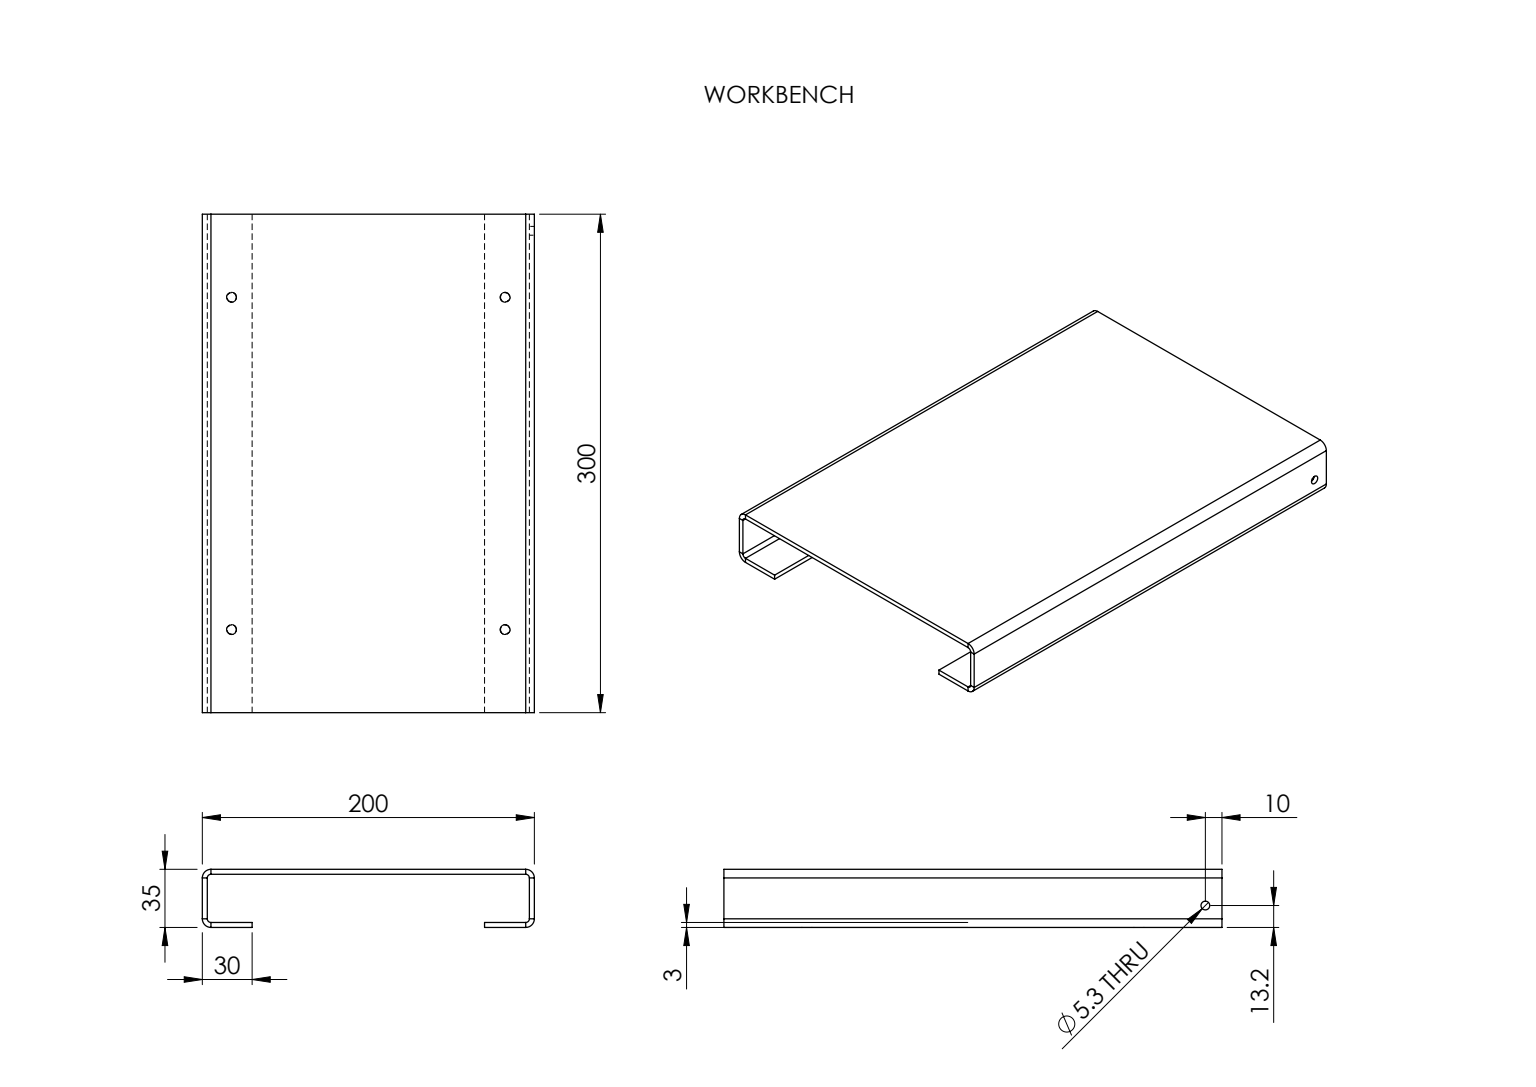
ISO-10303-21;
HEADER;
FILE_DESCRIPTION (('STEP AP214'),
    '1' );
FILE_NAME ('workbench.step',
    '2026-10-25T17:17:34',
    ( '' ),
    ( '' ),
    'SwSTEP 2.0',
    'SolidWorks 2026',
    '' );
FILE_SCHEMA (( 'AUTOMOTIVE_DESIGN' ));
ENDSEC;

DATA;
#2=CARTESIAN_POINT ( 'NONE',  ( 85.15643035625001289, -33.70312499938548711, 98.40857419181659793 ) ) ;
#3=CARTESIAN_POINT ( 'NONE',  ( 82.39999999999999147, -32.36250000000000426, -96.99999999999997158 ) ) ;
#5=CARTESIAN_POINT ( 'NONE',  ( 80.90000000000000568, -33.24374999877097281, -97.40192378864668399 ) ) ;
#8=ORIENTED_EDGE ( 'NONE', *, *, #12900, .F. ) ;
#13=ORIENTED_EDGE ( 'NONE', *, *, #6864, .F. ) ;
#14=VERTEX_POINT ( 'NONE', #6375 ) ;
#17=CARTESIAN_POINT ( 'NONE',  ( -85.40000000000000568, -32.23124999877096997, 98.26794919243111792 ) ) ;
#19=CARTESIAN_POINT ( 'NONE',  ( -79.77811200999887831, -35.00000000000000000, 100.8506536761481414 ) ) ;
#20=CARTESIAN_POINT ( 'NONE',  ( 82.40000000000000568, -30.00000000000000355, -103.0000000000000000 ) ) ;
#21=CARTESIAN_POINT ( 'NONE',  ( -81.02178482187500208, -34.45312499938548711, 97.61286128772489690 ) ) ;
#29=EDGE_LOOP ( 'NONE', ( #8971, #4412, #15076, #17801 ) ) ;
#30=CARTESIAN_POINT ( 'NONE',  ( -85.15643035624999868, -34.22812499938547859, -101.5914258081833879 ) ) ;
#33=CARTESIAN_POINT ( 'NONE',  ( 80.07894310789828296, -34.99999999999997868, -101.4973817956044400 ) ) ;
#38=ORIENTED_EDGE ( 'NONE', *, *, #10348, .F. ) ;
#39=CARTESIAN_POINT ( 'NONE',  ( -84.28136653320154892, -32.00000000000001421, 97.98546077809197641 ) ) ;
#41=CARTESIAN_POINT ( 'NONE',  ( -85.40000000000000568, -32.60624999877097707, 101.7320508075688679 ) ) ;
#42=CARTESIAN_POINT ( 'NONE',  ( 82.39999999999999147, -32.36250000000000426, 103.4641016151377499 ) ) ;
#43=CARTESIAN_POINT ( 'NONE',  ( -80.80636817121818183, -32.00000000000000000, -97.53037344451308854 ) ) ;
#46=CARTESIAN_POINT ( 'NONE',  ( 82.39999999999999147, -33.62812499938549138, 96.81714838363319586 ) ) ;
#48=CARTESIAN_POINT ( 'NONE',  ( 85.15643035625001289, -30.59062499938548285, -99.99999999999998579 ) ) ;
#50=( BOUNDED_CURVE ( )  B_SPLINE_CURVE ( 2, ( #14072, #3327, #4905, #3619, #6463, #18477, #9481, #10851, #12417 ),
 .UNSPECIFIED., .F., .F. ) 
 B_SPLINE_CURVE_WITH_KNOTS ( ( 3, 2, 2, 2, 3 ),
 ( 0.6041666666666666297, 0.6111111111111111605, 0.6250000000000000000, 0.6388888888888888395, 0.6458333333333332593 ),
 .UNSPECIFIED. ) 
 CURVE ( )  GEOMETRIC_REPRESENTATION_ITEM ( )  RATIONAL_B_SPLINE_CURVE ( ( 0.9330127018922192983, 0.9330127018922187432, 1.000000000000000000, 0.8660254037844387076, 1.000000000000000000, 0.8660254037844387076, 1.000000000000000000, 0.9330127018922198534, 0.9330127018922192983 ) ) 
 REPRESENTATION_ITEM ( '' )  );
#53=CARTESIAN_POINT ( 'NONE',  ( 83.77821517812500929, -34.26562499938548711, -97.61286128772489690 ) ) ;
#55=CYLINDRICAL_SURFACE ( 'NONE', #7872, 3.000000000000002665 ) ;
#57=( BOUNDED_CURVE ( )  B_SPLINE_CURVE ( 2, ( #14794, #2683, #1229, #10402, #2880, #14892, #1421, #4162, #17640 ),
 .UNSPECIFIED., .F., .F. ) 
 B_SPLINE_CURVE_WITH_KNOTS ( ( 3, 2, 2, 2, 3 ),
 ( 0.6458333333333333703, 0.6527777777777777901, 0.6666666666666666297, 0.6805555555555555802, 0.6875000000000000000 ),
 .UNSPECIFIED. ) 
 CURVE ( )  GEOMETRIC_REPRESENTATION_ITEM ( )  RATIONAL_B_SPLINE_CURVE ( ( 0.9330127018922192983, 0.9330127018922198534, 1.000000000000000000, 0.8660254037844387076, 1.000000000000000000, 0.8660254037844387076, 1.000000000000000000, 0.9330127018922194093, 0.9330127018922194093 ) ) 
 REPRESENTATION_ITEM ( '' )  );
#58=CARTESIAN_POINT ( 'NONE',  ( -85.40000000000000568, -30.03750000000000497, 98.26794919243111792 ) ) ;
#60=CARTESIAN_POINT ( 'NONE',  ( -80.90000000000000568, -32.85000000000000142, 97.40192378864668399 ) ) ;
#64=EDGE_CURVE ( 'NONE', #2579, #12229, #9687, .T. ) ;
#65=LINE ( 'NONE', #3169, #11720 ) ;
#68=CARTESIAN_POINT ( 'NONE',  ( -79.39999999999999147, -32.47500000000000142, 99.99999999999998579 ) ) ;
#69=CARTESIAN_POINT ( 'NONE',  ( 83.77821517812500929, -32.57812499938548711, 102.3871387122750889 ) ) ;
#72=CARTESIAN_POINT ( 'NONE',  ( 85.15643035625001289, -30.25312499938548783, -99.99999999999998579 ) ) ;
#74=CARTESIAN_POINT ( 'NONE',  ( -83.77821517812500929, -32.87812499938548427, 102.3871387122750889 ) ) ;
#75=CARTESIAN_POINT ( 'NONE',  ( -85.15643035624999868, -30.29062499938548925, -101.5914258081833879 ) ) ;
#76=ORIENTED_EDGE ( 'NONE', *, *, #18961, .F. ) ;
#77=CARTESIAN_POINT ( 'NONE',  ( 85.40000000000000568, -35.34374999877096712, 99.99999999999998579 ) ) ;
#79=CARTESIAN_POINT ( 'NONE',  ( -82.40000000000000568, -30.00000000000000355, -96.99999999999998579 ) ) ;
#80=VECTOR ( 'NONE', #9829, 1000.000000000000000 ) ;
#81=CARTESIAN_POINT ( 'NONE',  ( -99.99999999999998579, -5.200000000000000178, 150.0000000000000000 ) ) ;
#83=CARTESIAN_POINT ( 'NONE',  ( -83.77821517812500929, -31.07812499938548711, 102.3871387122750889 ) ) ;
#84=( BOUNDED_CURVE ( )  B_SPLINE_CURVE ( 2, ( #13183, #17688, #10354, #13091, #8980, #17790, #14840, #19061, #2929 ),
 .UNSPECIFIED., .F., .F. ) 
 B_SPLINE_CURVE_WITH_KNOTS ( ( 3, 2, 2, 2, 3 ),
 ( 0.7708333333333332593, 0.7777777777777777901, 0.7916666666666666297, 0.8055555555555555802, 0.8125000000000000000 ),
 .UNSPECIFIED. ) 
 CURVE ( )  GEOMETRIC_REPRESENTATION_ITEM ( )  RATIONAL_B_SPLINE_CURVE ( ( 0.9330127018922192983, 0.9330127018922187432, 1.000000000000000000, 0.8660254037844387076, 1.000000000000000000, 0.8660254037844387076, 1.000000000000000000, 0.9330127018922194093, 0.9330127018922194093 ) ) 
 REPRESENTATION_ITEM ( '' )  );
#85=CARTESIAN_POINT ( 'NONE',  ( 82.61711639273572416, -31.99999999999999289, 102.8399189874672857 ) ) ;
#87=CARTESIAN_POINT ( 'NONE',  ( -83.90000000000000568, -30.82500000000000284, -97.40192378864668399 ) ) ;
#90=CARTESIAN_POINT ( 'NONE',  ( -85.15643035625001289, -32.95312499938548711, -99.99999999999998579 ) ) ;
#91=CARTESIAN_POINT ( 'NONE',  ( -82.14831453747900980, -32.00000000000000711, -102.8584433575392438 ) ) ;
#97=CARTESIAN_POINT ( 'NONE',  ( 83.77821517812500929, -33.66562499938548569, 97.61286128772489690 ) ) ;
#98=CARTESIAN_POINT ( 'NONE',  ( 80.90000000000000568, -32.40000000000000568, -97.40192378864668399 ) ) ;
#99=AXIS2_PLACEMENT_3D ( 'NONE', #13083, #5582, #10259 ) ;
#102=CARTESIAN_POINT ( 'NONE',  ( 83.90000000000000568, -35.26874999877097139, -102.5980762113533018 ) ) ;
#110=ORIENTED_EDGE ( 'NONE', *, *, #1169, .T. ) ;
#113=CARTESIAN_POINT ( 'NONE',  ( -81.90908125319960220, -32.00000000000000711, 97.16185054498753004 ) ) ;
#116=CARTESIAN_POINT ( 'NONE',  ( -79.39999999999999147, -34.76250000000000284, 101.7320508075688537 ) ) ;
#118=CARTESIAN_POINT ( 'NONE',  ( 69.99999999999998579, -31.99999999999998579, 150.0000000000000000 ) ) ;
#120=CARTESIAN_POINT ( 'NONE',  ( -85.15643035624999868, -33.44062499938548427, 98.40857419181659793 ) ) ;
#124=( BOUNDED_SURFACE ( )  B_SPLINE_SURFACE ( 1, 2, ( 
 ( #72, #18045, #10508, #17940, #4551, #3080, #4656, #1713, #12454, #13815, #2197, #651, #7770, #5135, #16858, #3463, #457, #16755, #7864, #15189, #8158, #2001, #1806, #6406, #9522, #9323, #14107, #17050, #9225, #11080, #551, #3563, #9626, #9421, #3371, #6508, #18420, #5041, #15389, #15287, #4754, #4848, #1902, #10982, #8060, #13913, #2100, #4947, #3269, #18518, #15588, #14015, #6599, #13723, #10793, #6699, #18329, #3661, #12361, #10890, #7958, #744, #364, #6313, #18135, #12266, #16951, #15487, #12547, #18231, #10698, #16664, #18617, #11277, #3951, #5339, #19004, #9815, #8536, #840, #5526, #6893, #1218, #6984, #14302, #2574, #12935, #5624, #16064, #14392, #1117, #18907, #15777, #18717, #3852, #17245, #2386, #12643, #12749, #8348, #11474, #4052, #15878, #938, #17441, #15685, #4148, #5235, #6803, #12843, #2482, #11183, #8440, #8253, #14486, #9719, #10011, #18812, #2669, #7077, #2289, #11570, #11375, #17341, #5436, #9916, #1031, #14203, #8629, #15969, #13033, #17533, #10108, #14587, #17147 ),
 ( #3754, #18022, #5908, #5808, #8918, #14880, #1509, #17822, #17733, #13124, #13221, #4340, #48, #16450, #2963, #10487, #13318, #11665, #7554, #4636, #3060, #9022, #16165, #19193, #15075, #7362, #148, #11759, #19295, #10301, #13511, #17628, #2776, #6099, #10201, #10391, #7459, #13419, #1318, #4243, #8729, #19094, #16260, #4433, #2870, #12047, #8827, #14981, #14683, #6000, #1409, #7174, #11950, #14784, #1605, #17920, #10586, #16551, #4529, #3150, #9113, #11854, #16352, #5715, #7266, #7751, #9602, #1786, #6293, #530, #12435, #4925, #16736, #15366, #4730, #12527, #7646, #15169, #15268, #10870, #13706, #6483, #3544, #1982, #15468, #346, #18116, #1883, #2078, #8035, #1694, #6581, #13601, #18403, #11059, #13992, #12244, #18211, #10964, #7940, #10772, #12341, #631, #3346, #5023, #4831, #18500, #9306, #10675, #440, #16841, #16644, #3447, #13891, #9500, #7842, #3640, #3246, #16934, #5119, #13797, #6385, #18305, #17030, #9402, #242, #6201, #12148, #9204, #17221, #8136, #18982, #17420, #4123, #2271 ) ),
 .UNSPECIFIED., .F., .F., .F. ) 
 B_SPLINE_SURFACE_WITH_KNOTS ( ( 2, 2 ),
 ( 3, 2, 2, 2, 2, 2, 2, 2, 2, 2, 2, 2, 2, 2, 2, 2, 2, 2, 2, 2, 2, 2, 2, 2, 2, 2, 2, 2, 2, 2, 2, 2, 2, 2, 2, 2, 2, 2, 2, 2, 2, 2, 2, 2, 2, 2, 2, 2, 2, 2, 2, 2, 2, 2, 2, 2, 2, 2, 2, 2, 2, 2, 2, 2, 2, 2, 2, 3 ),
 ( 0.000000000000000000, 1.000000000000000000 ),
 ( 0.000000000000000000, 0.01388888888888888812, 0.02777777777777777624, 0.04166666666666666435, 0.05555555555555555247, 0.06944444444444444753, 0.08333333333333332871, 0.09722222222222222376, 0.1111111111111111049, 0.1250000000000000000, 0.1388888888888888951, 0.1527777777777777901, 0.1666666666666666574, 0.1805555555555555525, 0.1944444444444444475, 0.2083333333333333426, 0.2222222222222222099, 0.2361111111111111049, 0.2500000000000000000, 0.2638888888888888951, 0.2777777777777777901, 0.2916666666666666852, 0.3055555555555555802, 0.3194444444444444198, 0.3333333333333333148, 0.3472222222222222099, 0.3611111111111111049, 0.3750000000000000000, 0.3888888888888888951, 0.4027777777777777901, 0.4166666666666666852, 0.4305555555555555802, 0.4444444444444444198, 0.4583333333333333148, 0.4722222222222222099, 0.4861111111111111049, 0.5000000000000000000, 0.5138888888888888395, 0.5277777777777777901, 0.5416666666666666297, 0.5555555555555555802, 0.5694444444444444198, 0.5833333333333333703, 0.5972222222222222099, 0.6111111111111111605, 0.6250000000000000000, 0.6388888888888888395, 0.6527777777777777901, 0.6666666666666666297, 0.6805555555555555802, 0.6944444444444444198, 0.7083333333333333703, 0.7222222222222222099, 0.7361111111111111605, 0.7500000000000000000, 0.7638888888888888395, 0.7777777777777777901, 0.7916666666666666297, 0.8055555555555555802, 0.8194444444444444198, 0.8333333333333333703, 0.8472222222222222099, 0.8611111111111111605, 0.8750000000000000000, 0.8888888888888888395, 0.9027777777777777901, 0.9166666666666666297, 0.9258785565094813652 ),
 .UNSPECIFIED. ) 
 GEOMETRIC_REPRESENTATION_ITEM ( )  RATIONAL_B_SPLINE_SURFACE ( (
 ( 1.000000000000000000, 0.8660254037844387076, 1.000000000000000000, 0.8660254037844387076, 1.000000000000000000, 0.8660254037844387076, 1.000000000000000000, 0.8660254037844387076, 1.000000000000000000, 0.8660254037844387076, 1.000000000000000000, 0.8660254037844387076, 1.000000000000000000, 0.8660254037844387076, 1.000000000000000000, 0.8660254037844387076, 1.000000000000000000, 0.8660254037844387076, 1.000000000000000000, 0.8660254037844387076, 1.000000000000000000, 0.8660254037844387076, 1.000000000000000000, 0.8660254037844387076, 1.000000000000000000, 0.8660254037844387076, 1.000000000000000000, 0.8660254037844387076, 1.000000000000000000, 0.8660254037844387076, 1.000000000000000000, 0.8660254037844387076, 1.000000000000000000, 0.8660254037844387076, 1.000000000000000000, 0.8660254037844387076, 1.000000000000000000, 0.8660254037844387076, 1.000000000000000000, 0.8660254037844387076, 1.000000000000000000, 0.8660254037844387076, 1.000000000000000000, 0.8660254037844387076, 1.000000000000000000, 0.8660254037844387076, 1.000000000000000000, 0.8660254037844387076, 1.000000000000000000, 0.8660254037844387076, 1.000000000000000000, 0.8660254037844387076, 1.000000000000000000, 0.8660254037844387076, 1.000000000000000000, 0.8660254037844387076, 1.000000000000000000, 0.8660254037844387076, 1.000000000000000000, 0.8660254037844387076, 1.000000000000000000, 0.8660254037844387076, 1.000000000000000000, 0.8660254037844387076, 1.000000000000000000, 0.8660254037844387076, 1.000000000000000000, 0.8660254037844387076, 1.000000000000000000, 0.8660254037844387076, 1.000000000000000000, 0.8660254037844387076, 1.000000000000000000, 0.8660254037844387076, 1.000000000000000000, 0.8660254037844387076, 1.000000000000000000, 0.8660254037844387076, 1.000000000000000000, 0.8660254037844387076, 1.000000000000000000, 0.8660254037844387076, 1.000000000000000000, 0.8660254037844387076, 1.000000000000000000, 0.8660254037844387076, 1.000000000000000000, 0.8660254037844387076, 1.000000000000000000, 0.8660254037844387076, 1.000000000000000000, 0.8660254037844387076, 1.000000000000000000, 0.8660254037844387076, 1.000000000000000000, 0.8660254037844387076, 1.000000000000000000, 0.8660254037844387076, 1.000000000000000000, 0.8660254037844387076, 1.000000000000000000, 0.8660254037844387076, 1.000000000000000000, 0.8660254037844387076, 1.000000000000000000, 0.8660254037844387076, 1.000000000000000000, 0.8660254037844387076, 1.000000000000000000, 0.8660254037844387076, 1.000000000000000000, 0.8660254037844387076, 1.000000000000000000, 0.8660254037844387076, 1.000000000000000000, 0.8660254037844387076, 1.000000000000000000, 0.8660254037844387076, 1.000000000000000000, 0.8660254037844387076, 1.000000000000000000, 0.8660254037844387076, 1.000000000000000000, 0.8660254037844387076, 1.000000000000000000, 0.8660254037844387076, 1.000000000000000000, 0.8660254037844387076, 1.000000000000000000, 0.8660254037844387076, 1.000000000000000000, 0.8660254037844387076, 1.000000000000000000, 0.9111405360107203144, 0.9401542295229963209),
 ( 1.000000000000000000, 0.8660254037844387076, 1.000000000000000000, 0.8660254037844387076, 1.000000000000000000, 0.8660254037844387076, 1.000000000000000000, 0.8660254037844387076, 1.000000000000000000, 0.8660254037844387076, 1.000000000000000000, 0.8660254037844387076, 1.000000000000000000, 0.8660254037844387076, 1.000000000000000000, 0.8660254037844387076, 1.000000000000000000, 0.8660254037844387076, 1.000000000000000000, 0.8660254037844387076, 1.000000000000000000, 0.8660254037844387076, 1.000000000000000000, 0.8660254037844387076, 1.000000000000000000, 0.8660254037844387076, 1.000000000000000000, 0.8660254037844387076, 1.000000000000000000, 0.8660254037844387076, 1.000000000000000000, 0.8660254037844387076, 1.000000000000000000, 0.8660254037844387076, 1.000000000000000000, 0.8660254037844387076, 1.000000000000000000, 0.8660254037844387076, 1.000000000000000000, 0.8660254037844387076, 1.000000000000000000, 0.8660254037844387076, 1.000000000000000000, 0.8660254037844387076, 1.000000000000000000, 0.8660254037844387076, 1.000000000000000000, 0.8660254037844387076, 1.000000000000000000, 0.8660254037844387076, 1.000000000000000000, 0.8660254037844387076, 1.000000000000000000, 0.8660254037844387076, 1.000000000000000000, 0.8660254037844387076, 1.000000000000000000, 0.8660254037844387076, 1.000000000000000000, 0.8660254037844387076, 1.000000000000000000, 0.8660254037844387076, 1.000000000000000000, 0.8660254037844387076, 1.000000000000000000, 0.8660254037844387076, 1.000000000000000000, 0.8660254037844387076, 1.000000000000000000, 0.8660254037844387076, 1.000000000000000000, 0.8660254037844387076, 1.000000000000000000, 0.8660254037844387076, 1.000000000000000000, 0.8660254037844387076, 1.000000000000000000, 0.8660254037844387076, 1.000000000000000000, 0.8660254037844387076, 1.000000000000000000, 0.8660254037844387076, 1.000000000000000000, 0.8660254037844387076, 1.000000000000000000, 0.8660254037844387076, 1.000000000000000000, 0.8660254037844387076, 1.000000000000000000, 0.8660254037844387076, 1.000000000000000000, 0.8660254037844387076, 1.000000000000000000, 0.8660254037844387076, 1.000000000000000000, 0.8660254037844387076, 1.000000000000000000, 0.8660254037844387076, 1.000000000000000000, 0.8660254037844387076, 1.000000000000000000, 0.8660254037844387076, 1.000000000000000000, 0.8660254037844387076, 1.000000000000000000, 0.8660254037844387076, 1.000000000000000000, 0.8660254037844387076, 1.000000000000000000, 0.8660254037844387076, 1.000000000000000000, 0.8660254037844387076, 1.000000000000000000, 0.8660254037844387076, 1.000000000000000000, 0.8660254037844387076, 1.000000000000000000, 0.8660254037844387076, 1.000000000000000000, 0.8660254037844387076, 1.000000000000000000, 0.8660254037844387076, 1.000000000000000000, 0.8660254037844387076, 1.000000000000000000, 0.8660254037844387076, 1.000000000000000000, 0.8660254037844387076, 1.000000000000000000, 0.8660254037844387076, 1.000000000000000000, 0.8660254037844387076, 1.000000000000000000, 0.9111405360107203144, 0.9401542295229963209) ) ) 
 REPRESENTATION_ITEM ( '' )  SURFACE ( )  );
#126=CARTESIAN_POINT ( 'NONE',  ( -80.90000000000000568, -33.45000000000000284, 102.5980762113533018 ) ) ;
#127=CARTESIAN_POINT ( 'NONE',  ( -79.39999999999999147, -34.70624999877097139, -98.26794919243113213 ) ) ;
#131=CARTESIAN_POINT ( 'NONE',  ( -79.64356964374999848, -33.51562499938548711, -99.99999999999998579 ) ) ;
#134=CARTESIAN_POINT ( 'NONE',  ( 81.96801452314025482, -35.00000000000000000, -102.7281823352556671 ) ) ;
#139=EDGE_LOOP ( 'NONE', ( #12823, #17187, #7892, #9526 ) ) ;
#142=CARTESIAN_POINT ( 'NONE',  ( -79.39999999999999147, -32.90624999877096712, 101.7320508075688537 ) ) ;
#143=CARTESIAN_POINT ( 'NONE',  ( 80.90000000000000568, -31.50000000000000000, 102.5980762113533018 ) ) ;
#146=CARTESIAN_POINT ( 'NONE',  ( 83.90000000000000568, -32.11874999877097281, 97.40192378864668399 ) ) ;
#147=CARTESIAN_POINT ( 'NONE',  ( 79.39999999999999147, -33.33749999999999858, -98.26794919243110371 ) ) ;
#148=CARTESIAN_POINT ( 'NONE',  ( 83.77821517812500929, -31.11562499938548498, -97.61286128772489690 ) ) ;
#151=CARTESIAN_POINT ( 'NONE',  ( 82.40000000000000568, -34.10624999877096997, 102.9999999999999858 ) ) ;
#152=CARTESIAN_POINT ( 'NONE',  ( 79.64356964375001269, -34.37812499938548427, -98.40857419181659793 ) ) ;
#154=CARTESIAN_POINT ( 'NONE',  ( -81.59615242270662350, -34.76115380933863719, 103.0000000000000000 ) ) ;
#156=CARTESIAN_POINT ( 'NONE',  ( -79.39999999999999147, -31.08750000000000213, 98.26794919243110371 ) ) ;
#157=ORIENTED_EDGE ( 'NONE', *, *, #9586, .F. ) ;
#163=DIRECTION ( 'NONE',  ( 1.000000000000000000, 0.000000000000000000, 0.000000000000000000 ) ) ;
#164=CARTESIAN_POINT ( 'NONE',  ( -82.40000000000000568, -32.30624999877097281, 97.00000000000000000 ) ) ;
#166=CARTESIAN_POINT ( 'NONE',  ( 81.02178482187500208, -34.90312499938548285, 102.3871387122750889 ) ) ;
#169=CARTESIAN_POINT ( 'NONE',  ( -83.77821517812500929, -32.42812499938548854, 102.3871387122750889 ) ) ;
#170=CARTESIAN_POINT ( 'NONE',  ( -81.02178482187500208, -30.55312499938548854, -97.61286128772489690 ) ) ;
#171=( BOUNDED_CURVE ( )  B_SPLINE_CURVE ( 2, ( #17183, #11218, #2322, #15621, #3787, #16002, #5563, #9753, #17473 ),
 .UNSPECIFIED., .F., .F. ) 
 B_SPLINE_CURVE_WITH_KNOTS ( ( 3, 2, 2, 2, 3 ),
 ( 0.7291666666666668517, 0.7361111111111111605, 0.7500000000000000000, 0.7638888888888888395, 0.7708333333333332593 ),
 .UNSPECIFIED. ) 
 CURVE ( )  GEOMETRIC_REPRESENTATION_ITEM ( )  RATIONAL_B_SPLINE_CURVE ( ( 0.9330127018922194093, 0.9330127018922209636, 1.000000000000000000, 0.8660254037844387076, 1.000000000000000000, 0.8660254037844387076, 1.000000000000000000, 0.9330127018922198534, 0.9330127018922192983 ) ) 
 REPRESENTATION_ITEM ( '' )  );
#173=CARTESIAN_POINT ( 'NONE',  ( 83.77821517812500929, -31.07812499938548711, 97.61286128772489690 ) ) ;
#174=CARTESIAN_POINT ( 'NONE',  ( -94.79999999999999716, -35.00000000000000000, 150.0000000000000000 ) ) ;
#176=VECTOR ( 'NONE', #9077, 1000.000000000000000 ) ;
#179=CARTESIAN_POINT ( 'NONE',  ( -81.02178482187500208, -31.30312499938548498, 97.61286128772489690 ) ) ;
#181=ORIENTED_EDGE ( 'NONE', *, *, #9607, .T. ) ;
#182=CARTESIAN_POINT ( 'NONE',  ( -79.39999999999999147, -32.06250000000000000, -98.26794919243113213 ) ) ;
#184=DIRECTION ( 'NONE',  ( 1.000000000000000000, -2.001604010742470847E-15, 0.000000000000000000 ) ) ;
#185=CARTESIAN_POINT ( 'NONE',  ( -81.02178482187500208, -32.35312499938548569, -97.61286128772489690 ) ) ;
#191=CARTESIAN_POINT ( 'NONE',  ( -85.15643035625001289, -34.60312499938548569, -98.40857419181659793 ) ) ;
#192=CARTESIAN_POINT ( 'NONE',  ( 85.15643035625001289, -34.22812499938548569, 101.5914258081833879 ) ) ;
#194=CIRCLE ( 'NONE', #8915, 2.199999999999993516 ) ;
#196=CARTESIAN_POINT ( 'NONE',  ( 82.39999999999999147, -33.43124999877097281, -103.4641016151377499 ) ) ;
#208=ORIENTED_EDGE ( 'NONE', *, *, #11264, .T. ) ;
#211=CARTESIAN_POINT ( 'NONE',  ( -85.15643035625001289, -33.40312499938548285, 99.99999999999998579 ) ) ;
#218=CARTESIAN_POINT ( 'NONE',  ( 82.39999999999999147, -34.83749999999999858, -103.0000000000000000 ) ) ;
#220=CARTESIAN_POINT ( 'NONE',  ( -82.40000000000000568, -30.00000000000000355, -103.0000000000000000 ) ) ;
#224=CARTESIAN_POINT ( 'NONE',  ( -85.15643035625001289, -33.29062499938547859, -99.99999999999998579 ) ) ;
#231=ORIENTED_EDGE ( 'NONE', *, *, #3636, .T. ) ;
#232=CARTESIAN_POINT ( 'NONE',  ( -83.74167325096719594, -31.99999999999997868, 102.4658751321106962 ) ) ;
#235=CARTESIAN_POINT ( 'NONE',  ( -83.90000000000000568, -30.91874999877096997, 97.40192378864668399 ) ) ;
#236=CARTESIAN_POINT ( 'NONE',  ( 82.39999999999999147, -32.58750000000000568, 96.53589838486223584 ) ) ;
#237=CARTESIAN_POINT ( 'NONE',  ( -80.42036527867321638, -32.00000000000000000, -97.80162405160960759 ) ) ;
#241=CARTESIAN_POINT ( 'NONE',  ( 81.59615242270662350, -33.46740381056766722, -102.9999999999999716 ) ) ;
#242=CARTESIAN_POINT ( 'NONE',  ( 79.64356964375001269, -34.82812499938548711, -98.40857419181659793 ) ) ;
#246=CARTESIAN_POINT ( 'NONE',  ( 85.15643035624999868, -33.77812499938548285, -98.40857419181659793 ) ) ;
#247=VECTOR ( 'NONE', #7483, 1000.000000000000000 ) ;
#249=CARTESIAN_POINT ( 'NONE',  ( 94.79999999999995453, -29.80000000000000071, 150.0000000000000000 ) ) ;
#252=CARTESIAN_POINT ( 'NONE',  ( -80.90000000000000568, -30.75000000000000355, 102.5980762113533018 ) ) ;
#258=CARTESIAN_POINT ( 'NONE',  ( 79.64356964375001269, -30.85312499938548569, 98.40857419181659793 ) ) ;
#263=CARTESIAN_POINT ( 'NONE',  ( 85.12124608221321864, -31.99999999999999289, 100.4735569575797030 ) ) ;
#264=CARTESIAN_POINT ( 'NONE',  ( 83.77821517812500929, -33.92812499938548854, 102.3871387122750889 ) ) ;
#268=CARTESIAN_POINT ( 'NONE',  ( -84.74067385206558356, -32.00000000000000000, -101.4666071953143529 ) ) ;
#269=CARTESIAN_POINT ( 'NONE',  ( -79.64356964374999848, -34.52812499938548285, -99.99999999999998579 ) ) ;
#271=ORIENTED_EDGE ( 'NONE', *, *, #3421, .F. ) ;
#272=CARTESIAN_POINT ( 'NONE',  ( 79.64356964375001269, -31.41562499938548569, 98.40857419181659793 ) ) ;
#273=CARTESIAN_POINT ( 'NONE',  ( 96.99999999999998579, 4.758098676964956264E-15, -150.0000000000000000 ) ) ;
#277=CARTESIAN_POINT ( 'NONE',  ( -82.39999999999999147, -31.49062499938548854, 103.1828516163667899 ) ) ;
#280=CARTESIAN_POINT ( 'NONE',  ( -85.40000000000000568, -30.86250000000000071, -98.26794919243111792 ) ) ;
#281=CARTESIAN_POINT ( 'NONE',  ( 85.40000000000000568, -34.46249999999999858, -101.7320508075688679 ) ) ;
#282=DIRECTION ( 'NONE',  ( -1.000000000000000000, 0.000000000000000000, 0.000000000000000000 ) ) ;
#283=CARTESIAN_POINT ( 'NONE',  ( -85.15643035624999868, -33.81562499938549138, -98.40857419181659793 ) ) ;
#291=CARTESIAN_POINT ( 'NONE',  ( -79.64356964374998427, -34.00312499938548427, -98.40857419181659793 ) ) ;
#292=CARTESIAN_POINT ( 'NONE',  ( 82.39999999999999147, -34.30312499938548143, 103.1828516163667899 ) ) ;
#293=CARTESIAN_POINT ( 'NONE',  ( 79.39999999999999147, -34.31250000000000000, 98.26794919243113213 ) ) ;
#294=( BOUNDED_CURVE ( )  B_SPLINE_CURVE ( 2, ( #4333, #5428, #17722, #10192, #1107, #14385, #5519, #1310, #7258 ),
 .UNSPECIFIED., .F., .F. ) 
 B_SPLINE_CURVE_WITH_KNOTS ( ( 3, 2, 2, 2, 3 ),
 ( 0.3125000000000001665, 0.3194444444444444198, 0.3333333333333333148, 0.3472222222222222099, 0.3541666666666666297 ),
 .UNSPECIFIED. ) 
 CURVE ( )  GEOMETRIC_REPRESENTATION_ITEM ( )  RATIONAL_B_SPLINE_CURVE ( ( 0.9330127018922194093, 0.9330127018922209636, 1.000000000000000000, 0.8660254037844387076, 1.000000000000000000, 0.8660254037844387076, 1.000000000000000000, 0.9330127018922196314, 0.9330127018922194093 ) ) 
 REPRESENTATION_ITEM ( '' )  );
#295=CARTESIAN_POINT ( 'NONE',  ( 110.9999999999999574, -21.80000000000003268, -142.6499999999999773 ) ) ;
#296=CARTESIAN_POINT ( 'NONE',  ( 82.39999999999999147, -34.55624999877096570, -96.53589838486223584 ) ) ;
#311=CARTESIAN_POINT ( 'NONE',  ( -99.99999999999998579, -29.80000000000000426, 150.0000000000000000 ) ) ;
#315=EDGE_CURVE ( 'NONE', #15577, #16231, #9273, .T. ) ;
#320=CARTESIAN_POINT ( 'NONE',  ( 82.40000000000000568, -34.61250000000001137, -97.00000000000000000 ) ) ;
#321=CARTESIAN_POINT ( 'NONE',  ( -79.39999999999999147, -33.37500000000000000, 99.99999999999998579 ) ) ;
#323=EDGE_CURVE ( 'NONE', #14868, #14858, #1084, .T. ) ;
#328=CARTESIAN_POINT ( 'NONE',  ( -85.15643035624999868, -32.35312499938549280, -98.40857419181659793 ) ) ;
#337=CARTESIAN_POINT ( 'NONE',  ( 79.39999999999999147, -34.63124999877096855, 101.7320508075688963 ) ) ;
#339=CARTESIAN_POINT ( 'NONE',  ( 82.39999999999999147, -34.97812499938547859, -103.1828516163667899 ) ) ;
#340=CARTESIAN_POINT ( 'NONE',  ( -79.39999999999999147, -31.03124999877097068, 98.26794919243110371 ) ) ;
#341=CARTESIAN_POINT ( 'NONE',  ( 85.40000000000000568, -32.25000000000000000, 99.99999999999998579 ) ) ;
#342=CARTESIAN_POINT ( 'NONE',  ( -83.52979456739218733, -32.00000000000002132, -97.41965524898077433 ) ) ;
#344=CARTESIAN_POINT ( 'NONE',  ( 83.77821517812500929, -32.42812499938548854, -102.3871387122750889 ) ) ;
#345=CARTESIAN_POINT ( 'NONE',  ( 82.40000000000000568, -30.00000000000000355, 99.99999999999998579 ) ) ;
#346=CARTESIAN_POINT ( 'NONE',  ( 85.15643035624999868, -33.32812499938548001, -98.40857419181659793 ) ) ;
#350=CARTESIAN_POINT ( 'NONE',  ( -83.20384757729335945, -34.14240381056767148, 96.99999999999998579 ) ) ;
#351=CARTESIAN_POINT ( 'NONE',  ( -85.40000000000000568, -34.08749999999999858, 98.26794919243111792 ) ) ;
#352=DIRECTION ( 'NONE',  ( 0.000000000000000000, -1.000000000000000000, 0.000000000000000000 ) ) ;
#355=CARTESIAN_POINT ( 'NONE',  ( -85.15643035624999868, -34.60312499938548569, 101.5914258081833879 ) ) ;
#359=CARTESIAN_POINT ( 'NONE',  ( 83.77821517812500929, -31.11562499938548498, 102.3871387122750889 ) ) ;
#363=CARTESIAN_POINT ( 'NONE',  ( 79.64356964374999848, -30.81562499938548427, 99.99999999999998579 ) ) ;
#364=CARTESIAN_POINT ( 'NONE',  ( 83.77821517812500929, -32.57812499938548711, -97.61286128772489690 ) ) ;
#366=CARTESIAN_POINT ( 'NONE',  ( -84.67508262029694777, -32.00000000000000711, -98.43364869553373353 ) ) ;
#367=CARTESIAN_POINT ( 'NONE',  ( -82.39999999999999147, -33.74062499938548854, -96.81714838363319586 ) ) ;
#369=CARTESIAN_POINT ( 'NONE',  ( 80.90000000000000568, -34.59374999877096712, 102.5980762113533018 ) ) ;
#372=CARTESIAN_POINT ( 'NONE',  ( -83.77821517812500929, -34.37812499938548427, 97.61286128772489690 ) ) ;
#375=CARTESIAN_POINT ( 'NONE',  ( -83.90000000000000568, -30.52500000000000213, -102.5980762113533018 ) ) ;
#376=CARTESIAN_POINT ( 'NONE',  ( 83.04276107155152431, -34.99999999999999289, 102.9375709370400642 ) ) ;
#377=CARTESIAN_POINT ( 'NONE',  ( 80.08630547029493130, -32.02340763552834346, -102.1282894555899361 ) ) ;
#383=LINE ( 'NONE', #15609, #4157 ) ;
#384=CARTESIAN_POINT ( 'NONE',  ( 79.64356964374998427, -32.57812499938548711, 101.5914258081833879 ) ) ;
#387=CARTESIAN_POINT ( 'NONE',  ( 83.90000000000000568, -34.51874999877097139, -97.40192378864668399 ) ) ;
#388=CYLINDRICAL_SURFACE ( 'NONE', #13636, 3.000000000000002665 ) ;
#391=ORIENTED_EDGE ( 'NONE', *, *, #17376, .F. ) ;
#395=CARTESIAN_POINT ( 'NONE',  ( -81.59615242270662350, -33.01740381056767148, -96.99999999999998579 ) ) ;
#396=ORIENTED_EDGE ( 'NONE', *, *, #404, .T. ) ;
#397=ORIENTED_EDGE ( 'NONE', *, *, #4624, .T. ) ;
#399=CARTESIAN_POINT ( 'NONE',  ( -81.59615242270665192, -33.86115380933864571, -97.00000000000000000 ) ) ;
#402=CARTESIAN_POINT ( 'NONE',  ( 85.15643035625001289, -32.09062499938548996, 101.5914258081833879 ) ) ;
#403=CARTESIAN_POINT ( 'NONE',  ( -80.90000000000000568, -32.79374999877096997, -102.5980762113533018 ) ) ;
#404=EDGE_CURVE ( 'NONE', #11560, #13270, #807, .T. ) ;
#406=SHAPE_REPRESENTATION ( 'workbench', ( #10540 ), #11151 ) ;
#411=CARTESIAN_POINT ( 'NONE',  ( 85.10336890118310293, -34.99999999999999289, -100.9939266215710347 ) ) ;
#413=EDGE_CURVE ( 'NONE', #18033, #12559, #12529, .T. ) ;
#419=CARTESIAN_POINT ( 'NONE',  ( -82.39999999999999147, -33.85312499938547859, -103.1828516163667899 ) ) ;
#421=AXIS2_PLACEMENT_3D ( 'NONE', #13678, #16422, #3033 ) ;
#422=VERTEX_POINT ( 'NONE', #7616 ) ;
#423=AXIS2_PLACEMENT_3D ( 'NONE', #249, #13325, #17925 ) ;
#427=ORIENTED_EDGE ( 'NONE', *, *, #13335, .T. ) ;
#428=CARTESIAN_POINT ( 'NONE',  ( -82.40000000000000568, -30.00000000000000355, 99.99999999999998579 ) ) ;
#429=ORIENTED_EDGE ( 'NONE', *, *, #4800, .F. ) ;
#430=EDGE_CURVE ( 'NONE', #19181, #5168, #15901, .T. ) ;
#431=ORIENTED_EDGE ( 'NONE', *, *, #17842, .F. ) ;
#433=CARTESIAN_POINT ( 'NONE',  ( 82.39999999999999147, -30.78750000000000497, -103.4641016151377499 ) ) ;
#435=CARTESIAN_POINT ( 'NONE',  ( -79.39999999999999147, -34.21874999877096712, 99.99999999999998579 ) ) ;
#436=CARTESIAN_POINT ( 'NONE',  ( -85.40000000000000568, -32.15624999877096712, -98.26794919243111792 ) ) ;
#437=AXIS2_PLACEMENT_3D ( 'NONE', #16344, #19283, #7543 ) ;
#438=LINE ( 'NONE', #9597, #5397 ) ;
#439=CARTESIAN_POINT ( 'NONE',  ( 81.02178482187500208, -34.00312499938548427, -97.61286128772489690 ) ) ;
#440=CARTESIAN_POINT ( 'NONE',  ( 85.15643035624999868, -34.22812499938547859, -98.40857419181659793 ) ) ;
#443=CARTESIAN_POINT ( 'NONE',  ( -83.90000000000000568, -33.97500000000000853, 102.5980762113533018 ) ) ;
#448=CARTESIAN_POINT ( 'NONE',  ( -85.40000000000000568, -31.80000000000000071, 99.99999999999998579 ) ) ;
#449=EDGE_LOOP ( 'NONE', ( #736, #12388, #396, #15662 ) ) ;
#452=DIRECTION ( 'NONE',  ( 0.000000000000000000, 1.000000000000000000, 0.000000000000000000 ) ) ;
#453=CARTESIAN_POINT ( 'NONE',  ( 84.74067385206575409, -31.99999999999999289, -98.53339280468588868 ) ) ;
#455=CARTESIAN_POINT ( 'NONE',  ( -82.39999999999999147, -32.16562499938548569, -103.1828516163667899 ) ) ;
#456=CARTESIAN_POINT ( 'NONE',  ( 82.39999999999999147, -35.09062499938548285, 96.81714838363319586 ) ) ;
#457=CARTESIAN_POINT ( 'NONE',  ( 81.02178482187500208, -30.85312499938548569, -97.61286128772489690 ) ) ;
#460=CARTESIAN_POINT ( 'NONE',  ( -84.28136653320154892, -32.00000000000001421, 97.98546077809197641 ) ) ;
#461=CARTESIAN_POINT ( 'NONE',  ( -79.64356964374999848, -33.17812499938548854, -99.99999999999998579 ) ) ;
#463=CARTESIAN_POINT ( 'NONE',  ( 85.15643035624999868, -33.81562499938549138, 98.40857419181659793 ) ) ;
#466=CARTESIAN_POINT ( 'NONE',  ( -83.77821517812500929, -35.12812499938548427, 102.3871387122750889 ) ) ;
#468=ORIENTED_EDGE ( 'NONE', *, *, #17120, .F. ) ;
#469=CARTESIAN_POINT ( 'NONE',  ( -85.40000000000000568, -30.90000000000000213, -99.99999999999998579 ) ) ;
#470=CARTESIAN_POINT ( 'NONE',  ( 82.65333140691207348, -34.99995246259152992, 102.9892844631211943 ) ) ;
#472=DIRECTION ( 'NONE',  ( 0.000000000000000000, -1.000000000000000000, 0.000000000000000000 ) ) ;
#478=CARTESIAN_POINT ( 'NONE',  ( 83.90000000000000568, -34.57500000000000284, -97.40192378864668399 ) ) ;
#479=CARTESIAN_POINT ( 'NONE',  ( 79.64356964374999848, -34.86562499938548143, 99.99999999999998579 ) ) ;
#480=CARTESIAN_POINT ( 'NONE',  ( 80.90000000000000568, -34.35000000000000853, 97.40192378864668399 ) ) ;
#481=CARTESIAN_POINT ( 'NONE',  ( -83.20384757729337366, -34.35134618820330843, 103.0000000000000000 ) ) ;
#482=CARTESIAN_POINT ( 'NONE',  ( 85.15643035624999868, -31.11562499938548854, -101.5914258081833879 ) ) ;
#483=DIRECTION ( 'NONE',  ( 0.000000000000000000, -1.000000000000000000, 0.000000000000000000 ) ) ;
#490=ORIENTED_EDGE ( 'NONE', *, *, #9846, .F. ) ;
#493=CARTESIAN_POINT ( 'NONE',  ( -80.90000000000000568, -34.64999999999999858, 97.40192378864668399 ) ) ;
#494=ORIENTED_EDGE ( 'NONE', *, *, #11033, .F. ) ;
#496=EDGE_CURVE ( 'NONE', #14858, #13499, #17905, .T. ) ;
#497=CARTESIAN_POINT ( 'NONE',  ( -79.39999999999999147, -34.63124999877096855, -101.7320508075688821 ) ) ;
#507=ORIENTED_EDGE ( 'NONE', *, *, #14382, .T. ) ;
#516=EDGE_CURVE ( 'NONE', #5045, #540, #9364, .T. ) ;
#518=VERTEX_POINT ( 'NONE', #596 ) ;
#520=CARTESIAN_POINT ( 'NONE',  ( 82.39999999999999147, -31.46250000000000568, -96.53589838486223584 ) ) ;
#522=CARTESIAN_POINT ( 'NONE',  ( -79.39999999999999147, -34.70624999877097139, 101.7320508075688537 ) ) ;
#526=CARTESIAN_POINT ( 'NONE',  ( 85.15643035625001289, -33.40312499938548285, -99.99999999999998579 ) ) ;
#527=CARTESIAN_POINT ( 'NONE',  ( -83.77821517812500929, -33.81562499938548427, 97.61286128772489690 ) ) ;
#528=EDGE_CURVE ( 'NONE', #3019, #11864, #4432, .T. ) ;
#530=CARTESIAN_POINT ( 'NONE',  ( 82.39999999999999147, -32.72812499938548569, -103.1828516163667899 ) ) ;
#533=( LENGTH_UNIT ( ) NAMED_UNIT ( * ) SI_UNIT ( .MILLI., .METRE. ) );
#534=CARTESIAN_POINT ( 'NONE',  ( 85.40000000000000568, -33.58124999877097139, -98.26794919243111792 ) ) ;
#538=CARTESIAN_POINT ( 'NONE',  ( -85.40000000000000568, -33.18750000000000000, 98.26794919243111792 ) ) ;
#540=VERTEX_POINT ( 'NONE', #17612 ) ;
#543=CARTESIAN_POINT ( 'NONE',  ( 81.02178482187500208, -31.64062499938548356, 102.3871387122750889 ) ) ;
#547=AXIS2_PLACEMENT_3D ( 'NONE', #14828, #1559, #10535 ) ;
#548=CARTESIAN_POINT ( 'NONE',  ( -82.39999999999999147, -32.39062499938548711, -96.81714838363319586 ) ) ;
#549=CARTESIAN_POINT ( 'NONE',  ( 85.15643035624999868, -33.81562499938549138, 98.40857419181659793 ) ) ;
#551=CARTESIAN_POINT ( 'NONE',  ( 79.64356964374999848, -31.37812499938548427, -99.99999999999998579 ) ) ;
#553=CARTESIAN_POINT ( 'NONE',  ( -82.39999999999999147, -34.41562499938548569, 96.81714838363319586 ) ) ;
#554=CARTESIAN_POINT ( 'NONE',  ( -83.77821517812500929, -33.77812499938548285, -97.61286128772489690 ) ) ;
#557=CARTESIAN_POINT ( 'NONE',  ( 79.64356964374999848, -32.27812499938548996, 99.99999999999998579 ) ) ;
#560=CARTESIAN_POINT ( 'NONE',  ( -81.02178482187500208, -33.25312499938548427, 102.3871387122750889 ) ) ;
#561=( BOUNDED_CURVE ( )  B_SPLINE_CURVE ( 2, ( #320, #6075, #16525, #7722, #13773, #6361, #4605, #12216, #218 ),
 .UNSPECIFIED., .F., .F. ) 
 B_SPLINE_CURVE_WITH_KNOTS ( ( 3, 2, 2, 2, 3 ),
 ( 0.8541666666666665186, 0.8611111111111111605, 0.8750000000000000000, 0.8888888888888888395, 0.8958333333333333703 ),
 .UNSPECIFIED. ) 
 CURVE ( )  GEOMETRIC_REPRESENTATION_ITEM ( )  RATIONAL_B_SPLINE_CURVE ( ( 0.9330127018922194093, 0.9330127018922177440, 1.000000000000000000, 0.8660254037844387076, 1.000000000000000000, 0.8660254037844387076, 1.000000000000000000, 0.9330127018922187432, 0.9330127018922192983 ) ) 
 REPRESENTATION_ITEM ( '' )  );
#564=CARTESIAN_POINT ( 'NONE',  ( -82.39999999999999147, -32.81250000000000000, -103.4641016151377499 ) ) ;
#568=EDGE_CURVE ( 'NONE', #13520, #13807, #4419, .T. ) ;
#569=CARTESIAN_POINT ( 'NONE',  ( -81.02178482187500208, -34.60312499938549280, -97.61286128772489690 ) ) ;
#576=CARTESIAN_POINT ( 'NONE',  ( -83.90000000000000568, -33.07500000000000284, 102.5980762113533018 ) ) ;
#579=CARTESIAN_POINT ( 'NONE',  ( 79.64356964375001269, -30.44062499938548783, -98.40857419181659793 ) ) ;
#583=ORIENTED_EDGE ( 'NONE', *, *, #17120, .T. ) ;
#584=CARTESIAN_POINT ( 'NONE',  ( 85.40000000000000568, -30.88124999877097210, 101.7320508075688679 ) ) ;
#590=CARTESIAN_POINT ( 'NONE',  ( -80.90000000000000568, -32.85000000000000142, -102.5980762113533018 ) ) ;
#591=VECTOR ( 'NONE', #8640, 1000.000000000000000 ) ;
#592=VERTEX_POINT ( 'NONE', #17809 ) ;
#593=ORIENTED_EDGE ( 'NONE', *, *, #12880, .F. ) ;
#594=CARTESIAN_POINT ( 'NONE',  ( -82.39999999999999147, -32.50312499938548427, -103.1828516163667899 ) ) ;
#595=CARTESIAN_POINT ( 'NONE',  ( -82.40000000000001990, -33.26250000000000284, 97.00000000000000000 ) ) ;
#596=CARTESIAN_POINT ( 'NONE',  ( 82.40000000000001990, -34.61250000000001137, 103.0000000000000000 ) ) ;
#599=CARTESIAN_POINT ( 'NONE',  ( -83.90000000000000568, -34.96874999877096712, -102.5980762113533018 ) ) ;
#603=( BOUNDED_SURFACE ( )  B_SPLINE_SURFACE ( 1, 2, ( 
 ( #2430, #8389, #14340, #978, #12884, #7121, #7303, #17575, #16392, #7401, #1447, #14820, #3002, #13364, #4186, #11893, #2816, #8773, #17670, #14628, #14530, #4283, #2082, #13260, #11606, #5752, #8863, #13163, #19234, #19135, #5946, #4380, #1359, #11701, #13075, #14723, #17864, #7210, #2911, #2715, #10146, #4475, #10248, #10428, #16210, #8957, #19040, #16301, #5850, #11804, #14926, #8675, #1552, #1162, #5663, #17773, #16108, #10337, #1263, #18372, #17090, #6355, #11224, #11121, #403, #11027, #8104, #9668, #17189, #16990, #4992, #6549, #15628, #16902, #9367, #15723, #13856, #3506, #10935, #12307, #10836, #2234, #12494, #1945, #9564, #13766, #3793, #15530, #3701, #2042, #3602, #9760, #5174, #18465, #18660, #18273, #8200, #5084, #7905, #2146, #4891, #7811, #14057, #14151, #8002, #691, #16805, #785, #6644, #5278, #3415, #6740, #15329, #497, #6451, #12403, #12591, #9465, #12686, #18559, #15430, #13958, #599, #10246, #17668, #19039, #5662, #14626, #10050, #4281, #2518, #2329, #881, #3994, #19132 ),
 ( #13161, #977, #11517, #13074, #7120, #10144, #9858, #8574, #14242, #5571, #17288, #5750, #4185, #17574, #11605, #11699, #16106, #11323, #8673, #1066, #7023, #9959, #6932, #8292, #15913, #2714, #18947, #18756, #11419, #1261, #12881, #17479, #18853, #7208, #2613, #12976, #17380, #6843, #14432, #12787, #5474, #5375, #15820, #3891, #2429, #8475, #8388, #4088, #14339, #16008, #1161, #14528, #1550, #13545, #16299, #13642, #185, #6136, #5848, #12086, #8861, #11891, #18060, #7499, #11802, #4378, #1444, #14818, #7593, #4671, #11990, #17958, #90, #6042, #7398, #12182, #17771, #13258, #4473, #13455, #13362, #3190, #2704, #2999, #10620, #16586, #5944, #10426, #4567, #10336, #10525, #9149, #16492, #16389, #2908, #283, #15112, #3095, #17862, #8955, #14924, #9055, #15020, #4772, #1640, #1727, #7685, #6234, #18150, #16208, #2814, #8770, #14721, #1357, #7301, #19232, #569, #3388, #9537, #12565, #15404, #1825, #18246, #760, #7879, #1916, #9438, #7785, #12282, #2211, #9340, #6524, #2118, #15503, #18533 ) ),
 .UNSPECIFIED., .F., .F., .F. ) 
 B_SPLINE_SURFACE_WITH_KNOTS ( ( 2, 2 ),
 ( 3, 2, 2, 2, 2, 2, 2, 2, 2, 2, 2, 2, 2, 2, 2, 2, 2, 2, 2, 2, 2, 2, 2, 2, 2, 2, 2, 2, 2, 2, 2, 2, 2, 2, 2, 2, 2, 2, 2, 2, 2, 2, 2, 2, 2, 2, 2, 2, 2, 2, 2, 2, 2, 2, 2, 2, 2, 2, 2, 2, 2, 2, 2, 2, 2, 2, 2, 3 ),
 ( 0.000000000000000000, 1.000000000000000000 ),
 ( 0.000000000000000000, 0.01388888888888888812, 0.02777777777777777624, 0.04166666666666666435, 0.05555555555555555247, 0.06944444444444444753, 0.08333333333333332871, 0.09722222222222222376, 0.1111111111111111049, 0.1250000000000000000, 0.1388888888888888951, 0.1527777777777777901, 0.1666666666666666574, 0.1805555555555555525, 0.1944444444444444475, 0.2083333333333333426, 0.2222222222222222099, 0.2361111111111111049, 0.2500000000000000000, 0.2638888888888888951, 0.2777777777777777901, 0.2916666666666666852, 0.3055555555555555802, 0.3194444444444444198, 0.3333333333333333148, 0.3472222222222222099, 0.3611111111111111049, 0.3750000000000000000, 0.3888888888888888951, 0.4027777777777777901, 0.4166666666666666852, 0.4305555555555555802, 0.4444444444444444198, 0.4583333333333333148, 0.4722222222222222099, 0.4861111111111111049, 0.5000000000000000000, 0.5138888888888888395, 0.5277777777777777901, 0.5416666666666666297, 0.5555555555555555802, 0.5694444444444444198, 0.5833333333333333703, 0.5972222222222222099, 0.6111111111111111605, 0.6250000000000000000, 0.6388888888888888395, 0.6527777777777777901, 0.6666666666666666297, 0.6805555555555555802, 0.6944444444444444198, 0.7083333333333333703, 0.7222222222222222099, 0.7361111111111111605, 0.7500000000000000000, 0.7638888888888888395, 0.7777777777777777901, 0.7916666666666666297, 0.8055555555555555802, 0.8194444444444444198, 0.8333333333333333703, 0.8472222222222222099, 0.8611111111111111605, 0.8750000000000000000, 0.8888888888888888395, 0.9027777777777777901, 0.9166666666666666297, 0.9258785144422092550 ),
 .UNSPECIFIED. ) 
 GEOMETRIC_REPRESENTATION_ITEM ( )  RATIONAL_B_SPLINE_SURFACE ( (
 ( 1.000000000000000000, 0.8660254037844387076, 1.000000000000000000, 0.8660254037844387076, 1.000000000000000000, 0.8660254037844387076, 1.000000000000000000, 0.8660254037844387076, 1.000000000000000000, 0.8660254037844387076, 1.000000000000000000, 0.8660254037844387076, 1.000000000000000000, 0.8660254037844387076, 1.000000000000000000, 0.8660254037844387076, 1.000000000000000000, 0.8660254037844387076, 1.000000000000000000, 0.8660254037844387076, 1.000000000000000000, 0.8660254037844387076, 1.000000000000000000, 0.8660254037844387076, 1.000000000000000000, 0.8660254037844387076, 1.000000000000000000, 0.8660254037844387076, 1.000000000000000000, 0.8660254037844387076, 1.000000000000000000, 0.8660254037844387076, 1.000000000000000000, 0.8660254037844387076, 1.000000000000000000, 0.8660254037844387076, 1.000000000000000000, 0.8660254037844387076, 1.000000000000000000, 0.8660254037844387076, 1.000000000000000000, 0.8660254037844387076, 1.000000000000000000, 0.8660254037844387076, 1.000000000000000000, 0.8660254037844387076, 1.000000000000000000, 0.8660254037844387076, 1.000000000000000000, 0.8660254037844387076, 1.000000000000000000, 0.8660254037844387076, 1.000000000000000000, 0.8660254037844387076, 1.000000000000000000, 0.8660254037844387076, 1.000000000000000000, 0.8660254037844387076, 1.000000000000000000, 0.8660254037844387076, 1.000000000000000000, 0.8660254037844387076, 1.000000000000000000, 0.8660254037844387076, 1.000000000000000000, 0.8660254037844387076, 1.000000000000000000, 0.8660254037844387076, 1.000000000000000000, 0.8660254037844387076, 1.000000000000000000, 0.8660254037844387076, 1.000000000000000000, 0.8660254037844387076, 1.000000000000000000, 0.8660254037844387076, 1.000000000000000000, 0.8660254037844387076, 1.000000000000000000, 0.8660254037844387076, 1.000000000000000000, 0.8660254037844387076, 1.000000000000000000, 0.8660254037844387076, 1.000000000000000000, 0.8660254037844387076, 1.000000000000000000, 0.8660254037844387076, 1.000000000000000000, 0.8660254037844387076, 1.000000000000000000, 0.8660254037844387076, 1.000000000000000000, 0.8660254037844387076, 1.000000000000000000, 0.8660254037844387076, 1.000000000000000000, 0.8660254037844387076, 1.000000000000000000, 0.8660254037844387076, 1.000000000000000000, 0.8660254037844387076, 1.000000000000000000, 0.8660254037844387076, 1.000000000000000000, 0.8660254037844387076, 1.000000000000000000, 0.8660254037844387076, 1.000000000000000000, 0.8660254037844387076, 1.000000000000000000, 0.8660254037844387076, 1.000000000000000000, 0.8660254037844387076, 1.000000000000000000, 0.8660254037844387076, 1.000000000000000000, 0.8660254037844387076, 1.000000000000000000, 0.8660254037844387076, 1.000000000000000000, 0.8660254037844387076, 1.000000000000000000, 0.8660254037844387076, 1.000000000000000000, 0.8660254037844387076, 1.000000000000000000, 0.8660254037844387076, 1.000000000000000000, 0.8660254037844387076, 1.000000000000000000, 0.8660254037844387076, 1.000000000000000000, 0.9111409417988175496, 0.9401539645359766606),
 ( 1.000000000000000000, 0.8660254037844387076, 1.000000000000000000, 0.8660254037844387076, 1.000000000000000000, 0.8660254037844387076, 1.000000000000000000, 0.8660254037844387076, 1.000000000000000000, 0.8660254037844387076, 1.000000000000000000, 0.8660254037844387076, 1.000000000000000000, 0.8660254037844387076, 1.000000000000000000, 0.8660254037844387076, 1.000000000000000000, 0.8660254037844387076, 1.000000000000000000, 0.8660254037844387076, 1.000000000000000000, 0.8660254037844387076, 1.000000000000000000, 0.8660254037844387076, 1.000000000000000000, 0.8660254037844387076, 1.000000000000000000, 0.8660254037844387076, 1.000000000000000000, 0.8660254037844387076, 1.000000000000000000, 0.8660254037844387076, 1.000000000000000000, 0.8660254037844387076, 1.000000000000000000, 0.8660254037844387076, 1.000000000000000000, 0.8660254037844387076, 1.000000000000000000, 0.8660254037844387076, 1.000000000000000000, 0.8660254037844387076, 1.000000000000000000, 0.8660254037844387076, 1.000000000000000000, 0.8660254037844387076, 1.000000000000000000, 0.8660254037844387076, 1.000000000000000000, 0.8660254037844387076, 1.000000000000000000, 0.8660254037844387076, 1.000000000000000000, 0.8660254037844387076, 1.000000000000000000, 0.8660254037844387076, 1.000000000000000000, 0.8660254037844387076, 1.000000000000000000, 0.8660254037844387076, 1.000000000000000000, 0.8660254037844387076, 1.000000000000000000, 0.8660254037844387076, 1.000000000000000000, 0.8660254037844387076, 1.000000000000000000, 0.8660254037844387076, 1.000000000000000000, 0.8660254037844387076, 1.000000000000000000, 0.8660254037844387076, 1.000000000000000000, 0.8660254037844387076, 1.000000000000000000, 0.8660254037844387076, 1.000000000000000000, 0.8660254037844387076, 1.000000000000000000, 0.8660254037844387076, 1.000000000000000000, 0.8660254037844387076, 1.000000000000000000, 0.8660254037844387076, 1.000000000000000000, 0.8660254037844387076, 1.000000000000000000, 0.8660254037844387076, 1.000000000000000000, 0.8660254037844387076, 1.000000000000000000, 0.8660254037844387076, 1.000000000000000000, 0.8660254037844387076, 1.000000000000000000, 0.8660254037844387076, 1.000000000000000000, 0.8660254037844387076, 1.000000000000000000, 0.8660254037844387076, 1.000000000000000000, 0.8660254037844387076, 1.000000000000000000, 0.8660254037844387076, 1.000000000000000000, 0.8660254037844387076, 1.000000000000000000, 0.8660254037844387076, 1.000000000000000000, 0.8660254037844387076, 1.000000000000000000, 0.8660254037844387076, 1.000000000000000000, 0.8660254037844387076, 1.000000000000000000, 0.8660254037844387076, 1.000000000000000000, 0.8660254037844387076, 1.000000000000000000, 0.8660254037844387076, 1.000000000000000000, 0.8660254037844387076, 1.000000000000000000, 0.8660254037844387076, 1.000000000000000000, 0.8660254037844387076, 1.000000000000000000, 0.8660254037844387076, 1.000000000000000000, 0.8660254037844387076, 1.000000000000000000, 0.8660254037844387076, 1.000000000000000000, 0.9111409417988175496, 0.9401539645359766606) ) ) 
 REPRESENTATION_ITEM ( '' )  SURFACE ( )  );
#606=CARTESIAN_POINT ( 'NONE',  ( 81.59615242270662350, -34.12634618820329990, -96.99999999999998579 ) ) ;
#609=VERTEX_POINT ( 'NONE', #4327 ) ;
#610=CARTESIAN_POINT ( 'NONE',  ( -79.64356964375001269, -34.82812499938548711, -101.5914258081833879 ) ) ;
#611=CARTESIAN_POINT ( 'NONE',  ( 82.40000000000000568, -30.00000000000000355, -96.99999999999998579 ) ) ;
#620=ORIENTED_EDGE ( 'NONE', *, *, #7465, .T. ) ;
#621=CARTESIAN_POINT ( 'NONE',  ( -84.44763168836716716, -32.00000000000000000, 101.8452947671445799 ) ) ;
#622=CARTESIAN_POINT ( 'NONE',  ( 80.90000000000000568, -30.30000000000000426, -102.5980762113533018 ) ) ;
#624=CARTESIAN_POINT ( 'NONE',  ( -85.40000000000000568, -35.36739044046696279, 98.90809476984486537 ) ) ;
#626=CARTESIAN_POINT ( 'NONE',  ( 83.20384757729337366, -32.15759618943233278, -103.0000000000000000 ) ) ;
#628=CARTESIAN_POINT ( 'NONE',  ( 83.77821517812500929, -34.22812499938549280, -102.3871387122750889 ) ) ;
#630=CARTESIAN_POINT ( 'NONE',  ( -79.64356964375001269, -32.12812499938548427, 98.40857419181659793 ) ) ;
#631=CARTESIAN_POINT ( 'NONE',  ( 79.64356964374999848, -33.96562499938548285, -99.99999999999998579 ) ) ;
#634=CARTESIAN_POINT ( 'NONE',  ( -80.90000000000000568, -33.89999999999999858, 102.5980762113533018 ) ) ;
#635=( BOUNDED_CURVE ( )  B_SPLINE_CURVE ( 2, ( #15798, #17169, #11586, #14410, #9739, #11298, #14220, #11396, #15704 ),
 .UNSPECIFIED., .F., .F. ) 
 B_SPLINE_CURVE_WITH_KNOTS ( ( 3, 2, 2, 2, 3 ),
 ( 0.6458333333333333703, 0.6527777777777777901, 0.6666666666666666297, 0.6805555555555555802, 0.6875000000000000000 ),
 .UNSPECIFIED. ) 
 CURVE ( )  GEOMETRIC_REPRESENTATION_ITEM ( )  RATIONAL_B_SPLINE_CURVE ( ( 0.9330127018922192983, 0.9330127018922198534, 1.000000000000000000, 0.8660254037844387076, 1.000000000000000000, 0.8660254037844387076, 1.000000000000000000, 0.9330127018922194093, 0.9330127018922194093 ) ) 
 REPRESENTATION_ITEM ( '' )  );
#640=CARTESIAN_POINT ( 'NONE',  ( -80.90000000000000568, -32.55000000000000426, 102.5980762113533018 ) ) ;
#644=CARTESIAN_POINT ( 'NONE',  ( 83.77821517812500929, -31.56562499938548427, 102.3871387122750889 ) ) ;
#648=CARTESIAN_POINT ( 'NONE',  ( -83.77821517812500929, -32.42812499938548854, -97.61286128772489690 ) ) ;
#649=CARTESIAN_POINT ( 'NONE',  ( 79.64356964375001269, -32.12812499938548427, 101.5914258081833879 ) ) ;
#651=CARTESIAN_POINT ( 'NONE',  ( 85.15643035624999868, -30.66562499938548569, -101.5914258081833879 ) ) ;
#653=CARTESIAN_POINT ( 'NONE',  ( -85.15643035625001289, -34.34062499938548285, 98.40857419181659793 ) ) ;
#654=CARTESIAN_POINT ( 'NONE',  ( -81.02178482187500208, -32.80312499938548854, -97.61286128772489690 ) ) ;
#655=ORIENTED_EDGE ( 'NONE', *, *, #15701, .F. ) ;
#656=CARTESIAN_POINT ( 'NONE',  ( 81.02178482187500208, -32.80312499938548854, 97.61286128772489690 ) ) ;
#658=CARTESIAN_POINT ( 'NONE',  ( -79.64356964374999848, -30.36562499938548498, 99.99999999999998579 ) ) ;
#659=CARTESIAN_POINT ( 'NONE',  ( -79.64356964374999848, -34.07812499938548711, 99.99999999999998579 ) ) ;
#661=EDGE_LOOP ( 'NONE', ( #10048, #2017, #17543, #5703 ) ) ;
#662=CARTESIAN_POINT ( 'NONE',  ( -79.39999999999999147, -32.43750000000000000, -101.7320508075688821 ) ) ;
#666=DIRECTION ( 'NONE',  ( 0.000000000000000000, 0.000000000000000000, -1.000000000000000000 ) ) ;
#671=CARTESIAN_POINT ( 'NONE',  ( 82.40000000000000568, -30.00000000000000355, -99.99999999999998579 ) ) ;
#674=DIRECTION ( 'NONE',  ( -0.000000000000000000, -0.000000000000000000, -1.000000000000000000 ) ) ;
#675=CARTESIAN_POINT ( 'NONE',  ( 85.15643035625001289, -30.70312499938548711, -99.99999999999998579 ) ) ;
#678=( BOUNDED_CURVE ( )  B_SPLINE_CURVE ( 2, ( #4464, #17947, #13065, #17565, #8947, #19221, #11597, #8854, #5742 ),
 .UNSPECIFIED., .F., .F. ) 
 B_SPLINE_CURVE_WITH_KNOTS ( ( 3, 2, 2, 2, 3 ),
 ( 0.3958333333333334259, 0.4027777777777777901, 0.4166666666666666852, 0.4305555555555555802, 0.4374999999999999445 ),
 .UNSPECIFIED. ) 
 CURVE ( )  GEOMETRIC_REPRESENTATION_ITEM ( )  RATIONAL_B_SPLINE_CURVE ( ( 0.9330127018922192983, 0.9330127018922200755, 1.000000000000000000, 0.8660254037844387076, 1.000000000000000000, 0.8660254037844387076, 1.000000000000000000, 0.9330127018922198534, 0.9330127018922192983 ) ) 
 REPRESENTATION_ITEM ( '' )  );
#679=CARTESIAN_POINT ( 'NONE',  ( 79.39999999999999147, -31.03124999877097068, 101.7320508075688821 ) ) ;
#684=CARTESIAN_POINT ( 'NONE',  ( -79.39999999999999147, -32.92500000000000426, -99.99999999999998579 ) ) ;
#686=ORIENTED_EDGE ( 'NONE', *, *, #7224, .F. ) ;
#687=CARTESIAN_POINT ( 'NONE',  ( -85.15643035624999868, -31.07812499938548356, -101.5914258081833879 ) ) ;
#688=CARTESIAN_POINT ( 'NONE',  ( -83.20384757729337366, -32.34240381056766722, -103.0000000000000000 ) ) ;
#690=CARTESIAN_POINT ( 'NONE',  ( 83.77821517812500929, -33.32812499938548711, 97.61286128772489690 ) ) ;
#691=CARTESIAN_POINT ( 'NONE',  ( -82.39999999999999147, -34.33124999877097139, -96.53589838486223584 ) ) ;
#692=CARTESIAN_POINT ( 'NONE',  ( 82.39999999999999147, -33.93750000000000000, 96.53589838486223584 ) ) ;
#695=EDGE_CURVE ( 'NONE', #5463, #11282, #11271, .T. ) ;
#699=CARTESIAN_POINT ( 'NONE',  ( 83.90000000000000568, -30.46874999877096712, -97.40192378864668399 ) ) ;
#702=CARTESIAN_POINT ( 'NONE',  ( 83.77821517812500929, -33.36562499938548854, -97.61286128772489690 ) ) ;
#704=EDGE_CURVE ( 'NONE', #8584, #4219, #13266, .T. ) ;
#708=CARTESIAN_POINT ( 'NONE',  ( 82.40000000000000568, -30.00000000000000355, -103.0000000000000000 ) ) ;
#717=CARTESIAN_POINT ( 'NONE',  ( 81.02178482187500208, -34.79062499938548569, -97.61286128772489690 ) ) ;
#719=CARTESIAN_POINT ( 'NONE',  ( -83.90000000000000568, -33.91874999877096997, 102.5980762113533018 ) ) ;
#721=DIRECTION ( 'NONE',  ( -0.000000000000000000, -0.000000000000000000, -1.000000000000000000 ) ) ;
#723=CARTESIAN_POINT ( 'NONE',  ( 79.64356964374999848, -32.16562499938548569, 99.99999999999998579 ) ) ;
#725=CARTESIAN_POINT ( 'NONE',  ( -83.77821517812500929, -33.21562499938548285, 102.3871387122750889 ) ) ;
#729=VERTEX_POINT ( 'NONE', #6372 ) ;
#731=CARTESIAN_POINT ( 'NONE',  ( -80.90000000000000568, -34.80000000000000426, 102.5980762113533018 ) ) ;
#735=CARTESIAN_POINT ( 'NONE',  ( -79.39999999999999147, -32.88750000000000284, 98.26794919243110371 ) ) ;
#736=ORIENTED_EDGE ( 'NONE', *, *, #13637, .F. ) ;
#737=CARTESIAN_POINT ( 'NONE',  ( -82.32247963938036150, -35.00000000000000711, -97.23891671615864141 ) ) ;
#738=CARTESIAN_POINT ( 'NONE',  ( 81.02178482187500208, -33.59062499938548285, 97.61286128772489690 ) ) ;
#739=CARTESIAN_POINT ( 'NONE',  ( 85.40000000000000568, -32.60624999877096997, -101.7320508075688821 ) ) ;
#741=CARTESIAN_POINT ( 'NONE',  ( 83.52979456739228681, -32.00000000000000000, 97.41965524898084539 ) ) ;
#742=CARTESIAN_POINT ( 'NONE',  ( 83.77821517812500929, -31.41562499938548569, 97.61286128772489690 ) ) ;
#744=CARTESIAN_POINT ( 'NONE',  ( 85.15643035624999868, -32.54062499938548569, -98.40857419181659793 ) ) ;
#746=CARTESIAN_POINT ( 'NONE',  ( -82.39999999999999147, -33.51562499938548711, 96.81714838363319586 ) ) ;
#747=CARTESIAN_POINT ( 'NONE',  ( -83.77821517812500929, -30.96562499938548640, -97.61286128772489690 ) ) ;
#748=ORIENTED_EDGE ( 'NONE', *, *, #11145, .T. ) ;
#749=CARTESIAN_POINT ( 'NONE',  ( 79.64356964374999848, -33.62812499938548427, 99.99999999999998579 ) ) ;
#751=CARTESIAN_POINT ( 'NONE',  ( -85.15643035624999868, -31.45312499938548356, 101.5914258081833879 ) ) ;
#752=CARTESIAN_POINT ( 'NONE',  ( -85.15643035624999868, -34.34062499938548285, 98.40857419181659793 ) ) ;
#753=CARTESIAN_POINT ( 'NONE',  ( 85.40000000000000568, -34.95000000000000284, 99.99999999999998579 ) ) ;
#755=CARTESIAN_POINT ( 'NONE',  ( -85.40000000000000568, -34.01250000000000284, -98.26794919243111792 ) ) ;
#760=CARTESIAN_POINT ( 'NONE',  ( -82.39999999999999147, -34.86562499938548854, -103.1828516163667899 ) ) ;
#763=CYLINDRICAL_SURFACE ( 'NONE', #16164, 3.000000000000002665 ) ;
#766=CARTESIAN_POINT ( 'NONE',  ( 85.15643035624999868, -31.11562499938548854, 98.40857419181659793 ) ) ;
#768=CARTESIAN_POINT ( 'NONE',  ( 81.02178482187500208, -30.55312499938548854, -102.3871387122750889 ) ) ;
#772=CARTESIAN_POINT ( 'NONE',  ( 79.39999999999999147, -30.65624999877096712, 98.26794919243113213 ) ) ;
#777=CYLINDRICAL_SURFACE ( 'NONE', #18363, 3.000000000000002665 ) ;
#778=ORIENTED_EDGE ( 'NONE', *, *, #4094, .F. ) ;
#779=VERTEX_POINT ( 'NONE', #3045 ) ;
#780=CARTESIAN_POINT ( 'NONE',  ( -83.77821517812500929, -32.31562499938548427, -97.61286128772489690 ) ) ;
#781=CARTESIAN_POINT ( 'NONE',  ( -82.39999999999999147, -33.65624999877097423, -103.0000000000000000 ) ) ;
#784=CARTESIAN_POINT ( 'NONE',  ( 82.39999999999999147, -32.84062499938548996, 96.81714838363319586 ) ) ;
#785=CARTESIAN_POINT ( 'NONE',  ( -85.40000000000000568, -34.40624999877096712, -98.26794919243111792 ) ) ;
#786=CARTESIAN_POINT ( 'NONE',  ( 84.69814068649969840, -35.00052333152936512, 101.9283540611242955 ) ) ;
#790=CARTESIAN_POINT ( 'NONE',  ( 85.00132729415355470, -35.00000000000000711, -101.2112556744910563 ) ) ;
#792=DIRECTION ( 'NONE',  ( 0.000000000000000000, 0.000000000000000000, 1.000000000000000000 ) ) ;
#796=CARTESIAN_POINT ( 'NONE',  ( 85.15643035625001289, -32.42812499938548854, -98.40857419181659793 ) ) ;
#799=( BOUNDED_CURVE ( )  B_SPLINE_CURVE ( 2, ( #10926, #13757, #590, #3595, #684, #1937, #18265, #395, #18168 ),
 .UNSPECIFIED., .F., .F. ) 
 B_SPLINE_CURVE_WITH_KNOTS ( ( 3, 2, 2, 2, 3 ),
 ( 0.5208333333333333703, 0.5277777777777777901, 0.5416666666666666297, 0.5555555555555555802, 0.5625000000000000000 ),
 .UNSPECIFIED. ) 
 CURVE ( )  GEOMETRIC_REPRESENTATION_ITEM ( )  RATIONAL_B_SPLINE_CURVE ( ( 0.9330127018922192983, 0.9330127018922198534, 1.000000000000000000, 0.8660254037844387076, 1.000000000000000000, 0.8660254037844387076, 1.000000000000000000, 0.9330127018922194093, 0.9330127018922194093 ) ) 
 REPRESENTATION_ITEM ( '' )  );
#800=VERTEX_POINT ( 'NONE', #18004 ) ;
#807=LINE ( 'NONE', #9075, #14712 ) ;
#810=CARTESIAN_POINT ( 'NONE',  ( 80.90000000000000568, -33.45000000000000284, -102.5980762113533018 ) ) ;
#812=CARTESIAN_POINT ( 'NONE',  ( -80.90000000000000568, -35.19374999877096855, 102.5980762113533018 ) ) ;
#817=CARTESIAN_POINT ( 'NONE',  ( 79.64356964374998427, -34.49062499938548854, -98.40857419181659793 ) ) ;
#819=CARTESIAN_POINT ( 'NONE',  ( -79.64356964375001269, -32.20312499938548001, 101.5914258081833879 ) ) ;
#821=DIRECTION ( 'NONE',  ( 1.000000000000000000, 0.000000000000000000, -0.000000000000000000 ) ) ;
#825=B_SPLINE_CURVE_WITH_KNOTS ( 'NONE', 3,
 ( #10025, #11490, #16078, #19109, #7092, #14796, #5637, #14603, #19208, #11583, #2686, #5729, #17454, #4257, #5823, #8742, #8643, #2588 ),
 .UNSPECIFIED., .F., .F.,
 ( 4, 2, 2, 2, 2, 2, 2, 2, 4 ),
 ( 0.000000000000000000, 0.0007106627595359116300, 0.001421325519071823260, 0.002131988278607734998, 0.002842651038143646520, 0.003553313797679558041, 0.004263976557215469997, 0.004974639316751381518, 0.005685302076287293040 ),
 .UNSPECIFIED. ) ;
#826=FACE_OUTER_BOUND ( 'NONE', #7143, .T. ) ;
#827=CARTESIAN_POINT ( 'NONE',  ( 85.40000000000000568, -33.60000000000000142, 99.99999999999998579 ) ) ;
#831=ADVANCED_FACE ( 'NONE', ( #1967 ), #1871, .F. ) ;
#835=CARTESIAN_POINT ( 'NONE',  ( 85.15643035625001289, -31.94062499938548427, 99.99999999999998579 ) ) ;
#838=CARTESIAN_POINT ( 'NONE',  ( 84.44763168836732348, -32.00000000000002132, 98.15470523285560489 ) ) ;
#839=CARTESIAN_POINT ( 'NONE',  ( 85.15643035625001289, -32.84062499938548285, 99.99999999999998579 ) ) ;
#840=CARTESIAN_POINT ( 'NONE',  ( 79.64356964375001269, -33.21562499938548996, -101.5914258081833879 ) ) ;
#842=CARTESIAN_POINT ( 'NONE',  ( -79.64356964374998427, -34.45312499938548711, 101.5914258081833879 ) ) ;
#844=CARTESIAN_POINT ( 'NONE',  ( 85.15643035624999868, -32.09062499938548996, 101.5914258081833879 ) ) ;
#847=CARTESIAN_POINT ( 'NONE',  ( -82.39999999999999147, -30.92812499938548143, 103.1828516163667899 ) ) ;
#848=CARTESIAN_POINT ( 'NONE',  ( -85.15643035625001289, -31.94062499938548427, 99.99999999999998579 ) ) ;
#851=CARTESIAN_POINT ( 'NONE',  ( -79.39999999999999147, -34.23750000000000426, -101.7320508075688821 ) ) ;
#855=CIRCLE ( 'NONE', #7750, 2.649999999999982148 ) ;
#857=CARTESIAN_POINT ( 'NONE',  ( -85.40000000000000568, -34.53750000000000142, 98.26794919243111792 ) ) ;
#858=CARTESIAN_POINT ( 'NONE',  ( -80.90000000000000568, -32.94374999877096855, 102.5980762113533018 ) ) ;
#859=CYLINDRICAL_SURFACE ( 'NONE', #3213, 3.000000000000002665 ) ;
#860=CARTESIAN_POINT ( 'NONE',  ( 79.64356964374998427, -34.82812499938548711, 101.5914258081833879 ) ) ;
#861=CARTESIAN_POINT ( 'NONE',  ( 85.15643035624999868, -30.74062499938548143, 101.5914258081833879 ) ) ;
#863=VECTOR ( 'NONE', #18702, 1000.000000000000000 ) ;
#864=CARTESIAN_POINT ( 'NONE',  ( -85.40000000000000568, -32.73750000000000426, -101.7320508075688821 ) ) ;
#865=CARTESIAN_POINT ( 'NONE',  ( 83.77821517812500929, -31.22812499938548569, -97.61286128772489690 ) ) ;
#866=CARTESIAN_POINT ( 'NONE',  ( 81.59615242270662350, -32.96115380933864003, 97.00000000000000000 ) ) ;
#867=VERTEX_POINT ( 'NONE', #16826 ) ;
#876=CARTESIAN_POINT ( 'NONE',  ( -82.39999999999999147, -31.15312499938548640, -103.1828516163667899 ) ) ;
#879=CARTESIAN_POINT ( 'NONE',  ( 83.77821517812500929, -34.37812499938548427, 102.3871387122750889 ) ) ;
#880=VECTOR ( 'NONE', #2468, 1000.000000000000000 ) ;
#881=CARTESIAN_POINT ( 'NONE',  ( -85.40000000000000568, -35.34374999877096712, -99.99999999999998579 ) ) ;
#882=CARTESIAN_POINT ( 'NONE',  ( 85.40000000000000568, -34.91250000000000142, 98.26794919243111792 ) ) ;
#883=CARTESIAN_POINT ( 'NONE',  ( 79.39999999999999147, -34.63124999877096855, -98.26794919243110371 ) ) ;
#887=CARTESIAN_POINT ( 'NONE',  ( -79.64356964374998427, -32.57812499938548711, -101.5914258081833879 ) ) ;
#889=CARTESIAN_POINT ( 'NONE',  ( -82.40000000000000568, -34.10624999877096997, -102.9999999999999858 ) ) ;
#892=EDGE_CURVE ( 'NONE', #2299, #18536, #6552, .T. ) ;
#893=VERTEX_POINT ( 'NONE', #7634 ) ;
#895=CARTESIAN_POINT ( 'NONE',  ( -81.02178482187500208, -34.94062499938548427, -97.61286128772489690 ) ) ;
#903=CARTESIAN_POINT ( 'NONE',  ( 99.99999999999994316, -35.00000000000000000, -150.0000000000000000 ) ) ;
#906=CARTESIAN_POINT ( 'NONE',  ( 85.40000000000000568, -32.66250000000000142, -101.7320508075688679 ) ) ;
#909=CARTESIAN_POINT ( 'NONE',  ( -79.64356964375001269, -30.89062499938548711, 98.40857419181659793 ) ) ;
#914=CARTESIAN_POINT ( 'NONE',  ( 82.39999999999999147, -34.86562499938548854, -96.81714838363319586 ) ) ;
#916=CARTESIAN_POINT ( 'NONE',  ( -81.02178482187500208, -32.24062499938548854, 102.3871387122750889 ) ) ;
#921=CARTESIAN_POINT ( 'NONE',  ( -82.40000000000000568, -30.00000000000000355, -99.99999999999998579 ) ) ;
#922=LINE ( 'NONE', #17517, #863 ) ;
#931=CARTESIAN_POINT ( 'NONE',  ( 83.77821517812500929, -31.86562499938548498, 97.61286128772489690 ) ) ;
#936=CARTESIAN_POINT ( 'NONE',  ( -83.77821517812500929, -33.92812499938548854, -102.3871387122750889 ) ) ;
#937=CARTESIAN_POINT ( 'NONE',  ( 79.64356964375001269, -32.65312499938548285, 98.40857419181659793 ) ) ;
#938=CARTESIAN_POINT ( 'NONE',  ( 79.64356964375001269, -34.11562499938548854, -101.5914258081833879 ) ) ;
#940=CARTESIAN_POINT ( 'NONE',  ( -79.64356964374998427, -33.55312499938548854, 101.5914258081833879 ) ) ;
#941=CARTESIAN_POINT ( 'NONE',  ( 79.64356964374999848, -30.81562499938548427, -99.99999999999998579 ) ) ;
#942=ORIENTED_EDGE ( 'NONE', *, *, #12020, .F. ) ;
#948=CARTESIAN_POINT ( 'NONE',  ( -85.15643035624999868, -31.00312499938548072, 101.5914258081833879 ) ) ;
#949=CARTESIAN_POINT ( 'NONE',  ( -79.64356964374999848, -30.81562499938548427, 99.99999999999998579 ) ) ;
#952=CARTESIAN_POINT ( 'NONE',  ( -82.39999999999999147, -33.26250000000000284, -103.4641016151377499 ) ) ;
#955=CARTESIAN_POINT ( 'NONE',  ( -99.99999999999998579, 0.000000000000000000, -150.0000000000000000 ) ) ;
#961=CARTESIAN_POINT ( 'NONE',  ( -85.40000000000000568, -33.09374999877096712, -99.99999999999998579 ) ) ;
#962=CARTESIAN_POINT ( 'NONE',  ( -84.28136653320154892, -32.00000000000001421, 97.98546077809197641 ) ) ;
#963=CARTESIAN_POINT ( 'NONE',  ( -82.40000000000001990, -32.53124999877097423, -97.00000000000000000 ) ) ;
#964=CARTESIAN_POINT ( 'NONE',  ( 79.64356964375001269, -33.21562499938548996, -101.5914258081833879 ) ) ;
#967=CARTESIAN_POINT ( 'NONE',  ( 80.90000000000000568, -31.44374999877096855, 102.5980762113533018 ) ) ;
#970=CYLINDRICAL_SURFACE ( 'NONE', #13030, 2.649999999999985700 ) ;
#971=CARTESIAN_POINT ( 'NONE',  ( -85.24876232368482931, -35.00000000000000711, -99.45334139305025190 ) ) ;
#973=CARTESIAN_POINT ( 'NONE',  ( -79.64356964375001269, -31.75312499938548427, -98.40857419181659793 ) ) ;
#974=CARTESIAN_POINT ( 'NONE',  ( 80.90000000000000568, -32.34374999877096712, 102.5980762113533018 ) ) ;
#976=CARTESIAN_POINT ( 'NONE',  ( 85.15643035625001289, -33.40312499938548285, 99.99999999999998579 ) ) ;
#977=CARTESIAN_POINT ( 'NONE',  ( -85.15643035624999868, -30.29062499938548925, -101.5914258081833879 ) ) ;
#978=CARTESIAN_POINT ( 'NONE',  ( -82.39999999999999147, -30.50624999877097210, -103.4641016151377499 ) ) ;
#982=CARTESIAN_POINT ( 'NONE',  ( -81.02178482187500208, -32.99062499938548854, -102.3871387122750889 ) ) ;
#984=CARTESIAN_POINT ( 'NONE',  ( 79.39999999999999147, -31.55624999877096926, -101.7320508075688537 ) ) ;
#986=EDGE_LOOP ( 'NONE', ( #10879, #13324, #8010, #1433 ) ) ;
#987=CARTESIAN_POINT ( 'NONE',  ( 79.64356964374998427, -33.92812499938548854, -98.40857419181659793 ) ) ;
#990=ORIENTED_EDGE ( 'NONE', *, *, #12505, .T. ) ;
#992=CARTESIAN_POINT ( 'NONE',  ( -82.40000000000001990, -32.30624999877097281, -103.0000000000000000 ) ) ;
#999=CARTESIAN_POINT ( 'NONE',  ( 83.90000000000000568, -33.97500000000000853, -102.5980762113533018 ) ) ;
#1000=CARTESIAN_POINT ( 'NONE',  ( 81.45486068924890333, -31.99999999999999289, -102.7533691519569885 ) ) ;
#1003=CARTESIAN_POINT ( 'NONE',  ( -79.64356964375001269, -31.86562499938548143, 101.5914258081833879 ) ) ;
#1005=CARTESIAN_POINT ( 'NONE',  ( -82.40000000000000568, -30.00000000000000355, -99.99999999999998579 ) ) ;
#1007=DIRECTION ( 'NONE',  ( 0.000000000000000000, 0.000000000000000000, 1.000000000000000000 ) ) ;
#1009=CYLINDRICAL_SURFACE ( 'NONE', #18973, 3.000000000000002665 ) ;
#1010=PLANE ( 'NONE',  #18028 ) ;
#1015=VECTOR ( 'NONE', #7998, 1000.000000000000000 ) ;
#1020=EDGE_CURVE ( 'NONE', #14645, #2256, #5419, .T. ) ;
#1024=CARTESIAN_POINT ( 'NONE',  ( -80.90000000000000568, -30.54374999877096997, 97.40192378864668399 ) ) ;
#1025=CARTESIAN_POINT ( 'NONE',  ( 82.39999999999999147, -34.52812499938548996, 96.81714838363319586 ) ) ;
#1029=CARTESIAN_POINT ( 'NONE',  ( -79.64356964374998427, -34.56562499938548427, -98.40857419181659793 ) ) ;
#1030=CARTESIAN_POINT ( 'NONE',  ( 83.77821517812500929, -31.86562499938548498, 97.61286128772489690 ) ) ;
#1031=CARTESIAN_POINT ( 'NONE',  ( 79.64356964374999848, -34.97812499938548569, -99.99999999999998579 ) ) ;
#1033=CARTESIAN_POINT ( 'NONE',  ( -79.64356964374998427, -34.00312499938548427, 101.5914258081833879 ) ) ;
#1034=CARTESIAN_POINT ( 'NONE',  ( 82.39999999999999147, -30.92812499938548143, -103.1828516163667899 ) ) ;
#1035=ORIENTED_EDGE ( 'NONE', *, *, #18905, .F. ) ;
#1040=CARTESIAN_POINT ( 'NONE',  ( -79.64356964375001269, -33.55312499938548854, 101.5914258081833879 ) ) ;
#1041=CARTESIAN_POINT ( 'NONE',  ( -85.15643035624999868, -30.62812499938548427, 98.40857419181659793 ) ) ;
#1046=CARTESIAN_POINT ( 'NONE',  ( 82.39999999999999147, -33.48750000000000426, -103.0000000000000000 ) ) ;
#1049=CARTESIAN_POINT ( 'NONE',  ( -82.39999999999999147, -32.98124999877096286, 102.9999999999999858 ) ) ;
#1052=CARTESIAN_POINT ( 'NONE',  ( -83.20384757729335945, -32.73615380933863150, -102.9999999999999716 ) ) ;
#1053=CARTESIAN_POINT ( 'NONE',  ( 83.77821517812500929, -33.92812499938548854, -97.61286128772489690 ) ) ;
#1055=ORIENTED_EDGE ( 'NONE', *, *, #18470, .T. ) ;
#1056=CARTESIAN_POINT ( 'NONE',  ( 85.40000000000000568, -33.99374999877097281, 99.99999999999998579 ) ) ;
#1062=CARTESIAN_POINT ( 'NONE',  ( -79.64356964375001269, -34.90312499938548285, -98.40857419181659793 ) ) ;
#1063=DIRECTION ( 'NONE',  ( 0.000000000000000000, 0.000000000000000000, -1.000000000000000000 ) ) ;
#1065=CARTESIAN_POINT ( 'NONE',  ( 79.64356964374998427, -32.69062499938548427, 101.5914258081833879 ) ) ;
#1066=CARTESIAN_POINT ( 'NONE',  ( -79.64356964375001269, -30.96562499938548640, -98.40857419181659793 ) ) ;
#1067=CARTESIAN_POINT ( 'NONE',  ( 79.39999999999999147, -34.31250000000000000, 98.26794919243113213 ) ) ;
#1068=CARTESIAN_POINT ( 'NONE',  ( -94.79999999999999716, -32.00000000000000000, 150.0000000000000000 ) ) ;
#1071=CARTESIAN_POINT ( 'NONE',  ( -82.39999999999999147, -32.95312499938548711, -103.1828516163667899 ) ) ;
#1073=CARTESIAN_POINT ( 'NONE',  ( 83.90000000000000568, -30.91874999877096997, -97.40192378864668399 ) ) ;
#1076=PLANE ( 'NONE',  #99 ) ;
#1078=CARTESIAN_POINT ( 'NONE',  ( -82.40000000000000568, -30.00000000000000355, 103.0000000000000000 ) ) ;
#1080=ADVANCED_FACE ( 'NONE', ( #6860 ), #15549, .T. ) ;
#1084=LINE ( 'NONE', #11915, #8796 ) ;
#1085=ORIENTED_EDGE ( 'NONE', *, *, #3636, .F. ) ;
#1086=CARTESIAN_POINT ( 'NONE',  ( 80.90000000000000568, -32.55000000000000426, -102.5980762113533018 ) ) ;
#1087=CARTESIAN_POINT ( 'NONE',  ( 83.74167325096733805, -31.99999999999999289, -102.4658751321106536 ) ) ;
#1088=CARTESIAN_POINT ( 'NONE',  ( -85.15643035625001289, -31.15312499938548996, 99.99999999999998579 ) ) ;
#1091=CARTESIAN_POINT ( 'NONE',  ( 83.77821517812500929, -34.37812499938548427, -97.61286128772489690 ) ) ;
#1094=FACE_OUTER_BOUND ( 'NONE', #17811, .T. ) ;
#1097=CARTESIAN_POINT ( 'NONE',  ( -81.02178482187500208, -30.44062499938548783, -97.61286128772489690 ) ) ;
#1098=CARTESIAN_POINT ( 'NONE',  ( -82.40000000000000568, -30.00000000000000355, 103.0000000000000000 ) ) ;
#1101=CARTESIAN_POINT ( 'NONE',  ( -85.40000000000000568, -34.91250000000000142, -98.26794919243111792 ) ) ;
#1107=CARTESIAN_POINT ( 'NONE',  ( 85.40000000000000568, -32.19374999877096855, -99.99999999999998579 ) ) ;
#1108=CARTESIAN_POINT ( 'NONE',  ( 81.02178482187500208, -34.04062499938548569, 97.61286128772489690 ) ) ;
#1109=DIRECTION ( 'NONE',  ( 0.000000000000000000, 0.000000000000000000, -1.000000000000000000 ) ) ;
#1115=CARTESIAN_POINT ( 'NONE',  ( -85.15643035625001289, -33.40312499938548285, -99.99999999999998579 ) ) ;
#1116=CARTESIAN_POINT ( 'NONE',  ( 85.15643035624999868, -35.05312499938548143, 98.40857419181659793 ) ) ;
#1117=CARTESIAN_POINT ( 'NONE',  ( 79.64356964374999848, -33.62812499938548427, -99.99999999999998579 ) ) ;
#1119=CARTESIAN_POINT ( 'NONE',  ( -83.77821517812500929, -32.31562499938548427, 102.3871387122750889 ) ) ;
#1120=CARTESIAN_POINT ( 'NONE',  ( 79.64356964374999848, -31.71562499938548285, -99.99999999999998579 ) ) ;
#1121=EDGE_CURVE ( 'NONE', #4832, #16118, #561, .T. ) ;
#1122=EDGE_LOOP ( 'NONE', ( #5152, #15546 ) ) ;
#1123=CARTESIAN_POINT ( 'NONE',  ( 81.02178482187500208, -35.05312499938548854, 97.61286128772489690 ) ) ;
#1128=CARTESIAN_POINT ( 'NONE',  ( -82.39999999999999147, -34.30312499938548143, 96.81714838363319586 ) ) ;
#1129=CARTESIAN_POINT ( 'NONE',  ( -79.64356964374999848, -31.26562499938548356, 99.99999999999998579 ) ) ;
#1131=CARTESIAN_POINT ( 'NONE',  ( -79.58826230849692251, -32.00000000000093792, -101.0460072438472139 ) ) ;
#1135=ADVANCED_FACE ( 'NONE', ( #13578 ), #13862, .F. ) ;
#1138=CARTESIAN_POINT ( 'NONE',  ( -83.90000000000000568, -34.96874999877096712, 97.40192378864668399 ) ) ;
#1140=CARTESIAN_POINT ( 'NONE',  ( 84.85729912020866550, -31.99999999999998579, 98.73859666561313020 ) ) ;
#1141=CARTESIAN_POINT ( 'NONE',  ( -82.39999999999999147, -33.20624999877097849, -102.9999999999999858 ) ) ;
#1143=AXIS2_PLACEMENT_3D ( 'NONE', #8341, #9245, #14297 ) ;
#1144=CARTESIAN_POINT ( 'NONE',  ( 82.40000000000000568, -30.00000000000000355, 103.0000000000000000 ) ) ;
#1145=DIRECTION ( 'NONE',  ( -1.000000000000000000, 0.000000000000000000, 0.000000000000000000 ) ) ;
#1146=CARTESIAN_POINT ( 'NONE',  ( 82.39999999999999147, -32.61562499938548854, -96.81714838363319586 ) ) ;
#1149=CARTESIAN_POINT ( 'NONE',  ( 80.90000000000000568, -33.39374999877097139, 97.40192378864668399 ) ) ;
#1151=FACE_OUTER_BOUND ( 'NONE', #13156, .T. ) ;
#1154=CARTESIAN_POINT ( 'NONE',  ( -84.06832524826180020, -35.00000000000001421, -97.74327260034003473 ) ) ;
#1156=EDGE_CURVE ( 'NONE', #7460, #2579, #7567, .T. ) ;
#1157=CARTESIAN_POINT ( 'NONE',  ( -85.15643035624999868, -34.22812499938547859, -101.5914258081833879 ) ) ;
#1161=CARTESIAN_POINT ( 'NONE',  ( -83.77821517812500929, -32.12812499938548427, -102.3871387122750889 ) ) ;
#1162=CARTESIAN_POINT ( 'NONE',  ( -79.39999999999999147, -32.38124999877096855, -101.7320508075688821 ) ) ;
#1163=DIRECTION ( 'NONE',  ( -0.000000000000000000, -0.000000000000000000, -1.000000000000000000 ) ) ;
#1165=VECTOR ( 'NONE', #12606, 1000.000000000000000 ) ;
#1168=CARTESIAN_POINT ( 'NONE',  ( -81.59615242270662350, -34.12634618820329990, -102.9999999999999858 ) ) ;
#1169=EDGE_CURVE ( 'NONE', #16799, #12847, #17295, .T. ) ;
#1170=CARTESIAN_POINT ( 'NONE',  ( 82.39999999999999147, -30.95624999877097139, -96.53589838486223584 ) ) ;
#1171=CIRCLE ( 'NONE', #2096, 2.199999999999993516 ) ;
#1173=ORIENTED_EDGE ( 'NONE', *, *, #12327, .F. ) ;
#1185=ORIENTED_EDGE ( 'NONE', *, *, #1121, .T. ) ;
#1186=( BOUNDED_CURVE ( )  B_SPLINE_CURVE ( 2, ( #8849, #13347, #16478, #11785, #17757, #4364, #13625, #6222, #12169, #7485, #16376, #3082, #169, #10324, #18137, #4757, #16666, #10700, #13440, #6026, #14805, #19320, #2985, #5931, #74, #11878, #3373, #14017, #16860, #12645, #7961, #5043, #3465, #9524, #2291, #3664, #10984, #17149, #15687, #3565, #15391, #746, #16953, #11186, #5137, #2002, #11082, #17052, #9628, #18233, #6315, #18619, #10892, #8160, #13915, #15590, #9423, #8062, #12269, #6408, #1904, #16757, #14109, #653, #12363, #553, #2102, #6701, #5237, #4950, #12549, #6511, #15289, #18331, #3756, #15490, #12456, #9325, #6601, #18520, #9721, #7866, #18422 ),
 .UNSPECIFIED., .F., .F. ) 
 B_SPLINE_CURVE_WITH_KNOTS ( ( 3, 2, 2, 2, 2, 2, 2, 2, 2, 2, 2, 2, 2, 2, 2, 2, 2, 2, 2, 2, 2, 2, 2, 2, 2, 2, 2, 2, 2, 2, 2, 2, 2, 2, 2, 2, 2, 2, 2, 2, 2, 3 ),
 ( 0.3495698921800953207, 0.3600184345287980592, 0.3750192026341646057, 0.3900199707395312076, 0.4050207388448978096, 0.4200215069502644116, 0.4350222750556309581, 0.4500230431609975601, 0.4650238112663641621, 0.4800245793717307086, 0.4950253474770972550, 0.5100261155824639125, 0.5250268836878304590, 0.5400276517931970055, 0.5550284198985635520, 0.5700291880039302095, 0.5850299561092967560, 0.6000307242146634135, 0.6150314923200299599, 0.6300322604253965064, 0.6450330285307630529, 0.6600337966361298214, 0.6750345647414962569, 0.6900353328468628034, 0.7050361009522294609, 0.7200368690575960073, 0.7350376371629625538, 0.7500384052683291003, 0.7650391733736958688, 0.7800399414790623043, 0.7950407095844289618, 0.8100414776897955083, 0.8250422457951620547, 0.8400430139005287122, 0.8550437820058951477, 0.8700445501112619162, 0.8850453182166284627, 0.9000460863219950092, 0.9150468544273615557, 0.9300476225327281021, 0.9450483906380946486, 0.9496006163947603440 ),
 .UNSPECIFIED. ) 
 CURVE ( )  GEOMETRIC_REPRESENTATION_ITEM ( )  RATIONAL_B_SPLINE_CURVE ( ( 0.9433623850486809737, 0.9066821623815489728, 1.000000000000000000, 0.8660254037844387076, 1.000000000000000000, 0.8660254037844387076, 1.000000000000000000, 0.8660254037844387076, 1.000000000000000000, 0.8660254037844387076, 1.000000000000000000, 0.8660254037844387076, 1.000000000000000000, 0.8660254037844387076, 1.000000000000000000, 0.8660254037844387076, 1.000000000000000000, 0.8660254037844387076, 1.000000000000000000, 0.8660254037844387076, 1.000000000000000000, 0.8660254037844387076, 1.000000000000000000, 0.8660254037844387076, 1.000000000000000000, 0.8660254037844387076, 1.000000000000000000, 0.8660254037844387076, 1.000000000000000000, 0.8660254037844387076, 1.000000000000000000, 0.8660254037844387076, 1.000000000000000000, 0.8660254037844387076, 1.000000000000000000, 0.8660254037844387076, 1.000000000000000000, 0.8660254037844387076, 1.000000000000000000, 0.8660254037844387076, 1.000000000000000000, 0.8660254037844387076, 1.000000000000000000, 0.8660254037844387076, 1.000000000000000000, 0.8660254037844387076, 1.000000000000000000, 0.8660254037844387076, 1.000000000000000000, 0.8660254037844387076, 1.000000000000000000, 0.8660254037844387076, 1.000000000000000000, 0.8660254037844387076, 1.000000000000000000, 0.8660254037844387076, 1.000000000000000000, 0.8660254037844387076, 1.000000000000000000, 0.8660254037844387076, 1.000000000000000000, 0.8660254037844387076, 1.000000000000000000, 0.8660254037844387076, 1.000000000000000000, 0.8660254037844387076, 1.000000000000000000, 0.8660254037844387076, 1.000000000000000000, 0.8660254037844387076, 1.000000000000000000, 0.8660254037844387076, 1.000000000000000000, 0.8660254037844387076, 1.000000000000000000, 0.8660254037844387076, 1.000000000000000000, 0.8660254037844387076, 1.000000000000000000, 0.8660254037844387076, 1.000000000000000000, 0.9593432414028746358, 0.9433623850486690943 ) ) 
 REPRESENTATION_ITEM ( '' )  );
#1188=CARTESIAN_POINT ( 'NONE',  ( 79.39999999999999147, -32.06250000000000000, -101.7320508075688537 ) ) ;
#1192=CARTESIAN_POINT ( 'NONE',  ( -81.02178482187500208, -31.00312499938548783, 102.3871387122750889 ) ) ;
#1195=CARTESIAN_POINT ( 'NONE',  ( 79.64057174634724845, -35.00000000000000000, 99.60353574117782216 ) ) ;
#1196=CARTESIAN_POINT ( 'NONE',  ( -85.15643035625001289, -34.64062499938548711, 99.99999999999998579 ) ) ;
#1199=CARTESIAN_POINT ( 'NONE',  ( -83.77821517812500929, -32.01562499938548001, -102.3871387122750889 ) ) ;
#1200=LINE ( 'NONE', #14466, #6177 ) ;
#1201=VECTOR ( 'NONE', #11469, 1000.000000000000000 ) ;
#1209=CARTESIAN_POINT ( 'NONE',  ( -82.40000000000000568, -30.00000000000000355, -99.99999999999998579 ) ) ;
#1210=CARTESIAN_POINT ( 'NONE',  ( 83.90000000000000568, -30.52500000000000213, 102.5980762113533018 ) ) ;
#1212=AXIS2_PLACEMENT_3D ( 'NONE', #4265, #4552, #19117 ) ;
#1216=CARTESIAN_POINT ( 'NONE',  ( -79.64356964374998427, -34.04062499938549280, -101.5914258081833879 ) ) ;
#1217=CARTESIAN_POINT ( 'NONE',  ( 82.39999999999999147, -34.52812499938548996, 96.81714838363319586 ) ) ;
#1218=CARTESIAN_POINT ( 'NONE',  ( 83.77821517812500929, -33.32812499938548711, -102.3871387122750889 ) ) ;
#1220=CARTESIAN_POINT ( 'NONE',  ( -79.64356964374998427, -32.65312499938548285, 101.5914258081833879 ) ) ;
#1221=CARTESIAN_POINT ( 'NONE',  ( 83.77821517812500929, -30.21562499938548285, -97.61286128772489690 ) ) ;
#1227=CARTESIAN_POINT ( 'NONE',  ( -85.15643035625001289, -33.74062499938548854, 99.99999999999998579 ) ) ;
#1228=VERTEX_POINT ( 'NONE', #12501 ) ;
#1229=CARTESIAN_POINT ( 'NONE',  ( -83.90000000000000568, -33.91874999877096997, 102.5980762113533018 ) ) ;
#1233=FACE_OUTER_BOUND ( 'NONE', #6066, .T. ) ;
#1234=EDGE_CURVE ( 'NONE', #13728, #11038, #3167, .T. ) ;
#1240=CARTESIAN_POINT ( 'NONE',  ( 79.64356964374999848, -33.62812499938548427, 99.99999999999998579 ) ) ;
#1243=CARTESIAN_POINT ( 'NONE',  ( 79.64356964374999848, -32.72812499938548569, -99.99999999999998579 ) ) ;
#1245=EDGE_LOOP ( 'NONE', ( #6037, #2189, #16909, #7995 ) ) ;
#1246=CARTESIAN_POINT ( 'NONE',  ( 83.90000000000000568, -32.56874999877096855, 97.40192378864668399 ) ) ;
#1250=( BOUNDED_CURVE ( )  B_SPLINE_CURVE ( 2, ( #13241, #10606, #2983, #8939, #5929 ),
 .UNSPECIFIED., .F., .F. ) 
 B_SPLINE_CURVE_WITH_KNOTS ( ( 3, 2, 3 ),
 ( 0.2975293541897477412, 0.3055555555555555802, 0.3125000000000001665 ),
 .UNSPECIFIED. ) 
 CURVE ( )  GEOMETRIC_REPRESENTATION_ITEM ( )  RATIONAL_B_SPLINE_CURVE ( ( 0.9346381638529939195, 0.9225778897267198353, 1.000000000000000000, 0.9330127018922177440, 0.9330127018922194093 ) ) 
 REPRESENTATION_ITEM ( '' )  );
#1252=DIRECTION ( 'NONE',  ( -1.000000000000000000, 0.000000000000000000, 0.000000000000000000 ) ) ;
#1253=CARTESIAN_POINT ( 'NONE',  ( -85.31192385480822793, -35.00000000000000711, -100.3932545473404048 ) ) ;
#1256=CARTESIAN_POINT ( 'NONE',  ( -82.39999999999999147, -32.95312499938548711, -103.1828516163667899 ) ) ;
#1258=CARTESIAN_POINT ( 'NONE',  ( -82.40000000000001990, -32.13750000000000284, -97.00000000000000000 ) ) ;
#1260=CARTESIAN_POINT ( 'NONE',  ( 81.02178482187500208, -34.90312499938548285, 102.3871387122750889 ) ) ;
#1261=CARTESIAN_POINT ( 'NONE',  ( -79.64356964375001269, -31.34062499938548640, -101.5914258081833879 ) ) ;
#1262=DIRECTION ( 'NONE',  ( 1.000000000000000000, 5.337610695313256118E-15, 0.000000000000000000 ) ) ;
#1263=CARTESIAN_POINT ( 'NONE',  ( -83.90000000000000568, -32.56874999877096855, -97.40192378864668399 ) ) ;
#1267=CARTESIAN_POINT ( 'NONE',  ( -79.64356964374998427, -32.20312499938548711, -98.40857419181659793 ) ) ;
#1268=CYLINDRICAL_SURFACE ( 'NONE', #15239, 2.199999999999993516 ) ;
#1270=CARTESIAN_POINT ( 'NONE',  ( 83.90000000000000568, -31.36874999877096926, -97.40192378864668399 ) ) ;
#1273=CARTESIAN_POINT ( 'NONE',  ( 82.39999999999999147, -34.52812499938548285, -103.1828516163667899 ) ) ;
#1280=CARTESIAN_POINT ( 'NONE',  ( -82.40000000000000568, -34.38749999999999574, -96.99999999999998579 ) ) ;
#1281=CARTESIAN_POINT ( 'NONE',  ( -79.83361526238435601, -35.00000000000000711, -98.97827398863965698 ) ) ;
#1284=EDGE_CURVE ( 'NONE', #5485, #5649, #1330, .T. ) ;
#1286=CARTESIAN_POINT ( 'NONE',  ( 83.90000000000000568, -34.87500000000000000, -102.5980762113533018 ) ) ;
#1287=ADVANCED_FACE ( 'NONE', ( #12410 ), #17276, .F. ) ;
#1289=CARTESIAN_POINT ( 'NONE',  ( -81.02178482187500208, -30.40312499938548640, 97.61286128772489690 ) ) ;
#1293=EDGE_CURVE ( 'NONE', #5861, #5491, #4553, .T. ) ;
#1294=CARTESIAN_POINT ( 'NONE',  ( 82.40000000000001990, -33.26250000000000284, -97.00000000000000000 ) ) ;
#1295=CARTESIAN_POINT ( 'NONE',  ( -79.64356964375001269, -34.90312499938548285, 101.5914258081833879 ) ) ;
#1298=CARTESIAN_POINT ( 'NONE',  ( -79.64356964375001269, -30.32812499938548711, -101.5914258081833879 ) ) ;
#1301=( BOUNDED_CURVE ( )  B_SPLINE_CURVE ( 2, ( #13801, #3645, #3352, #6585, #1987, #534, #9406, #18504, #2084 ),
 .UNSPECIFIED., .F., .F. ) 
 B_SPLINE_CURVE_WITH_KNOTS ( ( 3, 2, 2, 2, 3 ),
 ( 0.5625000000000000000, 0.5694444444444444198, 0.5833333333333333703, 0.5972222222222222099, 0.6041666666666666297 ),
 .UNSPECIFIED. ) 
 CURVE ( )  GEOMETRIC_REPRESENTATION_ITEM ( )  RATIONAL_B_SPLINE_CURVE ( ( 0.9330127018922194093, 0.9330127018922194093, 1.000000000000000000, 0.8660254037844387076, 1.000000000000000000, 0.8660254037844387076, 1.000000000000000000, 0.9330127018922198534, 0.9330127018922192983 ) ) 
 REPRESENTATION_ITEM ( '' )  );
#1306=ORIENTED_EDGE ( 'NONE', *, *, #10908, .F. ) ;
#1310=CARTESIAN_POINT ( 'NONE',  ( 83.20384757729335945, -32.28615380933863577, -97.00000000000000000 ) ) ;
#1311=CARTESIAN_POINT ( 'NONE',  ( 83.77821517812500929, -35.01562499938548711, 97.61286128772489690 ) ) ;
#1315=FACE_OUTER_BOUND ( 'NONE', #11332, .T. ) ;
#1316=CARTESIAN_POINT ( 'NONE',  ( 83.77821517812500929, -33.81562499938548427, 102.3871387122750889 ) ) ;
#1318=CARTESIAN_POINT ( 'NONE',  ( 83.77821517812500929, -31.56562499938548427, -97.61286128772489690 ) ) ;
#1320=CARTESIAN_POINT ( 'NONE',  ( -85.40000000000000568, -34.08749999999999858, 98.26794919243111792 ) ) ;
#1321=LINE ( 'NONE', #17248, #5381 ) ;
#1323=CARTESIAN_POINT ( 'NONE',  ( 79.64356964375001269, -34.49062499938548854, 101.5914258081833879 ) ) ;
#1324=CARTESIAN_POINT ( 'NONE',  ( 80.90000000000000568, -33.89999999999999858, -102.5980762113533018 ) ) ;
#1325=CARTESIAN_POINT ( 'NONE',  ( -82.39999999999999147, -32.95312499938548711, 96.81714838363319586 ) ) ;
#1330=CIRCLE ( 'NONE', #13493, 5.199999999999996625 ) ;
#1335=CARTESIAN_POINT ( 'NONE',  ( -82.40000000000001990, -33.26250000000000284, -103.0000000000000000 ) ) ;
#1336=CARTESIAN_POINT ( 'NONE',  ( -82.39999999999999147, -32.81250000000000000, -103.0000000000000000 ) ) ;
#1339=CARTESIAN_POINT ( 'NONE',  ( 81.02178482187500208, -33.70312499938548711, 97.61286128772489690 ) ) ;
#1340=CARTESIAN_POINT ( 'NONE',  ( -83.20384757729335945, -32.60759618943233562, 102.9999999999999858 ) ) ;
#1341=CARTESIAN_POINT ( 'NONE',  ( -81.59615242270662350, -32.56740381056766864, -97.00000000000000000 ) ) ;
#1342=CARTESIAN_POINT ( 'NONE',  ( 83.77821517812500929, -33.77812499938548285, -102.3871387122750889 ) ) ;
#1343=CARTESIAN_POINT ( 'NONE',  ( -85.15643035625001289, -32.05312499938548854, -99.99999999999998579 ) ) ;
#1345=ORIENTED_EDGE ( 'NONE', *, *, #5809, .T. ) ;
#1346=CARTESIAN_POINT ( 'NONE',  ( 82.39999999999999147, -33.20624999877097139, 103.4641016151377499 ) ) ;
#1350=EDGE_CURVE ( 'NONE', #4990, #15743, #6857, .T. ) ;
#1351=CARTESIAN_POINT ( 'NONE',  ( -79.64356964375001269, -30.44062499938548783, 98.40857419181659793 ) ) ;
#1354=CARTESIAN_POINT ( 'NONE',  ( -84.51155491706698797, -35.14114833091483803, -101.7717912238936719 ) ) ;
#1356=VERTEX_POINT ( 'NONE', #16575 ) ;
#1357=CARTESIAN_POINT ( 'NONE',  ( -79.64356964375001269, -34.49062499938548854, -101.5914258081833879 ) ) ;
#1359=CARTESIAN_POINT ( 'NONE',  ( -80.90000000000000568, -31.59374999877097423, -97.40192378864668399 ) ) ;
#1363=CARTESIAN_POINT ( 'NONE',  ( -79.64356964374998427, -34.37812499938548427, -101.5914258081833879 ) ) ;
#1366=FACE_OUTER_BOUND ( 'NONE', #1874, .T. ) ;
#1367=CARTESIAN_POINT ( 'NONE',  ( 79.39999999999999147, -31.93124999877096926, -98.26794919243110371 ) ) ;
#1369=( BOUNDED_CURVE ( )  B_SPLINE_CURVE ( 2, ( #8416, #19166, #3922, #2639, #4118, #10080, #12912, #5407, #14368 ),
 .UNSPECIFIED., .F., .F. ) 
 B_SPLINE_CURVE_WITH_KNOTS ( ( 3, 2, 2, 2, 3 ),
 ( 0.8541666666666665186, 0.8611111111111111605, 0.8750000000000000000, 0.8888888888888888395, 0.8958333333333333703 ),
 .UNSPECIFIED. ) 
 CURVE ( )  GEOMETRIC_REPRESENTATION_ITEM ( )  RATIONAL_B_SPLINE_CURVE ( ( 0.9330127018922194093, 0.9330127018922177440, 1.000000000000000000, 0.8660254037844387076, 1.000000000000000000, 0.8660254037844387076, 1.000000000000000000, 0.9330127018922187432, 0.9330127018922192983 ) ) 
 REPRESENTATION_ITEM ( '' )  );
#1371=CARTESIAN_POINT ( 'NONE',  ( 81.02178482187500208, -34.94062499938548427, -102.3871387122750889 ) ) ;
#1374=EDGE_CURVE ( 'NONE', #4798, #17054, #1186, .T. ) ;
#1378=CARTESIAN_POINT ( 'NONE',  ( -83.92761994969268358, -32.00000000000000000, 97.66884955414403180 ) ) ;
#1381=EDGE_LOOP ( 'NONE', ( #9993, #4042, #14838, #7130 ) ) ;
#1382=CARTESIAN_POINT ( 'NONE',  ( -82.32247963938031887, -35.00000000000000000, 102.7610832838413444 ) ) ;
#1383=CARTESIAN_POINT ( 'NONE',  ( 82.39999999999999147, -34.16250000000000142, -96.53589838486223584 ) ) ;
#1385=CARTESIAN_POINT ( 'NONE',  ( -79.64356964374999848, -34.07812499938548711, 99.99999999999998579 ) ) ;
#1392=SHAPE_REPRESENTATION_RELATIONSHIP ( 'NONE' , 'NONE' ,  #406, #5334 ) ;
#1393=CARTESIAN_POINT ( 'NONE',  ( -85.15643035624999868, -31.07812499938548356, -101.5914258081833879 ) ) ;
#1399=ORIENTED_EDGE ( 'NONE', *, *, #3870, .F. ) ;
#1401=EDGE_CURVE ( 'NONE', #15307, #16462, #2539, .T. ) ;
#1403=CARTESIAN_POINT ( 'NONE',  ( -85.40000000000000568, -32.15624999877096712, 101.7320508075688679 ) ) ;
#1404=CARTESIAN_POINT ( 'NONE',  ( 85.40000000000000568, -30.48749999999999716, 101.7320508075688679 ) ) ;
#1408=CARTESIAN_POINT ( 'NONE',  ( 85.15643035625001289, -34.19062499938548427, 99.99999999999998579 ) ) ;
#1409=CARTESIAN_POINT ( 'NONE',  ( 83.77821517812500929, -32.01562499938548001, -97.61286128772489690 ) ) ;
#1412=CARTESIAN_POINT ( 'NONE',  ( -85.15643035625001289, -34.64062499938548711, 99.99999999999998579 ) ) ;
#1413=CARTESIAN_POINT ( 'NONE',  ( 83.77821517812500929, -32.91562499938547859, -97.61286128772489690 ) ) ;
#1414=ORIENTED_EDGE ( 'NONE', *, *, #18431, .F. ) ;
#1415=DIRECTION ( 'NONE',  ( 0.000000000000000000, -1.000000000000000000, 0.000000000000000000 ) ) ;
#1416=CARTESIAN_POINT ( 'NONE',  ( -79.39999999999999147, -34.70624999877097139, 101.7320508075688537 ) ) ;
#1419=CARTESIAN_POINT ( 'NONE',  ( -79.64356964374999848, -33.06562499938548427, 99.99999999999998579 ) ) ;
#1421=CARTESIAN_POINT ( 'NONE',  ( -83.90000000000000568, -34.06874999877096855, 97.40192378864668399 ) ) ;
#1423=DIRECTION ( 'NONE',  ( 0.000000000000000000, -1.000000000000000000, 0.000000000000000000 ) ) ;
#1425=CARTESIAN_POINT ( 'NONE',  ( -82.40000000000001990, -32.08124999877097139, -97.00000000000000000 ) ) ;
#1428=CARTESIAN_POINT ( 'NONE',  ( 84.53225329756209305, -31.99999999999999289, 101.7559005160108256 ) ) ;
#1429=CARTESIAN_POINT ( 'NONE',  ( 79.64356964374999848, -31.82812499938548356, 99.99999999999998579 ) ) ;
#1430=DIRECTION ( 'NONE',  ( 0.000000000000000000, 1.000000000000000000, 0.000000000000000000 ) ) ;
#1431=CARTESIAN_POINT ( 'NONE',  ( -85.16931825408420309, -31.99999999999998579, -99.76128878215617135 ) ) ;
#1432=CARTESIAN_POINT ( 'NONE',  ( -83.77821517812500929, -30.32812499938548711, -102.3871387122750889 ) ) ;
#1433=ORIENTED_EDGE ( 'NONE', *, *, #7219, .F. ) ;
#1434=CARTESIAN_POINT ( 'NONE',  ( 85.40000000000000568, -34.48124999877096997, 101.7320508075688679 ) ) ;
#1435=DIRECTION ( 'NONE',  ( 0.000000000000000000, 0.000000000000000000, 1.000000000000000000 ) ) ;
#1437=CARTESIAN_POINT ( 'NONE',  ( -85.15643035624999868, -30.74062499938548143, 98.40857419181659793 ) ) ;
#1439=CARTESIAN_POINT ( 'NONE',  ( 79.68063642056725371, -32.00000000000002132, 101.2652131118146741 ) ) ;
#1440=ORIENTED_EDGE ( 'NONE', *, *, #15000, .F. ) ;
#1441=CARTESIAN_POINT ( 'NONE',  ( -83.77821517812500929, -34.26562499938548711, -102.3871387122750889 ) ) ;
#1443=FACE_OUTER_BOUND ( 'NONE', #7708, .T. ) ;
#1444=CARTESIAN_POINT ( 'NONE',  ( -79.64356964374999848, -32.72812499938548569, -99.99999999999998579 ) ) ;
#1447=CARTESIAN_POINT ( 'NONE',  ( -83.90000000000000568, -30.76874999877097139, -97.40192378864668399 ) ) ;
#1448=ADVANCED_FACE ( 'NONE', ( #2872 ), #1609, .F. ) ;
#1452=CARTESIAN_POINT ( 'NONE',  ( -85.15643035625001289, -34.67812499938548143, -101.5914258081833879 ) ) ;
#1453=CARTESIAN_POINT ( 'NONE',  ( 82.39999999999999147, -34.07812499938548711, 96.81714838363319586 ) ) ;
#1456=CARTESIAN_POINT ( 'NONE',  ( 83.90000000000000568, -34.06874999877096855, -97.40192378864668399 ) ) ;
#1459=CARTESIAN_POINT ( 'NONE',  ( 79.64356964374999848, -34.86562499938548143, -99.99999999999998579 ) ) ;
#1464=EDGE_LOOP ( 'NONE', ( #11747, #11309, #16868, #7244 ) ) ;
#1466=CARTESIAN_POINT ( 'NONE',  ( -79.39999999999999147, -34.27499999999999858, -99.99999999999998579 ) ) ;
#1469=ORIENTED_EDGE ( 'NONE', *, *, #10312, .F. ) ;
#1470=CARTESIAN_POINT ( 'NONE',  ( -83.03192786677307424, -35.00000000000000711, 102.6890373435400221 ) ) ;
#1473=CARTESIAN_POINT ( 'NONE',  ( -83.77821517812500929, -34.37812499938548427, 97.61286128772489690 ) ) ;
#1476=AXIS2_PLACEMENT_3D ( 'NONE', #15312, #674, #18638 ) ;
#1477=FACE_OUTER_BOUND ( 'NONE', #16511, .T. ) ;
#1478=( BOUNDED_CURVE ( )  B_SPLINE_CURVE ( 2, ( #3477, #13738, #4566, #16491, #6233, #7784, #6420, #1824, #1726 ),
 .UNSPECIFIED., .F., .F. ) 
 B_SPLINE_CURVE_WITH_KNOTS ( ( 3, 2, 2, 2, 3 ),
 ( 0.6041666666666666297, 0.6111111111111111605, 0.6250000000000000000, 0.6388888888888888395, 0.6458333333333333703 ),
 .UNSPECIFIED. ) 
 CURVE ( )  GEOMETRIC_REPRESENTATION_ITEM ( )  RATIONAL_B_SPLINE_CURVE ( ( 0.9330127018922192983, 0.9330127018922187432, 1.000000000000000000, 0.8660254037844387076, 1.000000000000000000, 0.8660254037844387076, 1.000000000000000000, 0.9330127018922187432, 0.9330127018922192983 ) ) 
 REPRESENTATION_ITEM ( '' )  );
#1479=EDGE_CURVE ( 'NONE', #16118, #14240, #2651, .T. ) ;
#1483=CARTESIAN_POINT ( 'NONE',  ( -85.40000000000000568, -34.48124999877096997, -101.7320508075688821 ) ) ;
#1484=EDGE_LOOP ( 'NONE', ( #2751, #15911, #9153, #14334 ) ) ;
#1485=AXIS2_PLACEMENT_3D ( 'NONE', #921, #15952, #5695 ) ;
#1487=CARTESIAN_POINT ( 'NONE',  ( -85.15643035625001289, -34.19062499938548427, -99.99999999999998579 ) ) ;
#1489=CARTESIAN_POINT ( 'NONE',  ( 96.99999999999994316, -29.80000000000000426, 150.0000000000000000 ) ) ;
#1494=VECTOR ( 'NONE', #15806, 1000.000000000000000 ) ;
#1495=MECHANICAL_DESIGN_GEOMETRIC_PRESENTATION_REPRESENTATION('',(#2115),#14585);
#1497=EDGE_CURVE ( 'NONE', #4468, #592, #11900, .T. ) ;
#1501=CARTESIAN_POINT ( 'NONE',  ( -79.39999999999999147, -32.41874999877096997, 99.99999999999998579 ) ) ;
#1502=CARTESIAN_POINT ( 'NONE',  ( 85.40000000000000568, -33.18750000000000000, 101.7320508075688679 ) ) ;
#1509=CARTESIAN_POINT ( 'NONE',  ( 79.64356964374999848, -30.36562499938548498, -99.99999999999998579 ) ) ;
#1513=CARTESIAN_POINT ( 'NONE',  ( 84.70388354820684640, -35.00002705695777649, -98.07851859032987818 ) ) ;
#1514=CARTESIAN_POINT ( 'NONE',  ( 85.15643035624999868, -33.25312499938548427, -101.5914258081833879 ) ) ;
#1518=CARTESIAN_POINT ( 'NONE',  ( 79.39999999999999147, -33.86250000000000426, -101.7320508075688537 ) ) ;
#1520=CARTESIAN_POINT ( 'NONE',  ( -83.77821517812500929, -34.56562499938548427, 102.3871387122750889 ) ) ;
#1523=AXIS2_PLACEMENT_3D ( 'NONE', #345, #18698, #6679 ) ;
#1525=CARTESIAN_POINT ( 'NONE',  ( 85.15643035625001289, -31.04062499938548569, 99.99999999999998579 ) ) ;
#1527=ADVANCED_FACE ( 'NONE', ( #7557 ), #13514, .F. ) ;
#1528=CARTESIAN_POINT ( 'NONE',  ( -99.99999999999998579, -5.200000000000000178, -150.0000000000000000 ) ) ;
#1529=CARTESIAN_POINT ( 'NONE',  ( -82.39999999999999147, -32.36250000000000426, 96.99999999999997158 ) ) ;
#1531=CARTESIAN_POINT ( 'NONE',  ( 85.03799702444359809, -32.00000000000000000, 100.8187845449565572 ) ) ;
#1532=CARTESIAN_POINT ( 'NONE',  ( 79.64356964375001269, -31.79062499938548569, 101.5914258081833879 ) ) ;
#1533=CARTESIAN_POINT ( 'NONE',  ( -82.40000000000000568, -30.00000000000000355, -96.99999999999998579 ) ) ;
#1534=EDGE_CURVE ( 'NONE', #3915, #18169, #9388, .T. ) ;
#1537=CARTESIAN_POINT ( 'NONE',  ( -81.02178482187500208, -30.40312499938548640, -102.3871387122750889 ) ) ;
#1540=CARTESIAN_POINT ( 'NONE',  ( 79.64356964374999848, -31.37812499938548427, 99.99999999999998579 ) ) ;
#1541=DIRECTION ( 'NONE',  ( -0.000000000000000000, -0.000000000000000000, -1.000000000000000000 ) ) ;
#1544=CARTESIAN_POINT ( 'NONE',  ( -79.64356964375001269, -31.86562499938548143, 101.5914258081833879 ) ) ;
#1545=LINE ( 'NONE', #16292, #10244 ) ;
#1547=CARTESIAN_POINT ( 'NONE',  ( -79.39999999999999147, -30.63750000000000284, -101.7320508075688821 ) ) ;
#1550=CARTESIAN_POINT ( 'NONE',  ( -81.02178482187500208, -32.20312499938548711, -102.3871387122750889 ) ) ;
#1551=CARTESIAN_POINT ( 'NONE',  ( 82.40000000000001990, -33.93750000000000711, 97.00000000000000000 ) ) ;
#1552=CARTESIAN_POINT ( 'NONE',  ( -80.90000000000000568, -32.34374999877096712, -102.5980762113533018 ) ) ;
#1557=CARTESIAN_POINT ( 'NONE',  ( 85.15643035625001289, -32.39062499938548711, 99.99999999999998579 ) ) ;
#1559=DIRECTION ( 'NONE',  ( -0.000000000000000000, -1.000000000000000000, -0.000000000000000000 ) ) ;
#1560=CARTESIAN_POINT ( 'NONE',  ( 79.39999999999999147, -34.63124999877096855, -98.26794919243110371 ) ) ;
#1568=ORIENTED_EDGE ( 'NONE', *, *, #568, .T. ) ;
#1569=ORIENTED_EDGE ( 'NONE', *, *, #6263, .T. ) ;
#1570=CARTESIAN_POINT ( 'NONE',  ( -81.59615242270662350, -34.36740381056766580, -96.99999999999998579 ) ) ;
#1572=CARTESIAN_POINT ( 'NONE',  ( -82.39999999999999147, -33.48750000000000426, -97.00000000000000000 ) ) ;
#1574=CARTESIAN_POINT ( 'NONE',  ( -99.99999999999998579, -35.00000000000000000, -150.0000000000000000 ) ) ;
#1576=CARTESIAN_POINT ( 'NONE',  ( -85.15643035624999868, -32.91562499938549280, 101.5914258081833879 ) ) ;
#1582=CARTESIAN_POINT ( 'NONE',  ( -83.20384757729337366, -34.35134618820330843, -97.00000000000000000 ) ) ;
#1584=CARTESIAN_POINT ( 'NONE',  ( -81.02178482187500208, -32.69062499938548427, -97.61286128772489690 ) ) ;
#1592=EDGE_CURVE ( 'NONE', #867, #14213, #19275, .T. ) ;
#1596=CARTESIAN_POINT ( 'NONE',  ( 99.99999999999994316, -32.00000000000000000, 150.0000000000000000 ) ) ;
#1598=CARTESIAN_POINT ( 'NONE',  ( -83.90000000000000568, -31.21874999877097068, 102.5980762113533018 ) ) ;
#1599=CARTESIAN_POINT ( 'NONE',  ( 79.39999999999999147, -32.06250000000000000, 98.26794919243113213 ) ) ;
#1603=CARTESIAN_POINT ( 'NONE',  ( 82.39999999999999147, -33.48750000000000426, -103.0000000000000000 ) ) ;
#1605=CARTESIAN_POINT ( 'NONE',  ( 79.64356964374999848, -32.16562499938548569, -99.99999999999998579 ) ) ;
#1609=CYLINDRICAL_SURFACE ( 'NONE', #8497, 3.000000000000002665 ) ;
#1610=CARTESIAN_POINT ( 'NONE',  ( 81.02178482187500208, -32.09062499938548285, -97.61286128772489690 ) ) ;
#1614=CARTESIAN_POINT ( 'NONE',  ( -79.39999999999999147, -31.53750000000000497, 98.26794919243110371 ) ) ;
#1617=CARTESIAN_POINT ( 'NONE',  ( -81.59615242270662350, -34.36740381056766580, 102.9999999999999858 ) ) ;
#1618=CARTESIAN_POINT ( 'NONE',  ( 83.20395887649176814, -35.00000000000001421, 97.36341917746361219 ) ) ;
#1620=CARTESIAN_POINT ( 'NONE',  ( -83.90000000000000568, -33.07500000000000284, -97.40192378864668399 ) ) ;
#1621=CARTESIAN_POINT ( 'NONE',  ( 99.99999999999997158, -5.200000000000008171, -150.0000000000000000 ) ) ;
#1622=CARTESIAN_POINT ( 'NONE',  ( 79.64356964375001269, -32.31562499938548427, 98.40857419181659793 ) ) ;
#1623=CARTESIAN_POINT ( 'NONE',  ( -82.39999999999999147, -32.58750000000000568, 102.9999999999999858 ) ) ;
#1626=CARTESIAN_POINT ( 'NONE',  ( -82.39999999999999147, -31.26562499938549067, -103.1828516163667899 ) ) ;
#1628=CARTESIAN_POINT ( 'NONE',  ( 81.02178482187500208, -30.85312499938548569, 102.3871387122750889 ) ) ;
#1629=CARTESIAN_POINT ( 'NONE',  ( 82.40000000000000568, -34.55624999877097281, 102.9999999999999858 ) ) ;
#1631=FACE_OUTER_BOUND ( 'NONE', #8929, .T. ) ;
#1633=CARTESIAN_POINT ( 'NONE',  ( -79.64356964374999848, -31.82812499938548356, 99.99999999999998579 ) ) ;
#1636=CARTESIAN_POINT ( 'NONE',  ( -79.39999999999999147, -30.26249999999999929, -98.26794919243113213 ) ) ;
#1638=CARTESIAN_POINT ( 'NONE',  ( 82.40000000000000568, -34.78124999877096712, -102.9999999999999858 ) ) ;
#1640=CARTESIAN_POINT ( 'NONE',  ( -81.02178482187500208, -34.15312499938548285, -97.61286128772489690 ) ) ;
#1645=CARTESIAN_POINT ( 'NONE',  ( -82.39999999999999147, -34.30312499938548143, -103.1828516163667899 ) ) ;
#1646=CARTESIAN_POINT ( 'NONE',  ( 81.02178482187500208, -32.54062499938548569, 102.3871387122750889 ) ) ;
#1650=CARTESIAN_POINT ( 'NONE',  ( 83.90000000000000568, -32.62500000000000000, -102.5980762113533018 ) ) ;
#1651=CARTESIAN_POINT ( 'NONE',  ( 85.40000000000000568, -34.03124999877096712, -98.26794919243111792 ) ) ;
#1653=ORIENTED_EDGE ( 'NONE', *, *, #6826, .T. ) ;
#1664=CARTESIAN_POINT ( 'NONE',  ( -83.20384757729337366, -33.50759618943233420, -97.00000000000000000 ) ) ;
#1668=CARTESIAN_POINT ( 'NONE',  ( -83.77821517812500929, -34.22812499938549280, 102.3871387122750889 ) ) ;
#1673=CARTESIAN_POINT ( 'NONE',  ( 82.40000000000000568, -30.00000000000000355, 96.99999999999998579 ) ) ;
#1674=CARTESIAN_POINT ( 'NONE',  ( -79.39999999999999147, -34.66874999877096997, -99.99999999999998579 ) ) ;
#1676=ORIENTED_EDGE ( 'NONE', *, *, #496, .T. ) ;
#1677=ADVANCED_FACE ( 'NONE', ( #16221, #14639 ), #1076, .F. ) ;
#1678=CARTESIAN_POINT ( 'NONE',  ( -79.64356964374999848, -34.41562499938548569, -99.99999999999998579 ) ) ;
#1682=CARTESIAN_POINT ( 'NONE',  ( 83.90000000000000568, -33.22500000000000142, -97.40192378864668399 ) ) ;
#1688=CARTESIAN_POINT ( 'NONE',  ( -79.39999999999999147, -31.48124999877097352, 98.26794919243110371 ) ) ;
#1689=CARTESIAN_POINT ( 'NONE',  ( 85.40000000000000568, -30.90000000000000213, 99.99999999999998579 ) ) ;
#1690=CARTESIAN_POINT ( 'NONE',  ( -81.68701737470176738, -31.99999999999998579, -97.18802777794499548 ) ) ;
#1692=CARTESIAN_POINT ( 'NONE',  ( 83.20384757729335945, -32.28615380933863577, 103.0000000000000000 ) ) ;
#1693=CARTESIAN_POINT ( 'NONE',  ( 80.80006050676068696, -31.99999999999999289, -97.54622936385604248 ) ) ;
#1694=CARTESIAN_POINT ( 'NONE',  ( 79.64356964374999848, -33.51562499938548711, -99.99999999999998579 ) ) ;
#1695=EDGE_LOOP ( 'NONE', ( #1173, #10213, #9283, #2397 ) ) ;
#1697=CARTESIAN_POINT ( 'NONE',  ( -82.39999999999999147, -34.52812499938548285, 103.1828516163667899 ) ) ;
#1698=CARTESIAN_POINT ( 'NONE',  ( 81.02178482187500208, -33.14062499938548711, -102.3871387122750889 ) ) ;
#1699=DIRECTION ( 'NONE',  ( 0.000000000000000000, 0.000000000000000000, 1.000000000000000000 ) ) ;
#1700=CARTESIAN_POINT ( 'NONE',  ( -79.39999999999999147, -34.66874999877096997, 99.99999999999998579 ) ) ;
#1702=CARTESIAN_POINT ( 'NONE',  ( -79.39999999999999147, -30.26249999999999929, 101.7320508075688537 ) ) ;
#1703=ORIENTED_EDGE ( 'NONE', *, *, #1293, .F. ) ;
#1711=CARTESIAN_POINT ( 'NONE',  ( 85.15643035624999868, -34.26562499938548711, 98.40857419181659793 ) ) ;
#1713=CARTESIAN_POINT ( 'NONE',  ( 79.64356964375001269, -30.51562499938548711, -101.5914258081833879 ) ) ;
#1715=CARTESIAN_POINT ( 'NONE',  ( 82.39999999999999147, -35.09062499938548285, -103.1828516163667899 ) ) ;
#1716=CARTESIAN_POINT ( 'NONE',  ( -85.15643035624999868, -34.26562499938548711, -98.40857419181659793 ) ) ;
#1717=VERTEX_POINT ( 'NONE', #8874 ) ;
#1718=CARTESIAN_POINT ( 'NONE',  ( 79.64356964375001269, -30.96562499938548640, 98.40857419181659793 ) ) ;
#1720=CARTESIAN_POINT ( 'NONE',  ( -85.15643035624999868, -31.11562499938548854, 101.5914258081833879 ) ) ;
#1722=ORIENTED_EDGE ( 'NONE', *, *, #10017, .T. ) ;
#1724=CARTESIAN_POINT ( 'NONE',  ( -83.90000000000000568, -31.87500000000000000, -102.5980762113533018 ) ) ;
#1726=CARTESIAN_POINT ( 'NONE',  ( 82.40000000000001990, -33.88124999877096855, 97.00000000000000000 ) ) ;
#1727=CARTESIAN_POINT ( 'NONE',  ( -82.39999999999999147, -34.19062499938548427, -96.81714838363319586 ) ) ;
#1734=CARTESIAN_POINT ( 'NONE',  ( -82.05869624310419397, -34.96883842999724124, -97.01420019955241969 ) ) ;
#1735=CARTESIAN_POINT ( 'NONE',  ( 83.77821517812500929, -32.31562499938548427, 97.61286128772489690 ) ) ;
#1736=CARTESIAN_POINT ( 'NONE',  ( 83.90000000000000568, -34.36874999877097281, -102.5980762113533018 ) ) ;
#1738=CARTESIAN_POINT ( 'NONE',  ( 82.39999999999999147, -32.58750000000000568, -102.9999999999999858 ) ) ;
#1739=CARTESIAN_POINT ( 'NONE',  ( 85.40000000000000568, -33.13124999877096855, -98.26794919243111792 ) ) ;
#1744=ADVANCED_FACE ( 'NONE', ( #9451 ), #5922, .F. ) ;
#1749=ORIENTED_EDGE ( 'NONE', *, *, #19047, .T. ) ;
#1751=VECTOR ( 'NONE', #13002, 1000.000000000000000 ) ;
#1752=FACE_OUTER_BOUND ( 'NONE', #19008, .T. ) ;
#1754=ORIENTED_EDGE ( 'NONE', *, *, #13096, .T. ) ;
#1757=CARTESIAN_POINT ( 'NONE',  ( -81.02178482187500208, -33.70312499938548711, 102.3871387122750889 ) ) ;
#1761=PLANE ( 'NONE',  #421 ) ;
#1762=CARTESIAN_POINT ( 'NONE',  ( 82.40000000000000568, -30.00000000000000355, 96.99999999999998579 ) ) ;
#1765=LINE ( 'NONE', #220, #18039 ) ;
#1768=CARTESIAN_POINT ( 'NONE',  ( -82.39999999999999147, -32.95312499938548711, -103.1828516163667899 ) ) ;
#1777=CARTESIAN_POINT ( 'NONE',  ( 82.39999999999999147, -33.20624999877097849, -97.00000000000000000 ) ) ;
#1778=CARTESIAN_POINT ( 'NONE',  ( 79.39999999999999147, -30.22500000000000142, -99.99999999999998579 ) ) ;
#1779=CARTESIAN_POINT ( 'NONE',  ( -85.40000000000000568, -32.23124999877096997, 98.26794919243111792 ) ) ;
#1780=CARTESIAN_POINT ( 'NONE',  ( 83.90000000000000568, -32.32500000000000284, 102.5980762113533018 ) ) ;
#1781=DIRECTION ( 'NONE',  ( -0.000000000000000000, -0.000000000000000000, -1.000000000000000000 ) ) ;
#1783=CARTESIAN_POINT ( 'NONE',  ( 82.39999999999999147, -32.84062499938548996, -103.1828516163667899 ) ) ;
#1784=VECTOR ( 'NONE', #18195, 1000.000000000000000 ) ;
#1786=CARTESIAN_POINT ( 'NONE',  ( 79.64356964375001269, -32.65312499938548285, -101.5914258081833879 ) ) ;
#1789=CARTESIAN_POINT ( 'NONE',  ( -82.40000000000001990, -34.16250000000000853, 97.00000000000000000 ) ) ;
#1790=CARTESIAN_POINT ( 'NONE',  ( 85.15643035624999868, -32.80312499938548854, -101.5914258081833879 ) ) ;
#1795=CARTESIAN_POINT ( 'NONE',  ( -83.77821517812500929, -35.01562499938548711, 102.3871387122750889 ) ) ;
#1796=EDGE_LOOP ( 'NONE', ( #14638, #7352, #14844, #15299 ) ) ;
#1799=CARTESIAN_POINT ( 'NONE',  ( 83.77821517812500929, -30.66562499938548569, 102.3871387122750889 ) ) ;
#1801=VECTOR ( 'NONE', #2887, 1000.000000000000000 ) ;
#1802=CARTESIAN_POINT ( 'NONE',  ( 84.97866794691725545, -31.99999999999998579, -99.01001922939877886 ) ) ;
#1804=CARTESIAN_POINT ( 'NONE',  ( -82.39999999999999147, -32.58750000000000568, 102.9999999999999858 ) ) ;
#1805=CARTESIAN_POINT ( 'NONE',  ( 84.51154815724953551, -35.25364861271051353, 101.7717992799616553 ) ) ;
#1806=CARTESIAN_POINT ( 'NONE',  ( 83.77821517812500929, -31.07812499938548711, -102.3871387122750889 ) ) ;
#1809=CARTESIAN_POINT ( 'NONE',  ( -84.97866794691721282, -32.00000000000001421, -100.9899807706014485 ) ) ;
#1810=CARTESIAN_POINT ( 'NONE',  ( -83.77821517812500929, -32.57812499938548711, -102.3871387122750889 ) ) ;
#1812=CARTESIAN_POINT ( 'NONE',  ( 80.90000000000000568, -35.19374999877096855, 97.40192378864668399 ) ) ;
#1817=CARTESIAN_POINT ( 'NONE',  ( -81.02178482187500208, -32.80312499938548854, 102.3871387122750889 ) ) ;
#1820=CARTESIAN_POINT ( 'NONE',  ( -83.90000000000000568, -32.17500000000000426, -97.40192378864668399 ) ) ;
#1823=CARTESIAN_POINT ( 'NONE',  ( 80.90000000000000568, -34.20000000000000284, -97.40192378864668399 ) ) ;
#1824=CARTESIAN_POINT ( 'NONE',  ( 81.59615242270665192, -33.86115380933864571, 97.00000000000000000 ) ) ;
#1825=CARTESIAN_POINT ( 'NONE',  ( -85.15643035624999868, -34.79062499938548569, -101.5914258081833879 ) ) ;
#1831=CARTESIAN_POINT ( 'NONE',  ( 83.20384757729337366, -32.34240381056766722, 103.0000000000000000 ) ) ;
#1832=CARTESIAN_POINT ( 'NONE',  ( 85.15643035625001289, -33.77812499938548285, 101.5914258081833879 ) ) ;
#1835=CARTESIAN_POINT ( 'NONE',  ( 80.90000000000000568, -34.14374999877097139, -97.40192378864668399 ) ) ;
#1842=EDGE_CURVE ( 'NONE', #5588, #19181, #14688, .T. ) ;
#1847=ORIENTED_EDGE ( 'NONE', *, *, #3268, .T. ) ;
#1848=CARTESIAN_POINT ( 'NONE',  ( -79.64356964375001269, -30.40312499938548285, -98.40857419181659793 ) ) ;
#1849=CARTESIAN_POINT ( 'NONE',  ( 96.99999999999997158, -5.200000000000003730, -150.0000000000000000 ) ) ;
#1851=ORIENTED_EDGE ( 'NONE', *, *, #12808, .F. ) ;
#1852=CARTESIAN_POINT ( 'NONE',  ( 84.44763168836732348, -32.00000000000002132, 98.15470523285560489 ) ) ;
#1853=CYLINDRICAL_SURFACE ( 'NONE', #11735, 2.199999999999993516 ) ;
#1854=LINE ( 'NONE', #16807, #16932 ) ;
#1865=CARTESIAN_POINT ( 'NONE',  ( -81.02178482187500208, -33.14062499938548711, -97.61286128772489690 ) ) ;
#1866=LINE ( 'NONE', #611, #2732 ) ;
#1867=EDGE_LOOP ( 'NONE', ( #1943, #15394, #2168, #4100 ) ) ;
#1868=ADVANCED_FACE ( 'NONE', ( #11479 ), #13038, .F. ) ;
#1870=CYLINDRICAL_SURFACE ( 'NONE', #16156, 3.000000000000002665 ) ;
#1871=CYLINDRICAL_SURFACE ( 'NONE', #4749, 3.000000000000002665 ) ;
#1872=DIRECTION ( 'NONE',  ( -0.000000000000000000, -1.000000000000000000, -0.000000000000000000 ) ) ;
#1873=ORIENTED_EDGE ( 'NONE', *, *, #18310, .F. ) ;
#1874=EDGE_LOOP ( 'NONE', ( #6386, #6158, #12245, #13159 ) ) ;
#1875=CARTESIAN_POINT ( 'NONE',  ( -99.99999999999998579, -29.80000000000000426, -150.0000000000000000 ) ) ;
#1876=CARTESIAN_POINT ( 'NONE',  ( 82.39999999999999147, -31.23750000000000071, -103.4641016151377499 ) ) ;
#1877=CARTESIAN_POINT ( 'NONE',  ( -83.90000000000000568, -34.36874999877097281, 102.5980762113533018 ) ) ;
#1881=CARTESIAN_POINT ( 'NONE',  ( 79.64356964374998427, -32.24062499938548854, -98.40857419181659793 ) ) ;
#1883=CARTESIAN_POINT ( 'NONE',  ( 82.39999999999999147, -33.40312499938548285, -96.81714838363319586 ) ) ;
#1885=B_SPLINE_CURVE_WITH_KNOTS ( 'NONE', 3,
 ( #9094, #13401, #18103, #33, #17906, #4512, #10468, #16434, #3043, #9005, #134, #13495, #3431, #14073, #9288, #12224 ),
 .UNSPECIFIED., .F., .F.,
 ( 4, 2, 2, 2, 2, 2, 2, 4 ),
 ( 0.000000000000000000, 0.0005391024520904479393, 0.001078204904180895879, 0.002156409808361764869, 0.002695512260452209014, 0.003234614712542652724, 0.003773717164633096869, 0.004312819616723541014 ),
 .UNSPECIFIED. ) ;
#1887=CARTESIAN_POINT ( 'NONE',  ( -85.40000000000000568, -34.91250000000000142, 101.7320508075688679 ) ) ;
#1888=B_SPLINE_CURVE_WITH_KNOTS ( 'NONE', 3,
 ( #7594, #16391, #19134, #13259, #10247, #13363, #17669, #91, #5751, #19233, #2385, #11991, #5849, #16209, #11700, #17772, #4379, #4474 ),
 .UNSPECIFIED., .F., .F.,
 ( 4, 2, 2, 2, 2, 2, 2, 2, 4 ),
 ( 0.000000000000000000, 0.0007089252359966202559, 0.001417850471993240512, 0.002126775707989860768, 0.002835700943986481024, 0.003544626179983101279, 0.004253551415979721535, 0.004962476651976341357, 0.005671401887972962047 ),
 .UNSPECIFIED. ) ;
#1893=CARTESIAN_POINT ( 'NONE',  ( -82.39999999999999147, -31.23750000000000071, 103.4641016151377499 ) ) ;
#1900=CARTESIAN_POINT ( 'NONE',  ( 82.39076102795759482, -31.99999999999997158, 97.13047754280712809 ) ) ;
#1901=CARTESIAN_POINT ( 'NONE',  ( 85.15643035624999868, -34.79062499938548569, 101.5914258081833879 ) ) ;
#1902=CARTESIAN_POINT ( 'NONE',  ( 79.64356964374999848, -31.82812499938548356, -99.99999999999998579 ) ) ;
#1904=CARTESIAN_POINT ( 'NONE',  ( -83.77821517812500929, -34.22812499938549280, 102.3871387122750889 ) ) ;
#1905=CARTESIAN_POINT ( 'NONE',  ( -85.15643035625001289, -33.40312499938548285, -99.99999999999998579 ) ) ;
#1907=CARTESIAN_POINT ( 'NONE',  ( 79.64356964375001269, -33.66562499938549280, 98.40857419181659793 ) ) ;
#1909=CARTESIAN_POINT ( 'NONE',  ( -85.15643035624999868, -35.16562499938547859, 101.5914258081833879 ) ) ;
#1911=CARTESIAN_POINT ( 'NONE',  ( 83.20384757729335945, -33.00134618820329990, 96.99999999999997158 ) ) ;
#1912=ORIENTED_EDGE ( 'NONE', *, *, #14250, .T. ) ;
#1913=CARTESIAN_POINT ( 'NONE',  ( -80.90000000000000568, -30.60000000000000142, -102.5980762113533018 ) ) ;
#1914=CARTESIAN_POINT ( 'NONE',  ( 79.39999999999999147, -34.31250000000000000, -101.7320508075688537 ) ) ;
#1916=CARTESIAN_POINT ( 'NONE',  ( -79.64356964375001269, -34.94062499938549138, -101.5914258081833879 ) ) ;
#1920=EDGE_LOOP ( 'NONE', ( #12424, #7805, #6513, #15193 ) ) ;
#1922=CARTESIAN_POINT ( 'NONE',  ( 83.20384757729335945, -34.40759618943233988, -102.9999999999999858 ) ) ;
#1926=CARTESIAN_POINT ( 'NONE',  ( 81.02178482187500208, -31.30312499938548498, -97.61286128772489690 ) ) ;
#1928=EDGE_CURVE ( 'NONE', #11038, #13093, #7368, .T. ) ;
#1931=ORIENTED_EDGE ( 'NONE', *, *, #704, .T. ) ;
#1937=CARTESIAN_POINT ( 'NONE',  ( -79.39999999999999147, -32.96250000000000568, -98.26794919243113213 ) ) ;
#1939=ORIENTED_EDGE ( 'NONE', *, *, #13900, .T. ) ;
#1942=CARTESIAN_POINT ( 'NONE',  ( -82.40000000000000568, -34.61250000000001137, 97.00000000000000000 ) ) ;
#1943=ORIENTED_EDGE ( 'NONE', *, *, #568, .F. ) ;
#1944=DIRECTION ( 'NONE',  ( 0.000000000000000000, 0.000000000000000000, 1.000000000000000000 ) ) ;
#1945=CARTESIAN_POINT ( 'NONE',  ( -85.40000000000000568, -33.50624999877096855, -98.26794919243111792 ) ) ;
#1957=ORIENTED_EDGE ( 'NONE', *, *, #1592, .T. ) ;
#1959=CARTESIAN_POINT ( 'NONE',  ( -85.15643035624999868, -34.67812499938548143, -101.5914258081833879 ) ) ;
#1962=ORIENTED_EDGE ( 'NONE', *, *, #11514, .F. ) ;
#1964=LINE ( 'NONE', #3430, #1165 ) ;
#1967=FACE_OUTER_BOUND ( 'NONE', #16196, .T. ) ;
#1969=DIRECTION ( 'NONE',  ( -0.000000000000000000, -1.000000000000000000, -0.000000000000000000 ) ) ;
#1972=CARTESIAN_POINT ( 'NONE',  ( 80.90000000000000568, -34.74374999877097281, 97.40192378864668399 ) ) ;
#1973=CARTESIAN_POINT ( 'NONE',  ( 79.39999999999999147, -30.71250000000000568, -101.7320508075688537 ) ) ;
#1974=CARTESIAN_POINT ( 'NONE',  ( -82.40000000000000568, -30.00000000000000355, -99.99999999999998579 ) ) ;
#1975=ADVANCED_FACE ( 'NONE', ( #12053 ), #14887, .F. ) ;
#1976=CARTESIAN_POINT ( 'NONE',  ( -82.39999999999999147, -33.65624999877096712, 96.53589838486223584 ) ) ;
#1977=CARTESIAN_POINT ( 'NONE',  ( 96.99999999999994316, -21.80000000000003268, -137.3499999999999943 ) ) ;
#1979=CARTESIAN_POINT ( 'NONE',  ( 79.64356964374999848, -32.72812499938548569, -99.99999999999998579 ) ) ;
#1980=CARTESIAN_POINT ( 'NONE',  ( -81.59615242270662350, -32.06115380933863435, -96.99999999999997158 ) ) ;
#1981=CARTESIAN_POINT ( 'NONE',  ( -83.77821517812500929, -33.66562499938548569, 102.3871387122750889 ) ) ;
#1982=CARTESIAN_POINT ( 'NONE',  ( 85.15643035624999868, -33.25312499938548427, -101.5914258081833879 ) ) ;
#1985=CARTESIAN_POINT ( 'NONE',  ( -79.39999999999999147, -33.37500000000000000, 99.99999999999998579 ) ) ;
#1986=( BOUNDED_CURVE ( )  B_SPLINE_CURVE ( 2, ( #1738, #15028, #1650, #10629, #16594, #9349, #14039, #8182, #6340 ),
 .UNSPECIFIED., .F., .F. ) 
 B_SPLINE_CURVE_WITH_KNOTS ( ( 3, 2, 2, 2, 3 ),
 ( 0.4791666666666666297, 0.4861111111111111049, 0.5000000000000000000, 0.5138888888888888395, 0.5208333333333333703 ),
 .UNSPECIFIED. ) 
 CURVE ( )  GEOMETRIC_REPRESENTATION_ITEM ( )  RATIONAL_B_SPLINE_CURVE ( ( 0.9330127018922194093, 0.9330127018922190762, 1.000000000000000000, 0.8660254037844387076, 1.000000000000000000, 0.8660254037844387076, 1.000000000000000000, 0.9330127018922187432, 0.9330127018922192983 ) ) 
 REPRESENTATION_ITEM ( '' )  );
#1987=CARTESIAN_POINT ( 'NONE',  ( 85.40000000000000568, -33.54374999877096286, -99.99999999999998579 ) ) ;
#1990=ADVANCED_FACE ( 'NONE', ( #6104 ), #55, .F. ) ;
#1992=CARTESIAN_POINT ( 'NONE',  ( -85.40000000000000568, -32.21249999999999858, 101.7320508075688679 ) ) ;
#1996=CARTESIAN_POINT ( 'NONE',  ( 83.77821517812500929, -32.91562499938547859, 102.3871387122750889 ) ) ;
#1997=CARTESIAN_POINT ( 'NONE',  ( 84.44763168836730927, -32.00000000000000711, -101.8452947671444093 ) ) ;
#1999=CARTESIAN_POINT ( 'NONE',  ( -85.15643035625001289, -32.09062499938548996, -101.5914258081833879 ) ) ;
#2000=CARTESIAN_POINT ( 'NONE',  ( 85.15643035625001289, -30.14062499938548711, 99.99999999999998579 ) ) ;
#2001=CARTESIAN_POINT ( 'NONE',  ( 82.39999999999999147, -31.04062499938548569, -103.1828516163667899 ) ) ;
#2002=CARTESIAN_POINT ( 'NONE',  ( -79.64356964374998427, -33.66562499938548569, 101.5914258081833879 ) ) ;
#2003=CARTESIAN_POINT ( 'NONE',  ( -81.02178482187500208, -34.60312499938549280, -97.61286128772489690 ) ) ;
#2005=CARTESIAN_POINT ( 'NONE',  ( 82.39999999999999147, -33.74062499938548854, 96.81714838363319586 ) ) ;
#2007=CARTESIAN_POINT ( 'NONE',  ( -79.64356964375001269, -30.40312499938548285, 101.5914258081833879 ) ) ;
#2008=CARTESIAN_POINT ( 'NONE',  ( -81.02178482187500208, -34.15312499938548285, 102.3871387122750889 ) ) ;
#2011=CARTESIAN_POINT ( 'NONE',  ( -85.40000000000000568, -32.73750000000000426, -101.7320508075688679 ) ) ;
#2017=ORIENTED_EDGE ( 'NONE', *, *, #1497, .F. ) ;
#2021=FACE_OUTER_BOUND ( 'NONE', #18994, .T. ) ;
#2022=CARTESIAN_POINT ( 'NONE',  ( -83.20384757729338787, -34.53615380933862866, 97.00000000000000000 ) ) ;
#2023=CARTESIAN_POINT ( 'NONE',  ( 83.77821517812500929, -32.57812499938548711, -97.61286128772489690 ) ) ;
#2025=AXIS2_PLACEMENT_3D ( 'NONE', #9054, #13641, #184 ) ;
#2027=( BOUNDED_CURVE ( )  B_SPLINE_CURVE ( 2, ( #6368, #16717, #14070, #4902, #16912, #6560, #12508, #18475, #5189 ),
 .UNSPECIFIED., .F., .F. ) 
 B_SPLINE_CURVE_WITH_KNOTS ( ( 3, 2, 2, 2, 3 ),
 ( 0.4374999999999999445, 0.4444444444444444198, 0.4583333333333333148, 0.4722222222222222099, 0.4791666666666666297 ),
 .UNSPECIFIED. ) 
 CURVE ( )  GEOMETRIC_REPRESENTATION_ITEM ( )  RATIONAL_B_SPLINE_CURVE ( ( 0.9330127018922192983, 0.9330127018922187432, 1.000000000000000000, 0.8660254037844387076, 1.000000000000000000, 0.8660254037844387076, 1.000000000000000000, 0.9330127018922196314, 0.9330127018922194093 ) ) 
 REPRESENTATION_ITEM ( '' )  );
#2028=CARTESIAN_POINT ( 'NONE',  ( 85.40000000000000568, -30.80624999877096926, 98.26794919243111792 ) ) ;
#2036=CARTESIAN_POINT ( 'NONE',  ( -79.64356964374999848, -30.81562499938548427, -99.99999999999998579 ) ) ;
#2041=CARTESIAN_POINT ( 'NONE',  ( 79.64356964374998427, -32.31562499938548427, 98.40857419181659793 ) ) ;
#2042=CARTESIAN_POINT ( 'NONE',  ( -79.39999999999999147, -33.73124999877096997, -101.7320508075688821 ) ) ;
#2044=CARTESIAN_POINT ( 'NONE',  ( -82.65333140691201663, -34.99995246259153703, 97.01071553687880566 ) ) ;
#2047=CARTESIAN_POINT ( 'NONE',  ( 83.43443729601675329, -34.99999999999999289, -102.5775038898419496 ) ) ;
#2060=ORIENTED_EDGE ( 'NONE', *, *, #1928, .T. ) ;
#2062=ADVANCED_FACE ( 'NONE', ( #16556 ), #16458, .F. ) ;
#2063=ORIENTED_EDGE ( 'NONE', *, *, #17735, .T. ) ;
#2064=ORIENTED_EDGE ( 'NONE', *, *, #8892, .T. ) ;
#2066=CARTESIAN_POINT ( 'NONE',  ( 81.02178482187500208, -34.49062499938548854, -102.3871387122750889 ) ) ;
#2067=CARTESIAN_POINT ( 'NONE',  ( -79.64356964374998427, -34.94062499938548427, -101.5914258081833879 ) ) ;
#2069=ADVANCED_FACE ( 'NONE', ( #3157 ), #11955, .T. ) ;
#2070=CARTESIAN_POINT ( 'NONE',  ( -85.40000000000000568, -34.03124999877096712, 98.26794919243111792 ) ) ;
#2072=CARTESIAN_POINT ( 'NONE',  ( -79.39999999999999147, -33.28124999877096712, 98.26794919243110371 ) ) ;
#2074=CIRCLE ( 'NONE', #1143, 3.000000000000002665 ) ;
#2075=CARTESIAN_POINT ( 'NONE',  ( 79.64356964374998427, -33.21562499938548996, -101.5914258081833879 ) ) ;
#2076=CARTESIAN_POINT ( 'NONE',  ( 82.40000000000000568, -33.93750000000000711, 97.00000000000000000 ) ) ;
#2077=CARTESIAN_POINT ( 'NONE',  ( -83.77821517812500929, -32.01562499938548001, 97.61286128772489690 ) ) ;
#2078=CARTESIAN_POINT ( 'NONE',  ( 81.02178482187500208, -33.44062499938548427, -97.61286128772489690 ) ) ;
#2081=CARTESIAN_POINT ( 'NONE',  ( -79.39999999999999147, -33.33749999999999858, 98.26794919243110371 ) ) ;
#2082=CARTESIAN_POINT ( 'NONE',  ( -83.90000000000000568, -31.21874999877097068, -97.40192378864668399 ) ) ;
#2083=ADVANCED_FACE ( 'NONE', ( #19301 ), #6298, .F. ) ;
#2084=CARTESIAN_POINT ( 'NONE',  ( 82.39999999999999147, -33.65624999877097423, -97.00000000000000000 ) ) ;
#2089=CARTESIAN_POINT ( 'NONE',  ( -80.90000000000000568, -31.94999999999999929, 97.40192378864668399 ) ) ;
#2092=CARTESIAN_POINT ( 'NONE',  ( 82.39999999999999147, -33.17812499938548854, 96.81714838363319586 ) ) ;
#2093=AXIS2_PLACEMENT_3D ( 'NONE', #15295, #8948, #3277 ) ;
#2096=AXIS2_PLACEMENT_3D ( 'NONE', #13867, #12506, #8011 ) ;
#2098=CARTESIAN_POINT ( 'NONE',  ( 85.15643035625001289, -31.49062499938548498, 99.99999999999998579 ) ) ;
#2099=( BOUNDED_CURVE ( )  B_SPLINE_CURVE ( 2, ( #18299, #626, #17023, #12431, #18693, #6574, #14179, #12522, #12619 ),
 .UNSPECIFIED., .F., .F. ) 
 B_SPLINE_CURVE_WITH_KNOTS ( ( 3, 2, 2, 2, 3 ),
 ( 0.3958333333333334259, 0.4027777777777777901, 0.4166666666666666852, 0.4305555555555555802, 0.4375000000000000555 ),
 .UNSPECIFIED. ) 
 CURVE ( )  GEOMETRIC_REPRESENTATION_ITEM ( )  RATIONAL_B_SPLINE_CURVE ( ( 0.9330127018922192983, 0.9330127018922200755, 1.000000000000000000, 0.8660254037844387076, 1.000000000000000000, 0.8660254037844387076, 1.000000000000000000, 0.9330127018922187432, 0.9330127018922192983 ) ) 
 REPRESENTATION_ITEM ( '' )  );
#2100=CARTESIAN_POINT ( 'NONE',  ( 83.77821517812500929, -31.97812499938548925, -102.3871387122750889 ) ) ;
#2102=CARTESIAN_POINT ( 'NONE',  ( -81.02178482187500208, -34.45312499938548711, 97.61286128772489690 ) ) ;
#2103=CARTESIAN_POINT ( 'NONE',  ( -85.15643035624999868, -32.91562499938549280, -98.40857419181659793 ) ) ;
#2104=ORIENTED_EDGE ( 'NONE', *, *, #12723, .T. ) ;
#2105=CARTESIAN_POINT ( 'NONE',  ( 81.02178482187500208, -33.10312499938548569, 102.3871387122750889 ) ) ;
#2108=CARTESIAN_POINT ( 'NONE',  ( -82.39999999999999147, -31.60312499938548569, 96.81714838363319586 ) ) ;
#2109=CARTESIAN_POINT ( 'NONE',  ( -79.64356964375001269, -33.14062499938548711, 98.40857419181659793 ) ) ;
#2111=EDGE_LOOP ( 'NONE', ( #18672, #110, #18684, #7941 ) ) ;
#2113=CARTESIAN_POINT ( 'NONE',  ( -79.39999999999999147, -33.41250000000000142, -98.26794919243113213 ) ) ;
#2115=STYLED_ITEM ( 'NONE', ( #2752 ), #5334 ) ;
#2117=CARTESIAN_POINT ( 'NONE',  ( 84.70388354820684640, -35.00002705695777649, -98.07851859032987818 ) ) ;
#2118=CARTESIAN_POINT ( 'NONE',  ( -85.15643035625001289, -35.20312499938548711, -99.99999999999998579 ) ) ;
#2122=ORIENTED_EDGE ( 'NONE', *, *, #2958, .F. ) ;
#2123=EDGE_CURVE ( 'NONE', #3130, #11060, #14746, .T. ) ;
#2124=DIRECTION ( 'NONE',  ( 0.000000000000000000, 0.000000000000000000, 1.000000000000000000 ) ) ;
#2128=DIRECTION ( 'NONE',  ( -0.000000000000000000, -1.000000000000000000, -0.000000000000000000 ) ) ;
#2129=CARTESIAN_POINT ( 'NONE',  ( 81.02178482187500208, -30.40312499938548640, -97.61286128772489690 ) ) ;
#2130=VECTOR ( 'NONE', #16619, 1000.000000000000000 ) ;
#2134=CARTESIAN_POINT ( 'NONE',  ( 83.90000000000000568, -30.46874999877096712, 102.5980762113533018 ) ) ;
#2139=CARTESIAN_POINT ( 'NONE',  ( -82.39999999999999147, -34.83749999999999858, 103.0000000000000000 ) ) ;
#2142=CARTESIAN_POINT ( 'NONE',  ( -82.39999999999999147, -32.05312499938548854, -103.1828516163667899 ) ) ;
#2143=CARTESIAN_POINT ( 'NONE',  ( -79.39999999999999147, -33.80624999877097281, -98.26794919243113213 ) ) ;
#2144=ORIENTED_EDGE ( 'NONE', *, *, #15355, .F. ) ;
#2145=CARTESIAN_POINT ( 'NONE',  ( 85.15643035625001289, -34.71562499938548285, 98.40857419181659793 ) ) ;
#2146=CARTESIAN_POINT ( 'NONE',  ( -82.39999999999999147, -34.10624999877096997, -103.4641016151377499 ) ) ;
#2147=VECTOR ( 'NONE', #5552, 1000.000000000000000 ) ;
#2148=CARTESIAN_POINT ( 'NONE',  ( 79.39999999999999147, -31.08750000000000213, 101.7320508075688821 ) ) ;
#2152=CARTESIAN_POINT ( 'NONE',  ( 85.24876232368839624, -34.99999999999999289, -100.5466586069351393 ) ) ;
#2156=ORIENTED_EDGE ( 'NONE', *, *, #4800, .T. ) ;
#2157=CARTESIAN_POINT ( 'NONE',  ( -83.90000000000000568, -34.12500000000000000, 97.40192378864668399 ) ) ;
#2160=( BOUNDED_CURVE ( )  B_SPLINE_CURVE ( 2, ( #12955, #13054, #18926, #3773, #11495, #19020, #4070, #17459, #14221 ),
 .UNSPECIFIED., .F., .F. ) 
 B_SPLINE_CURVE_WITH_KNOTS ( ( 3, 2, 2, 2, 3 ),
 ( 0.5208333333333334814, 0.5277777777777777901, 0.5416666666666666297, 0.5555555555555555802, 0.5625000000000000000 ),
 .UNSPECIFIED. ) 
 CURVE ( )  GEOMETRIC_REPRESENTATION_ITEM ( )  RATIONAL_B_SPLINE_CURVE ( ( 0.9330127018922194093, 0.9330127018922209636, 1.000000000000000000, 0.8660254037844387076, 1.000000000000000000, 0.8660254037844387076, 1.000000000000000000, 0.9330127018922194093, 0.9330127018922194093 ) ) 
 REPRESENTATION_ITEM ( '' )  );
#2161=ORIENTED_EDGE ( 'NONE', *, *, #5204, .F. ) ;
#2165=ORIENTED_EDGE ( 'NONE', *, *, #8055, .F. ) ;
#2166=DIRECTION ( 'NONE',  ( 0.000000000000000000, 1.000000000000000000, 0.000000000000000000 ) ) ;
#2168=ORIENTED_EDGE ( 'NONE', *, *, #14963, .T. ) ;
#2170=CARTESIAN_POINT ( 'NONE',  ( 85.15643035624999868, -35.05312499938548143, -101.5914258081833879 ) ) ;
#2172=CARTESIAN_POINT ( 'NONE',  ( -79.39999999999999147, -35.11874999877096570, 99.99999999999998579 ) ) ;
#2176=CARTESIAN_POINT ( 'NONE',  ( 85.15643035625001289, -32.02817623523065294, -101.0587761908874569 ) ) ;
#2177=CARTESIAN_POINT ( 'NONE',  ( 79.39999999999999147, -33.82500000000000284, 99.99999999999998579 ) ) ;
#2178=CARTESIAN_POINT ( 'NONE',  ( -82.39999999999999147, -34.30312499938548143, 96.81714838363319586 ) ) ;
#2180=ORIENTED_EDGE ( 'NONE', *, *, #14586, .T. ) ;
#2181=CARTESIAN_POINT ( 'NONE',  ( -83.90000000000000568, -34.12500000000000000, 97.40192378864668399 ) ) ;
#2188=CARTESIAN_POINT ( 'NONE',  ( -83.90000000000000568, -32.17500000000000426, 102.5980762113533018 ) ) ;
#2189=ORIENTED_EDGE ( 'NONE', *, *, #13529, .F. ) ;
#2192=CARTESIAN_POINT ( 'NONE',  ( 79.64356964374999848, -31.71562499938548285, 99.99999999999998579 ) ) ;
#2193=ADVANCED_FACE ( 'NONE', ( #826 ), #4930, .F. ) ;
#2195=CARTESIAN_POINT ( 'NONE',  ( 81.01744233620654256, -32.00000000000000000, 97.41649131116879801 ) ) ;
#2196=CARTESIAN_POINT ( 'NONE',  ( 85.15643035625001289, -32.39062499938548711, 99.99999999999998579 ) ) ;
#2197=CARTESIAN_POINT ( 'NONE',  ( 83.77821517812500929, -30.62812499938548783, -102.3871387122750889 ) ) ;
#2199=CARTESIAN_POINT ( 'NONE',  ( -83.77821517812500929, -30.66562499938548569, -102.3871387122750889 ) ) ;
#2201=ORIENTED_EDGE ( 'NONE', *, *, #3547, .T. ) ;
#2202=CARTESIAN_POINT ( 'NONE',  ( 83.77821517812500929, -33.32812499938548711, 97.61286128772489690 ) ) ;
#2204=CARTESIAN_POINT ( 'NONE',  ( -82.39999999999999147, -32.05312499938548854, 96.81714838363319586 ) ) ;
#2205=CARTESIAN_POINT ( 'NONE',  ( -84.51154815724953551, -35.25364861271051353, 98.22820072003833047 ) ) ;
#2206=DIRECTION ( 'NONE',  ( -0.000000000000000000, -1.000000000000000000, -0.000000000000000000 ) ) ;
#2207=VERTEX_POINT ( 'NONE', #18407 ) ;
#2208=CARTESIAN_POINT ( 'NONE',  ( -80.90000000000000568, -34.35000000000000853, -97.40192378864668399 ) ) ;
#2211=CARTESIAN_POINT ( 'NONE',  ( -82.39999999999999147, -35.09062499938548285, -96.81714838363319586 ) ) ;
#2216=LINE ( 'NONE', #15507, #18193 ) ;
#2217=CARTESIAN_POINT ( 'NONE',  ( -85.40000000000000568, -33.05624999877097281, -98.26794919243111792 ) ) ;
#2218=CARTESIAN_POINT ( 'NONE',  ( 82.39999999999999147, -31.49062499938548854, -103.1828516163667899 ) ) ;
#2219=CARTESIAN_POINT ( 'NONE',  ( 80.90000000000000568, -34.64999999999999858, 102.5980762113533018 ) ) ;
#2225=B_SPLINE_CURVE_WITH_KNOTS ( 'NONE', 3,
 ( #19, #17794, #16324, #5873, #11825, #2837, #7425, #8791, #2933, #14749, #8886, #1382, #14949, #14845, #1470, #13385 ),
 .UNSPECIFIED., .F., .F.,
 ( 4, 2, 2, 2, 2, 2, 2, 4 ),
 ( 0.000000000000000000, 0.0005391024520904520593, 0.001078204904180904119, 0.002156409808361781782, 0.002695512260452248912, 0.003234614712542715608, 0.003773717164633182304, 0.004312819616723649434 ),
 .UNSPECIFIED. ) ;
#2227=CARTESIAN_POINT ( 'NONE',  ( -84.75088379146902184, -34.99999999999999289, -98.39201219457972059 ) ) ;
#2228=ORIENTED_EDGE ( 'NONE', *, *, #6672, .F. ) ;
#2231=CARTESIAN_POINT ( 'NONE',  ( -83.77821517812500929, -30.66562499938548569, -102.3871387122750889 ) ) ;
#2233=CARTESIAN_POINT ( 'NONE',  ( 79.64356964374999848, -33.17812499938548854, 99.99999999999998579 ) ) ;
#2234=CARTESIAN_POINT ( 'NONE',  ( -82.39999999999999147, -33.43124999877097281, -96.53589838486223584 ) ) ;
#2236=DIRECTION ( 'NONE',  ( 0.000000000000000000, -1.000000000000000000, 0.000000000000000000 ) ) ;
#2241=CARTESIAN_POINT ( 'NONE',  ( -80.90000000000000568, -34.14374999877097139, 97.40192378864668399 ) ) ;
#2243=ORIENTED_EDGE ( 'NONE', *, *, #6057, .T. ) ;
#2244=EDGE_CURVE ( 'NONE', #5317, #1228, #1301, .T. ) ;
#2245=CARTESIAN_POINT ( 'NONE',  ( 81.02178482187500208, -33.59062499938548285, -102.3871387122750889 ) ) ;
#2247=DIRECTION ( 'NONE',  ( 0.000000000000000000, 0.000000000000000000, 1.000000000000000000 ) ) ;
#2248=ORIENTED_EDGE ( 'NONE', *, *, #14234, .F. ) ;
#2253=CARTESIAN_POINT ( 'NONE',  ( 96.99999999999994316, -21.80000000000003268, -139.9999999999999716 ) ) ;
#2254=AXIS2_PLACEMENT_3D ( 'NONE', #5055, #18531, #14119 ) ;
#2256=VERTEX_POINT ( 'NONE', #12439 ) ;
#2258=CARTESIAN_POINT ( 'NONE',  ( 79.39999999999999147, -32.51250000000000284, -101.7320508075688537 ) ) ;
#2260=CARTESIAN_POINT ( 'NONE',  ( -85.40000000000000568, -33.99374999877097281, 99.99999999999998579 ) ) ;
#2267=CARTESIAN_POINT ( 'NONE',  ( -85.15643035624999868, -32.87812499938549138, 98.40857419181659793 ) ) ;
#2271=CARTESIAN_POINT ( 'NONE',  ( 84.51154815724953551, -35.14114861271051637, -98.22820072003833047 ) ) ;
#2274=CARTESIAN_POINT ( 'NONE',  ( -79.39999999999999147, -34.27499999999999858, 99.99999999999998579 ) ) ;
#2281=AXIS2_PLACEMENT_3D ( 'NONE', #15257, #6282, #6184 ) ;
#2283=CARTESIAN_POINT ( 'NONE',  ( 79.64356964375001269, -33.47812499938547859, 101.5914258081833879 ) ) ;
#2287=DIRECTION ( 'NONE',  ( -0.000000000000000000, -0.000000000000000000, -1.000000000000000000 ) ) ;
#2288=CARTESIAN_POINT ( 'NONE',  ( 82.39999999999999147, -32.50312499938548427, 103.1828516163667899 ) ) ;
#2289=CARTESIAN_POINT ( 'NONE',  ( 85.15643035625001289, -34.75312499938548427, -99.99999999999998579 ) ) ;
#2291=CARTESIAN_POINT ( 'NONE',  ( -81.02178482187500208, -33.25312499938548427, 102.3871387122750889 ) ) ;
#2292=VERTEX_POINT ( 'NONE', #5027 ) ;
#2293=CARTESIAN_POINT ( 'NONE',  ( 85.15643035624999868, -32.54062499938548569, 101.5914258081833879 ) ) ;
#2296=CARTESIAN_POINT ( 'NONE',  ( -82.39999999999999147, -30.47812499938548569, 103.1828516163667899 ) ) ;
#2297=CARTESIAN_POINT ( 'NONE',  ( -82.39999999999999147, -33.29062499938549280, 103.1828516163667899 ) ) ;
#2299=VERTEX_POINT ( 'NONE', #11065 ) ;
#2300=CARTESIAN_POINT ( 'NONE',  ( -83.90000000000000568, -32.62500000000000000, -97.40192378864668399 ) ) ;
#2306=CARTESIAN_POINT ( 'NONE',  ( -82.40000000000001990, -32.75624999877096855, 97.00000000000000000 ) ) ;
#2308=CARTESIAN_POINT ( 'NONE',  ( 79.64356964374998427, -34.90312499938548285, 98.40857419181659793 ) ) ;
#2309=CARTESIAN_POINT ( 'NONE',  ( 81.02178482187500208, -30.55312499938548854, 97.61286128772489690 ) ) ;
#2312=CARTESIAN_POINT ( 'NONE',  ( 83.77821517812500929, -32.12812499938548427, -97.61286128772489690 ) ) ;
#2313=CARTESIAN_POINT ( 'NONE',  ( -83.20384757729333103, -33.18615380933863435, 96.99999999999997158 ) ) ;
#2314=ORIENTED_EDGE ( 'NONE', *, *, #16158, .T. ) ;
#2315=CARTESIAN_POINT ( 'NONE',  ( 85.40000000000000568, -30.39374999877097139, 99.99999999999998579 ) ) ;
#2322=CARTESIAN_POINT ( 'NONE',  ( 83.90000000000000568, -33.97500000000000853, 97.40192378864668399 ) ) ;
#2324=CARTESIAN_POINT ( 'NONE',  ( -81.02178482187500208, -32.69062499938548427, -97.61286128772489690 ) ) ;
#2326=DIRECTION ( 'NONE',  ( 1.000000000000000000, -1.577021341797101948E-15, 0.000000000000000000 ) ) ;
#2328=CARTESIAN_POINT ( 'NONE',  ( 79.64356964374998427, -34.04062499938549280, 101.5914258081833879 ) ) ;
#2329=CARTESIAN_POINT ( 'NONE',  ( -85.40000000000000568, -35.30624999877096570, -98.26794919243111792 ) ) ;
#2330=CARTESIAN_POINT ( 'NONE',  ( 79.39999999999999147, -33.86250000000000426, 98.26794919243113213 ) ) ;
#2337=ADVANCED_FACE ( 'NONE', ( #17324 ), #13017, .F. ) ;
#2338=DIRECTION ( 'NONE',  ( -0.000000000000000000, -0.000000000000000000, -1.000000000000000000 ) ) ;
#2340=ORIENTED_EDGE ( 'NONE', *, *, #18683, .F. ) ;
#2341=CARTESIAN_POINT ( 'NONE',  ( 82.39999999999999147, -32.72812499938548569, -103.1828516163667899 ) ) ;
#2345=ORIENTED_EDGE ( 'NONE', *, *, #2657, .F. ) ;
#2346=CARTESIAN_POINT ( 'NONE',  ( 85.40000000000000568, -32.70000000000000284, 99.99999999999998579 ) ) ;
#2350=CIRCLE ( 'NONE', #12947, 2.199999999999993516 ) ;
#2352=ORIENTED_EDGE ( 'NONE', *, *, #10186, .F. ) ;
#2353=CARTESIAN_POINT ( 'NONE',  ( 79.39999999999999147, -33.82500000000000284, -99.99999999999998579 ) ) ;
#2355=CARTESIAN_POINT ( 'NONE',  ( 82.40000000000000568, -30.00000000000000355, -99.99999999999998579 ) ) ;
#2356=CARTESIAN_POINT ( 'NONE',  ( -83.77821517812500929, -31.52812499938548996, 102.3871387122750889 ) ) ;
#2358=CARTESIAN_POINT ( 'NONE',  ( -81.59615242270662350, -33.41115380933863577, 102.9999999999999858 ) ) ;
#2360=CARTESIAN_POINT ( 'NONE',  ( 83.20384757729335945, -33.90134618820329848, 96.99999999999998579 ) ) ;
#2363=CARTESIAN_POINT ( 'NONE',  ( -85.15643035624999868, -32.80312499938548854, 101.5914258081833879 ) ) ;
#2365=CARTESIAN_POINT ( 'NONE',  ( 82.40000000000000568, -30.00000000000000355, 96.99999999999998579 ) ) ;
#2366=ORIENTED_EDGE ( 'NONE', *, *, #2123, .F. ) ;
#2369=B_SPLINE_CURVE_WITH_KNOTS ( 'NONE', 3,
 ( #14521, #8285, #14236, #1154, #7113, #18750, #2227, #2422, #8382, #971, #12874, #11885, #1253, #17662, #9050, #7588, #10139, #6036 ),
 .UNSPECIFIED., .F., .F.,
 ( 4, 2, 2, 2, 2, 2, 2, 2, 4 ),
 ( 0.000000000000000000, 0.0007089252359836130824, 0.001417850471967226165, 0.002126775707950839464, 0.002835700943934452330, 0.003544626179918065195, 0.004253551415901678928, 0.004962476651885291794, 0.005671401887868904659 ),
 .UNSPECIFIED. ) ;
#2375=CARTESIAN_POINT ( 'NONE',  ( -82.85452780460290967, -35.00000000000000000, -97.27546421900275675 ) ) ;
#2379=CARTESIAN_POINT ( 'NONE',  ( 83.77821517812500929, -33.66562499938548569, 97.61286128772489690 ) ) ;
#2383=CARTESIAN_POINT ( 'NONE',  ( -83.77821517812500929, -33.77812499938548285, -97.61286128772489690 ) ) ;
#2384=CARTESIAN_POINT ( 'NONE',  ( 85.15643035625001289, -31.94062499938548427, 99.99999999999998579 ) ) ;
#2385=CARTESIAN_POINT ( 'NONE',  ( -81.22643902596118437, -32.00000000000000000, -102.6636594982756492 ) ) ;
#2386=CARTESIAN_POINT ( 'NONE',  ( 85.15643035625001289, -33.85312499938549280, -99.99999999999998579 ) ) ;
#2388=CARTESIAN_POINT ( 'NONE',  ( -79.64356964374998427, -33.10312499938548569, 101.5914258081833879 ) ) ;
#2389=CARTESIAN_POINT ( 'NONE',  ( 81.02178482187500208, -30.74062499938548498, -97.61286128772489690 ) ) ;
#2394=CARTESIAN_POINT ( 'NONE',  ( -81.02178482187500208, -31.34062499938548996, 102.3871387122750889 ) ) ;
#2395=CARTESIAN_POINT ( 'NONE',  ( -81.02178482187500208, -30.74062499938548498, 97.61286128772489690 ) ) ;
#2397=ORIENTED_EDGE ( 'NONE', *, *, #10186, .T. ) ;
#2398=CARTESIAN_POINT ( 'NONE',  ( -80.90000000000000568, -34.64999999999999858, -102.5980762113533018 ) ) ;
#2399=CARTESIAN_POINT ( 'NONE',  ( 79.39999999999999147, -32.88750000000000284, -98.26794919243110371 ) ) ;
#2401=CARTESIAN_POINT ( 'NONE',  ( 81.59615242270662350, -32.06115380933863435, -103.0000000000000000 ) ) ;
#2405=CARTESIAN_POINT ( 'NONE',  ( -81.59615242270663771, -32.51115380933863008, -96.99999999999998579 ) ) ;
#2406=CARTESIAN_POINT ( 'NONE',  ( 79.64356964375001269, -30.89062499938548711, 101.5914258081833879 ) ) ;
#2410=CARTESIAN_POINT ( 'NONE',  ( 85.15643035625001289, -34.75312499938548427, -99.99999999999998579 ) ) ;
#2412=EDGE_LOOP ( 'NONE', ( #1035, #4107, #3673, #1185 ) ) ;
#2413=CARTESIAN_POINT ( 'NONE',  ( 79.39999999999999147, -31.10624999877097352, 98.26794919243113213 ) ) ;
#2420=EDGE_CURVE ( 'NONE', #15931, #19033, #10026, .T. ) ;
#2422=CARTESIAN_POINT ( 'NONE',  ( -85.00132729414812616, -34.99999999999999289, -98.78874432549871187 ) ) ;
#2424=CARTESIAN_POINT ( 'NONE',  ( -83.77821517812500929, -31.41562499938548569, -97.61286128772489690 ) ) ;
#2425=CARTESIAN_POINT ( 'NONE',  ( 82.40000000000000568, -32.30624999877097281, 102.9999999999999858 ) ) ;
#2427=CARTESIAN_POINT ( 'NONE',  ( 82.39999999999999147, -33.74062499938548854, 96.81714838363319586 ) ) ;
#2428=VECTOR ( 'NONE', #12896, 1000.000000000000000 ) ;
#2429=CARTESIAN_POINT ( 'NONE',  ( -81.02178482187500208, -31.90312499938548996, -97.61286128772489690 ) ) ;
#2430=CARTESIAN_POINT ( 'NONE',  ( -85.40000000000000568, -30.39374999877097139, -99.99999999999998579 ) ) ;
#2431=CARTESIAN_POINT ( 'NONE',  ( 82.40000000000000568, -34.78124999877096712, -102.9999999999999858 ) ) ;
#2435=CARTESIAN_POINT ( 'NONE',  ( -82.39999999999999147, -32.72812499938548569, -96.81714838363319586 ) ) ;
#2437=EDGE_CURVE ( 'NONE', #12229, #729, #922, .T. ) ;
#2439=ADVANCED_FACE ( 'NONE', ( #19078 ), #6879, .F. ) ;
#2443=CARTESIAN_POINT ( 'NONE',  ( 85.15643035625001289, -33.29062499938547859, -99.99999999999998579 ) ) ;
#2447=VERTEX_POINT ( 'NONE', #11359 ) ;
#2455=ORIENTED_EDGE ( 'NONE', *, *, #5799, .T. ) ;
#2456=CARTESIAN_POINT ( 'NONE',  ( 82.39999999999999147, -33.26250000000000284, -96.53589838486223584 ) ) ;
#2458=CARTESIAN_POINT ( 'NONE',  ( -82.39999999999999147, -31.71562499938548640, 96.81714838363319586 ) ) ;
#2462=CARTESIAN_POINT ( 'NONE',  ( 85.15643035625001289, -34.75312499938548427, -99.99999999999998579 ) ) ;
#2464=CARTESIAN_POINT ( 'NONE',  ( 84.97511176747907768, -35.00000000000000000, 101.5169977320537669 ) ) ;
#2466=VERTEX_POINT ( 'NONE', #3933 ) ;
#2468=DIRECTION ( 'NONE',  ( -0.000000000000000000, -1.000000000000000000, -0.000000000000000000 ) ) ;
#2469=CARTESIAN_POINT ( 'NONE',  ( 82.40000000000000568, -30.00000000000000355, 99.99999999999998579 ) ) ;
#2477=CARTESIAN_POINT ( 'NONE',  ( 80.90000000000000568, -30.75000000000000355, 97.40192378864668399 ) ) ;
#2478=CARTESIAN_POINT ( 'NONE',  ( 83.90000000000000568, -32.71874999877096712, -97.40192378864668399 ) ) ;
#2480=CARTESIAN_POINT ( 'NONE',  ( -81.02178482187500208, -34.45312499938548711, -102.3871387122750889 ) ) ;
#2481=CARTESIAN_POINT ( 'NONE',  ( 83.77821517812500929, -32.76562499938548711, 97.61286128772489690 ) ) ;
#2482=CARTESIAN_POINT ( 'NONE',  ( 83.77821517812500929, -34.37812499938548427, -97.61286128772489690 ) ) ;
#2484=CARTESIAN_POINT ( 'NONE',  ( -81.02178482187500208, -33.14062499938548711, 102.3871387122750889 ) ) ;
#2485=CARTESIAN_POINT ( 'NONE',  ( 82.39999999999999147, -31.15312499938548640, -96.81714838363319586 ) ) ;
#2486=EDGE_LOOP ( 'NONE', ( #14026, #13933, #2455, #4660 ) ) ;
#2487=CARTESIAN_POINT ( 'NONE',  ( 81.02178482187500208, -34.90312499938548285, 102.3871387122750889 ) ) ;
#2491=CARTESIAN_POINT ( 'NONE',  ( -83.77821517812500929, -33.36562499938548854, 97.61286128772489690 ) ) ;
#2492=CARTESIAN_POINT ( 'NONE',  ( -82.39999999999999147, -31.37812499938548427, 103.1828516163667899 ) ) ;
#2498=FACE_OUTER_BOUND ( 'NONE', #7291, .T. ) ;
#2500=CARTESIAN_POINT ( 'NONE',  ( -80.90000000000000568, -32.49374999877097281, -97.40192378864668399 ) ) ;
#2501=CARTESIAN_POINT ( 'NONE',  ( -82.40000000000001990, -34.61250000000001137, 97.00000000000000000 ) ) ;
#2504=DIRECTION ( 'NONE',  ( -0.000000000000000000, 0.000000000000000000, -1.000000000000000000 ) ) ;
#2505=CARTESIAN_POINT ( 'NONE',  ( 85.15643035624999868, -33.81562499938549138, -101.5914258081833879 ) ) ;
#2506=CARTESIAN_POINT ( 'NONE',  ( -85.40000000000000568, -33.09374999877096712, 99.99999999999998579 ) ) ;
#2508=CARTESIAN_POINT ( 'NONE',  ( 80.90000000000000568, -33.24374999877097281, 102.5980762113533018 ) ) ;
#2514=CARTESIAN_POINT ( 'NONE',  ( -82.39999999999999147, -34.07812499938548711, -96.81714838363319586 ) ) ;
#2517=CARTESIAN_POINT ( 'NONE',  ( 85.15643035625001289, -34.26562499938548711, 98.40857419181659793 ) ) ;
#2518=CARTESIAN_POINT ( 'NONE',  ( -83.90000000000000568, -35.26874999877097139, -97.40192378864668399 ) ) ;
#2519=CARTESIAN_POINT ( 'NONE',  ( 83.90000000000000568, -33.52499999999999858, 97.40192378864668399 ) ) ;
#2523=CARTESIAN_POINT ( 'NONE',  ( -83.77821517812500929, -33.66562499938548569, -97.61286128772489690 ) ) ;
#2524=CYLINDRICAL_SURFACE ( 'NONE', #16136, 2.199999999999993516 ) ;
#2525=CARTESIAN_POINT ( 'NONE',  ( 82.39999999999999147, -32.53124999877096712, -103.4641016151377499 ) ) ;
#2527=ORIENTED_EDGE ( 'NONE', *, *, #2244, .F. ) ;
#2531=CARTESIAN_POINT ( 'NONE',  ( 82.39999999999999147, -32.81250000000000000, 103.0000000000000000 ) ) ;
#2537=EDGE_CURVE ( 'NONE', #12381, #5168, #9093, .T. ) ;
#2538=ORIENTED_EDGE ( 'NONE', *, *, #16927, .T. ) ;
#2539=( BOUNDED_CURVE ( )  B_SPLINE_CURVE ( 2, ( #460, #14205, #10795, #4850, #13817, #5341, #11476, #3854, #9918, #5528, #1119, #8731, #17535, #9817, #15880, #10111, #4246, #2577, #17443, #1220, #13035, #16066, #19096, #11279, #2672, #6896, #6986, #12751, #5717, #13126, #15779, #2388, #2484, #8631, #18720, #8442, #8350, #7079, #14589, #7176, #8538, #2778, #14304, #940, #17247, #5626, #12845, #15971, #3953, #14395, #5438, #14488, #4054, #10013, #18814, #1033, #12937, #11572, #18909, #19006, #10204, #17631, #11377, #4150, #11667, #17343, #16167, #842, #6805, #1697, #16356, #4640, #1412, #13321, #10304, #17824, #4532, #9116, #8829, #18119, #19195, #19297, #16648 ),
 .UNSPECIFIED., .F., .F. ) 
 B_SPLINE_CURVE_WITH_KNOTS ( ( 3, 2, 2, 2, 2, 2, 2, 2, 2, 2, 2, 2, 2, 2, 2, 2, 2, 2, 2, 2, 2, 2, 2, 2, 2, 2, 2, 2, 2, 2, 2, 2, 2, 2, 2, 2, 2, 2, 2, 2, 2, 3 ),
 ( 0.3716916592826016164, 0.3750191855951754416, 0.3900199530189824570, 0.4050207204427894725, 0.4200214878665964879, 0.4350222552904035034, 0.4500230227142105188, 0.4650237901380175343, 0.4800245575618244942, 0.4950253249856315096, 0.5100260924094385251, 0.5250268598332455960, 0.5400276272570525560, 0.5550283946808595159, 0.5700291621046665869, 0.5850299295284735468, 0.6000306969522806178, 0.6150314643760875777, 0.6300322317998947597, 0.6450329992237016086, 0.6600337666475086795, 0.6750345340713157505, 0.6900353014951225994, 0.7050360689189296703, 0.7200368363427366303, 0.7350376037665438123, 0.7500383711903506612, 0.7650391386141577321, 0.7800399060379648031, 0.7950406734617718740, 0.8100414408855788340, 0.8250422083093857939, 0.8400429757331928649, 0.8550437431569997138, 0.8700445105808067847, 0.8850452780046138557, 0.9000460454284208156, 0.9150468128522278866, 0.9300475802760349575, 0.9450483476998419174, 0.9600491151236488774, 0.9717223562348836774 ),
 .UNSPECIFIED. ) 
 CURVE ( )  GEOMETRIC_REPRESENTATION_ITEM ( )  RATIONAL_B_SPLINE_CURVE ( ( 0.9537471549767033707, 0.9702812541832881443, 1.000000000000000000, 0.8660254037844387076, 1.000000000000000000, 0.8660254037844387076, 1.000000000000000000, 0.8660254037844387076, 1.000000000000000000, 0.8660254037844387076, 1.000000000000000000, 0.8660254037844387076, 1.000000000000000000, 0.8660254037844387076, 1.000000000000000000, 0.8660254037844387076, 1.000000000000000000, 0.8660254037844387076, 1.000000000000000000, 0.8660254037844387076, 1.000000000000000000, 0.8660254037844387076, 1.000000000000000000, 0.8660254037844387076, 1.000000000000000000, 0.8660254037844387076, 1.000000000000000000, 0.8660254037844387076, 1.000000000000000000, 0.8660254037844387076, 1.000000000000000000, 0.8660254037844387076, 1.000000000000000000, 0.8660254037844387076, 1.000000000000000000, 0.8660254037844387076, 1.000000000000000000, 0.8660254037844387076, 1.000000000000000000, 0.8660254037844387076, 1.000000000000000000, 0.8660254037844387076, 1.000000000000000000, 0.8660254037844387076, 1.000000000000000000, 0.8660254037844387076, 1.000000000000000000, 0.8660254037844387076, 1.000000000000000000, 0.8660254037844387076, 1.000000000000000000, 0.8660254037844387076, 1.000000000000000000, 0.8660254037844387076, 1.000000000000000000, 0.8660254037844387076, 1.000000000000000000, 0.8660254037844387076, 1.000000000000000000, 0.8660254037844387076, 1.000000000000000000, 0.8660254037844387076, 1.000000000000000000, 0.8660254037844387076, 1.000000000000000000, 0.8660254037844387076, 1.000000000000000000, 0.8660254037844387076, 1.000000000000000000, 0.8660254037844387076, 1.000000000000000000, 0.8660254037844387076, 1.000000000000000000, 0.8660254037844387076, 1.000000000000000000, 0.8660254037844387076, 1.000000000000000000, 0.8660254037844387076, 1.000000000000000000, 0.8660254037844387076, 1.000000000000000000, 0.8957441496011365745, 0.9537471549767190249 ) ) 
 REPRESENTATION_ITEM ( '' )  );
#2540=CARTESIAN_POINT ( 'NONE',  ( 79.39999999999999147, -32.88750000000000284, -98.26794919243110371 ) ) ;
#2541=CARTESIAN_POINT ( 'NONE',  ( 83.09162395290297809, -32.00000000000000000, -102.7516965079135502 ) ) ;
#2542=CARTESIAN_POINT ( 'NONE',  ( -83.77821517812500929, -31.67812499938548498, 97.61286128772489690 ) ) ;
#2547=CARTESIAN_POINT ( 'NONE',  ( 79.73531137350353504, -34.99999999999999289, 101.0054374292562187 ) ) ;
#2548=DIRECTION ( 'NONE',  ( -0.000000000000000000, -1.000000000000000000, -0.000000000000000000 ) ) ;
#2549=DIRECTION ( 'NONE',  ( 0.000000000000000000, 0.000000000000000000, 1.000000000000000000 ) ) ;
#2552=CARTESIAN_POINT ( 'NONE',  ( -82.39999999999999147, -30.70312499938548711, -103.1828516163667899 ) ) ;
#2556=CARTESIAN_POINT ( 'NONE',  ( -83.20384757729335945, -34.85759618943233562, -96.99999999999998579 ) ) ;
#2564=CARTESIAN_POINT ( 'NONE',  ( -80.90000000000000568, -30.69374999877097210, 102.5980762113533018 ) ) ;
#2565=CARTESIAN_POINT ( 'NONE',  ( 79.64356964375001269, -34.37812499938548427, 101.5914258081833879 ) ) ;
#2566=CARTESIAN_POINT ( 'NONE',  ( 94.79999999999984084, 0.000000000000000000, 150.0000000000000000 ) ) ;
#2567=VECTOR ( 'NONE', #9890, 1000.000000000000000 ) ;
#2570=( BOUNDED_CURVE ( )  B_SPLINE_CURVE ( 2, ( #16733, #2176, #5116, #16641, #18495, #12335, #11056, #1881, #8133, #3541, #10768, #10961, #344, #9598, #16838, #15562, #17026, #3341, #18399, #15464, #1979, #14085, #10671, #1783, #4920, #15361, #9202, #7936, #5020, #13989, #6383, #6197, #9302, #2075, #4728, #12146, #15266, #10866, #526, #6291, #8031, #9398, #13887, #4827, #15166, #7747, #18114, #7840, #3444, #18209, #12524, #13794, #18302, #16930, #439, #6479, #12432, #13704, #9497, #12240, #628, #6576, #3637, #11352, #1091, #15754, #4029, #817, #16039, #5210, #15658, #18784, #9891, #3731, #2462, #12914, #8508, #914, #2640, #11254, #9989, #8233, #5313 ),
 .UNSPECIFIED., .F., .F. ) 
 B_SPLINE_CURVE_WITH_KNOTS ( ( 3, 2, 2, 2, 2, 2, 2, 2, 2, 2, 2, 2, 2, 2, 2, 2, 2, 2, 2, 2, 2, 2, 2, 2, 2, 2, 2, 2, 2, 2, 2, 2, 2, 2, 2, 2, 2, 2, 2, 2, 2, 3 ),
 ( 0.3495698921800940995, 0.3600184345287980037, 0.3750192026341646057, 0.3900199707395312076, 0.4050207388448978096, 0.4200215069502644116, 0.4350222750556309581, 0.4500230431609975601, 0.4650238112663641621, 0.4800245793717307086, 0.4950253474770972550, 0.5100261155824639125, 0.5250268836878304590, 0.5400276517931970055, 0.5550284198985635520, 0.5700291880039302095, 0.5850299561092967560, 0.6000307242146634135, 0.6150314923200299599, 0.6300322604253966174, 0.6450330285307630529, 0.6600337966361298214, 0.6750345647414963679, 0.6900353328468629144, 0.7050361009522294609, 0.7200368690575960073, 0.7350376371629626648, 0.7500384052683292113, 0.7650391733736958688, 0.7800399414790624153, 0.7950407095844290728, 0.8100414776897955083, 0.8250422457951620547, 0.8400430139005288233, 0.8550437820058953697, 0.8700445501112619162, 0.8850453182166284627, 0.9000460863219950092, 0.9150468544273615557, 0.9300476225327283242, 0.9450483906380948707, 0.9496006163947574574 ),
 .UNSPECIFIED. ) 
 CURVE ( )  GEOMETRIC_REPRESENTATION_ITEM ( )  RATIONAL_B_SPLINE_CURVE ( ( 0.9433623850486894113, 0.9066821623815382036, 1.000000000000000000, 0.8660254037844387076, 1.000000000000000000, 0.8660254037844387076, 1.000000000000000000, 0.8660254037844387076, 1.000000000000000000, 0.8660254037844387076, 1.000000000000000000, 0.8660254037844387076, 1.000000000000000000, 0.8660254037844387076, 1.000000000000000000, 0.8660254037844387076, 1.000000000000000000, 0.8660254037844387076, 1.000000000000000000, 0.8660254037844387076, 1.000000000000000000, 0.8660254037844387076, 1.000000000000000000, 0.8660254037844387076, 1.000000000000000000, 0.8660254037844387076, 1.000000000000000000, 0.8660254037844387076, 1.000000000000000000, 0.8660254037844387076, 1.000000000000000000, 0.8660254037844387076, 1.000000000000000000, 0.8660254037844387076, 1.000000000000000000, 0.8660254037844387076, 1.000000000000000000, 0.8660254037844387076, 1.000000000000000000, 0.8660254037844387076, 1.000000000000000000, 0.8660254037844387076, 1.000000000000000000, 0.8660254037844387076, 1.000000000000000000, 0.8660254037844387076, 1.000000000000000000, 0.8660254037844387076, 1.000000000000000000, 0.8660254037844387076, 1.000000000000000000, 0.8660254037844387076, 1.000000000000000000, 0.8660254037844387076, 1.000000000000000000, 0.8660254037844387076, 1.000000000000000000, 0.8660254037844387076, 1.000000000000000000, 0.8660254037844387076, 1.000000000000000000, 0.8660254037844387076, 1.000000000000000000, 0.8660254037844387076, 1.000000000000000000, 0.8660254037844387076, 1.000000000000000000, 0.8660254037844387076, 1.000000000000000000, 0.8660254037844387076, 1.000000000000000000, 0.8660254037844387076, 1.000000000000000000, 0.8660254037844387076, 1.000000000000000000, 0.8660254037844387076, 1.000000000000000000, 0.8660254037844387076, 1.000000000000000000, 0.8660254037844387076, 1.000000000000000000, 0.9593432414029002819, 0.9433623850486891893 ) ) 
 REPRESENTATION_ITEM ( '' )  );
#2572=CARTESIAN_POINT ( 'NONE',  ( -79.64356964374998427, -33.59062499938548285, -101.5914258081833879 ) ) ;
#2573=CARTESIAN_POINT ( 'NONE',  ( 82.39999999999999147, -34.75312499938549138, 103.1828516163667899 ) ) ;
#2574=CARTESIAN_POINT ( 'NONE',  ( 85.15643035624999868, -33.44062499938548427, -98.40857419181659793 ) ) ;
#2577=CARTESIAN_POINT ( 'NONE',  ( -79.64356964374998427, -32.57812499938548711, 98.40857419181659793 ) ) ;
#2578=CARTESIAN_POINT ( 'NONE',  ( 85.15643035624999868, -31.52812499938547930, -98.40857419181659793 ) ) ;
#2579=VERTEX_POINT ( 'NONE', #6181 ) ;
#2583=CARTESIAN_POINT ( 'NONE',  ( -85.15643035625001289, -34.19062499938548427, 99.99999999999998579 ) ) ;
#2584=CARTESIAN_POINT ( 'NONE',  ( -79.64356964375001269, -31.22812499938548925, 98.40857419181659793 ) ) ;
#2588=CARTESIAN_POINT ( 'NONE',  ( 79.77811200999867935, -34.99999999999999289, -100.8506536761476013 ) ) ;
#2589=CARTESIAN_POINT ( 'NONE',  ( 85.40000000000000568, -33.63750000000000284, -98.26794919243111792 ) ) ;
#2590=ADVANCED_FACE ( 'NONE', ( #12132 ), #14862, .T. ) ;
#2595=CARTESIAN_POINT ( 'NONE',  ( 79.64356964375001269, -30.51562499938548711, 98.40857419181659793 ) ) ;
#2598=CARTESIAN_POINT ( 'NONE',  ( 85.15643035624999868, -34.34062499938548285, -98.40857419181659793 ) ) ;
#2601=CARTESIAN_POINT ( 'NONE',  ( 85.40000000000000568, -32.19374999877096855, 99.99999999999998579 ) ) ;
#2606=CARTESIAN_POINT ( 'NONE',  ( 83.90000000000000568, -34.42500000000000426, 97.40192378864668399 ) ) ;
#2608=EDGE_LOOP ( 'NONE', ( #14282, #8327, #16343, #15423 ) ) ;
#2609=CARTESIAN_POINT ( 'NONE',  ( -79.64356964375001269, -33.02812499938548285, -101.5914258081833879 ) ) ;
#2610=CYLINDRICAL_SURFACE ( 'NONE', #6627, 3.000000000000002665 ) ;
#2612=CARTESIAN_POINT ( 'NONE',  ( 79.64356964374999848, -34.97812499938548569, 99.99999999999998579 ) ) ;
#2613=CARTESIAN_POINT ( 'NONE',  ( -83.77821517812500929, -31.52812499938548996, -97.61286128772489690 ) ) ;
#2614=CARTESIAN_POINT ( 'NONE',  ( 83.33080762004576059, -35.05289549976084373, 103.5578907812544855 ) ) ;
#2615=CARTESIAN_POINT ( 'NONE',  ( -79.73531137350346398, -34.99999999999999289, 98.99456257074389498 ) ) ;
#2620=CARTESIAN_POINT ( 'NONE',  ( 82.39999999999999147, -31.63124999877097210, -103.4641016151377499 ) ) ;
#2630=CARTESIAN_POINT ( 'NONE',  ( -81.59615242270663771, -32.11740381056766580, 103.0000000000000000 ) ) ;
#2635=CARTESIAN_POINT ( 'NONE',  ( 85.40000000000000568, -32.73750000000000426, -98.26794919243111792 ) ) ;
#2636=CARTESIAN_POINT ( 'NONE',  ( -82.39999999999999147, -33.48750000000000426, 103.0000000000000000 ) ) ;
#2637=CARTESIAN_POINT ( 'NONE',  ( -82.39999999999999147, -32.16562499938549280, 96.81714838363319586 ) ) ;
#2639=CARTESIAN_POINT ( 'NONE',  ( -79.39999999999999147, -34.68750000000000000, -101.7320508075688963 ) ) ;
#2640=CARTESIAN_POINT ( 'NONE',  ( 81.02178482187500208, -34.90312499938548285, -97.61286128772489690 ) ) ;
#2641=CARTESIAN_POINT ( 'NONE',  ( 80.48808202378427268, -35.00000000000000000, 102.1951992292041638 ) ) ;
#2642=CARTESIAN_POINT ( 'NONE',  ( -81.02178482187500208, -34.49062499938548854, 102.3871387122750889 ) ) ;
#2646=CARTESIAN_POINT ( 'NONE',  ( -82.39999999999999147, -30.92812499938548143, -96.81714838363319586 ) ) ;
#2651=( BOUNDED_CURVE ( )  B_SPLINE_CURVE ( 2, ( #8921, #10589, #13604, #5811, #16554, #5911, #1513 ),
 .UNSPECIFIED., .F., .F. ) 
 B_SPLINE_CURVE_WITH_KNOTS ( ( 3, 2, 2, 3 ),
 ( 0.8958333333333333703, 0.9027777777777777901, 0.9166666666666666297, 0.9258785066912882389 ),
 .UNSPECIFIED. ) 
 CURVE ( )  GEOMETRIC_REPRESENTATION_ITEM ( )  RATIONAL_B_SPLINE_CURVE ( ( 0.9330127018922192983, 0.9330127018922198534, 1.000000000000000000, 0.8660254037844387076, 1.000000000000000000, 0.9111410165655264848, 0.9401539157124900736 ) ) 
 REPRESENTATION_ITEM ( '' )  );
#2654=CARTESIAN_POINT ( 'NONE',  ( 81.59615242270662350, -32.56740381056766864, 97.00000000000000000 ) ) ;
#2657=EDGE_CURVE ( 'NONE', #5317, #2292, #11838, .T. ) ;
#2660=CARTESIAN_POINT ( 'NONE',  ( -79.39999999999999147, -33.86250000000000426, -98.26794919243113213 ) ) ;
#2661=CARTESIAN_POINT ( 'NONE',  ( 85.15643035625001289, -34.64062499938548711, 99.99999999999998579 ) ) ;
#2665=CARTESIAN_POINT ( 'NONE',  ( -99.99999999999998579, -5.200000000000000178, -150.0000000000000000 ) ) ;
#2666=CARTESIAN_POINT ( 'NONE',  ( -79.64356964374999848, -33.17812499938548854, -99.99999999999998579 ) ) ;
#2667=CARTESIAN_POINT ( 'NONE',  ( 79.64356964375001269, -33.92812499938548854, 101.5914258081833879 ) ) ;
#2669=CARTESIAN_POINT ( 'NONE',  ( 83.77821517812500929, -34.67812499938548854, -102.3871387122750889 ) ) ;
#2672=CARTESIAN_POINT ( 'NONE',  ( -85.15643035625001289, -32.84062499938548285, 99.99999999999998579 ) ) ;
#2673=CARTESIAN_POINT ( 'NONE',  ( 79.64356964375001269, -31.22812499938548925, -98.40857419181659793 ) ) ;
#2676=CARTESIAN_POINT ( 'NONE',  ( 85.15643035624999868, -34.79062499938548569, 101.5914258081833879 ) ) ;
#2680=AXIS2_PLACEMENT_3D ( 'NONE', #9321, #2287, #15484 ) ;
#2681=CARTESIAN_POINT ( 'NONE',  ( -79.64356964374999848, -33.51562499938548711, 99.99999999999998579 ) ) ;
#2683=CARTESIAN_POINT ( 'NONE',  ( -83.20384757729335945, -33.90134618820329848, 102.9999999999999716 ) ) ;
#2684=( BOUNDED_CURVE ( )  B_SPLINE_CURVE ( 2, ( #3057, #13509, #146, #17819, #4429, #9108, #12044, #1692, #11660 ),
 .UNSPECIFIED., .F., .F. ) 
 B_SPLINE_CURVE_WITH_KNOTS ( ( 3, 2, 2, 2, 3 ),
 ( 0.3125000000000001665, 0.3194444444444444198, 0.3333333333333333148, 0.3472222222222222099, 0.3541666666666666297 ),
 .UNSPECIFIED. ) 
 CURVE ( )  GEOMETRIC_REPRESENTATION_ITEM ( )  RATIONAL_B_SPLINE_CURVE ( ( 0.9330127018922194093, 0.9330127018922209636, 1.000000000000000000, 0.8660254037844387076, 1.000000000000000000, 0.8660254037844387076, 1.000000000000000000, 0.9330127018922196314, 0.9330127018922194093 ) ) 
 REPRESENTATION_ITEM ( '' )  );
#2686=CARTESIAN_POINT ( 'NONE',  ( 79.91954014136219087, -34.99999999999998579, -98.55723758691000569 ) ) ;
#2690=CARTESIAN_POINT ( 'NONE',  ( -81.59615242270662350, -32.96115380933864003, 103.0000000000000000 ) ) ;
#2693=CARTESIAN_POINT ( 'NONE',  ( 79.64356964374999848, -32.72812499938548569, 99.99999999999998579 ) ) ;
#2696=CARTESIAN_POINT ( 'NONE',  ( 83.77821517812500929, -34.67812499938548854, -102.3871387122750889 ) ) ;
#2699=ADVANCED_FACE ( 'NONE', ( #16824, #10946, #12223 ), #11043, .T. ) ;
#2700=CARTESIAN_POINT ( 'NONE',  ( 85.40000000000000568, -32.23124999877096997, 101.7320508075688679 ) ) ;
#2702=EDGE_CURVE ( 'NONE', #4468, #10833, #1964, .T. ) ;
#2704=CARTESIAN_POINT ( 'NONE',  ( -83.77821517812500929, -33.32812499938548711, -97.61286128772489690 ) ) ;
#2705=LINE ( 'NONE', #19224, #5247 ) ;
#2708=CARTESIAN_POINT ( 'NONE',  ( -81.02178482187500208, -33.89062499938548711, -102.3871387122750889 ) ) ;
#2710=DIRECTION ( 'NONE',  ( -0.000000000000000000, -0.000000000000000000, -1.000000000000000000 ) ) ;
#2712=CARTESIAN_POINT ( 'NONE',  ( 83.77821517812500929, -34.82812499938548711, 102.3871387122750889 ) ) ;
#2714=CARTESIAN_POINT ( 'NONE',  ( -85.15643035624999868, -31.19062499938548783, -101.5914258081833879 ) ) ;
#2715=CARTESIAN_POINT ( 'NONE',  ( -82.39999999999999147, -31.85624999877097352, -103.4641016151377499 ) ) ;
#2720=CARTESIAN_POINT ( 'NONE',  ( -85.15643035625001289, -32.39062499938548711, -99.99999999999998579 ) ) ;
#2722=DIRECTION ( 'NONE',  ( -0.000000000000000000, -0.000000000000000000, -1.000000000000000000 ) ) ;
#2723=CARTESIAN_POINT ( 'NONE',  ( 85.40000000000000568, -32.19374999877096855, -99.99999999999998579 ) ) ;
#2728=CARTESIAN_POINT ( 'NONE',  ( 83.20395887649171129, -35.00000000000000711, -102.6365808225363878 ) ) ;
#2732=VECTOR ( 'NONE', #4812, 1000.000000000000000 ) ;
#2734=ORIENTED_EDGE ( 'NONE', *, *, #9238, .F. ) ;
#2736=DIRECTION ( 'NONE',  ( -1.586032892321652088E-15, -1.000000000000000000, 0.000000000000000000 ) ) ;
#2740=CARTESIAN_POINT ( 'NONE',  ( 79.39999999999999147, -34.68750000000000000, -98.26794919243110371 ) ) ;
#2743=CARTESIAN_POINT ( 'NONE',  ( -85.15643035624999868, -30.74062499938548143, 98.40857419181659793 ) ) ;
#2749=LINE ( 'NONE', #8607, #13353 ) ;
#2751=ORIENTED_EDGE ( 'NONE', *, *, #7602, .T. ) ;
#2752=PRESENTATION_STYLE_ASSIGNMENT (( #11646 ) ) ;
#2753=CARTESIAN_POINT ( 'NONE',  ( -85.15643035625001289, -35.20312499938548711, -99.99999999999998579 ) ) ;
#2763=ORIENTED_EDGE ( 'NONE', *, *, #1169, .F. ) ;
#2764=CARTESIAN_POINT ( 'NONE',  ( -84.56803305035340657, -32.00000000000000000, 101.7116913729794305 ) ) ;
#2767=CARTESIAN_POINT ( 'NONE',  ( 83.88339518848731302, -35.16733441503058089, 102.5204086375588162 ) ) ;
#2768=CARTESIAN_POINT ( 'NONE',  ( 85.40000000000000568, -34.01250000000000284, -101.7320508075688821 ) ) ;
#2769=AXIS2_PLACEMENT_3D ( 'NONE', #14325, #2504, #1145 ) ;
#2773=CARTESIAN_POINT ( 'NONE',  ( 83.77821517812500929, -35.01562499938548711, 97.61286128772489690 ) ) ;
#2775=EDGE_CURVE ( 'NONE', #18799, #19181, #50, .T. ) ;
#2776=CARTESIAN_POINT ( 'NONE',  ( 81.02178482187500208, -31.34062499938548996, -102.3871387122750889 ) ) ;
#2778=CARTESIAN_POINT ( 'NONE',  ( -79.64356964374998427, -33.47812499938547859, 98.40857419181659793 ) ) ;
#2779=CARTESIAN_POINT ( 'NONE',  ( 85.15643035624999868, -31.97812499938548925, -98.40857419181659793 ) ) ;
#2780=ORIENTED_EDGE ( 'NONE', *, *, #6300, .T. ) ;
#2785=CARTESIAN_POINT ( 'NONE',  ( -85.15643035624999868, -32.35312499938549280, 101.5914258081833879 ) ) ;
#2786=ORIENTED_EDGE ( 'NONE', *, *, #5809, .F. ) ;
#2788=EDGE_CURVE ( 'NONE', #18284, #16539, #8118, .T. ) ;
#2791=LINE ( 'NONE', #14501, #4873 ) ;
#2797=CARTESIAN_POINT ( 'NONE',  ( 85.15643035624999868, -32.99062499938548854, 101.5914258081833879 ) ) ;
#2801=CARTESIAN_POINT ( 'NONE',  ( 79.64356964374999848, -33.62812499938548427, -99.99999999999998579 ) ) ;
#2802=CARTESIAN_POINT ( 'NONE',  ( -79.64356964375001269, -30.89062499938548711, -101.5914258081833879 ) ) ;
#2803=ORIENTED_EDGE ( 'NONE', *, *, #8175, .F. ) ;
#2804=CARTESIAN_POINT ( 'NONE',  ( 85.40000000000000568, -32.64374999877097139, 99.99999999999998579 ) ) ;
#2805=CYLINDRICAL_SURFACE ( 'NONE', #4619, 5.199999999999996625 ) ;
#2810=CARTESIAN_POINT ( 'NONE',  ( -82.39999999999999147, -34.97812499938547859, -96.81714838363319586 ) ) ;
#2813=PLANE ( 'NONE',  #11708 ) ;
#2814=CARTESIAN_POINT ( 'NONE',  ( -83.77821517812500929, -34.37812499938548427, -102.3871387122750889 ) ) ;
#2816=CARTESIAN_POINT ( 'NONE',  ( -80.90000000000000568, -30.99374999877096926, -102.5980762113533018 ) ) ;
#2823=CARTESIAN_POINT ( 'NONE',  ( 80.90000000000000568, -31.44374999877096855, -97.40192378864668399 ) ) ;
#2827=CARTESIAN_POINT ( 'NONE',  ( 79.64356964374998427, -34.45312499938548711, -101.5914258081833879 ) ) ;
#2837=CARTESIAN_POINT ( 'NONE',  ( -80.52691934816500918, -34.99999999999999289, 102.0537355158133010 ) ) ;
#2838=CARTESIAN_POINT ( 'NONE',  ( 85.40000000000000568, -34.50000000000000000, -99.99999999999998579 ) ) ;
#2840=CARTESIAN_POINT ( 'NONE',  ( -79.64356964375001269, -34.11562499938548854, 101.5914258081833879 ) ) ;
#2847=CARTESIAN_POINT ( 'NONE',  ( 85.24876232368478668, -35.00000000000000711, 99.45334139304991083 ) ) ;
#2850=( NAMED_UNIT ( * ) SI_UNIT ( $, .STERADIAN. ) SOLID_ANGLE_UNIT ( ) );
#2851=CARTESIAN_POINT ( 'NONE',  ( -85.15643035624999868, -31.00312499938548072, -98.40857419181659793 ) ) ;
#2853=DIRECTION ( 'NONE',  ( -0.000000000000000000, -1.000000000000000000, -0.000000000000000000 ) ) ;
#2854=DIRECTION ( 'NONE',  ( 1.000000000000000000, -1.586032892321652285E-15, 0.000000000000000000 ) ) ;
#2856=CARTESIAN_POINT ( 'NONE',  ( 79.39999999999999147, -33.33749999999999858, 101.7320508075688963 ) ) ;
#2859=ORIENTED_EDGE ( 'NONE', *, *, #9611, .T. ) ;
#2860=CARTESIAN_POINT ( 'NONE',  ( -84.01447415327271528, -35.02670941564510088, -102.7431224211893692 ) ) ;
#2862=CARTESIAN_POINT ( 'NONE',  ( -85.40000000000000568, -31.25624999877096855, 101.7320508075688679 ) ) ;
#2863=CARTESIAN_POINT ( 'NONE',  ( 85.40000000000000568, -30.41249999999999787, 98.26794919243111792 ) ) ;
#2867=CARTESIAN_POINT ( 'NONE',  ( 81.02178482187500208, -34.04062499938548569, 97.61286128772489690 ) ) ;
#2869=AXIS2_PLACEMENT_3D ( 'NONE', #5103, #11045, #17011 ) ;
#2870=CARTESIAN_POINT ( 'NONE',  ( 81.02178482187500208, -31.79062499938548925, -102.3871387122750889 ) ) ;
#2872=FACE_OUTER_BOUND ( 'NONE', #12974, .T. ) ;
#2873=CARTESIAN_POINT ( 'NONE',  ( 81.02178482187500208, -32.54062499938548569, -97.61286128772489690 ) ) ;
#2874=VERTEX_POINT ( 'NONE', #4199 ) ;
#2878=CARTESIAN_POINT ( 'NONE',  ( -85.15643035624999868, -32.80312499938548854, 101.5914258081833879 ) ) ;
#2879=VERTEX_POINT ( 'NONE', #6858 ) ;
#2880=CARTESIAN_POINT ( 'NONE',  ( -85.40000000000000568, -33.99374999877097281, 99.99999999999998579 ) ) ;
#2881=VECTOR ( 'NONE', #3509, 1000.000000000000000 ) ;
#2882=AXIS2_PLACEMENT_3D ( 'NONE', #7560, #352, #1699 ) ;
#2886=LINE ( 'NONE', #14698, #15152 ) ;
#2887=DIRECTION ( 'NONE',  ( -0.000000000000000000, -0.000000000000000000, -1.000000000000000000 ) ) ;
#2890=CARTESIAN_POINT ( 'NONE',  ( 83.77821517812500929, -33.32812499938548711, 97.61286128772489690 ) ) ;
#2891=CARTESIAN_POINT ( 'NONE',  ( 82.40000000000000568, -30.00000000000000355, 99.99999999999998579 ) ) ;
#2892=CARTESIAN_POINT ( 'NONE',  ( -79.39999999999999147, -32.51250000000000284, -98.26794919243113213 ) ) ;
#2893=CARTESIAN_POINT ( 'NONE',  ( -85.11512745526623291, -32.00000000000000000, -99.40473233008064824 ) ) ;
#2894=CARTESIAN_POINT ( 'NONE',  ( -79.64356964375001269, -31.79062499938548569, -101.5914258081833879 ) ) ;
#2898=CARTESIAN_POINT ( 'NONE',  ( 83.90000000000000568, -32.71874999877096712, 102.5980762113533018 ) ) ;
#2899=CYLINDRICAL_SURFACE ( 'NONE', #8645, 3.000000000000002665 ) ;
#2901=CARTESIAN_POINT ( 'NONE',  ( -85.15643035624999868, -30.66562499938548569, 101.5914258081833879 ) ) ;
#2902=CARTESIAN_POINT ( 'NONE',  ( 82.14831453752277923, -31.99999999999999289, 102.8584433575407218 ) ) ;
#2904=CARTESIAN_POINT ( 'NONE',  ( -83.77821517812500929, -33.81562499938548427, -102.3871387122750889 ) ) ;
#2905=CARTESIAN_POINT ( 'NONE',  ( -99.99999999999998579, -3.000000000000000000, 150.0000000000000000 ) ) ;
#2908=CARTESIAN_POINT ( 'NONE',  ( -83.77821517812500929, -33.77812499938548285, -97.61286128772489690 ) ) ;
#2911=CARTESIAN_POINT ( 'NONE',  ( -83.90000000000000568, -31.81874999877096855, -102.5980762113533018 ) ) ;
#2915=CARTESIAN_POINT ( 'NONE',  ( -82.39999999999999147, -34.75312499938548427, -103.1828516163667899 ) ) ;
#2916=CARTESIAN_POINT ( 'NONE',  ( -82.40000000000001990, -32.53124999877097423, 103.0000000000000000 ) ) ;
#2918=CARTESIAN_POINT ( 'NONE',  ( 80.90000000000000568, -32.94374999877096855, -102.5980762113533018 ) ) ;
#2927=ORIENTED_EDGE ( 'NONE', *, *, #6057, .F. ) ;
#2928=ORIENTED_EDGE ( 'NONE', *, *, #10234, .F. ) ;
#2929=CARTESIAN_POINT ( 'NONE',  ( 82.40000000000000568, -34.38749999999999574, -102.9999999999999858 ) ) ;
#2933=CARTESIAN_POINT ( 'NONE',  ( -81.44948931429647132, -34.99999999999999289, 102.5934467159354284 ) ) ;
#2935=CARTESIAN_POINT ( 'NONE',  ( -79.64356964375001269, -33.59062499938548285, 98.40857419181659793 ) ) ;
#2941=CARTESIAN_POINT ( 'NONE',  ( -79.91954014136211981, -34.99999999999999289, -101.4427624130898238 ) ) ;
#2943=ORIENTED_EDGE ( 'NONE', *, *, #13179, .F. ) ;
#2944=CARTESIAN_POINT ( 'NONE',  ( -85.15643035624999868, -33.77812499938548285, -101.5914258081833879 ) ) ;
#2945=CARTESIAN_POINT ( 'NONE',  ( -85.40000000000000568, -33.63750000000000284, 98.26794919243111792 ) ) ;
#2954=CARTESIAN_POINT ( 'NONE',  ( -85.16931825408420309, -31.99999999999999289, 100.2387112178438144 ) ) ;
#2956=CARTESIAN_POINT ( 'NONE',  ( -85.40000000000000568, -32.19374999877096855, 99.99999999999998579 ) ) ;
#2957=CARTESIAN_POINT ( 'NONE',  ( 79.39999999999999147, -31.16250000000000497, 98.26794919243113213 ) ) ;
#2958=EDGE_CURVE ( 'NONE', #11282, #609, #5302, .T. ) ;
#2962=CARTESIAN_POINT ( 'NONE',  ( 85.15643035625001289, -33.74062499938548854, 99.99999999999998579 ) ) ;
#2963=CARTESIAN_POINT ( 'NONE',  ( 83.77821517812500929, -30.66562499938548569, -97.61286128772489690 ) ) ;
#2966=CARTESIAN_POINT ( 'NONE',  ( 79.39999999999999147, -34.25624999877096855, 98.26794919243113213 ) ) ;
#2967=CARTESIAN_POINT ( 'NONE',  ( 79.64356964375001269, -33.10312499938549280, -101.5914258081833879 ) ) ;
#2972=CARTESIAN_POINT ( 'NONE',  ( -81.02178482187500208, -34.94062499938548427, 102.3871387122750889 ) ) ;
#2976=CARTESIAN_POINT ( 'NONE',  ( 83.77821517812500929, -30.21562499938548285, 102.3871387122750889 ) ) ;
#2982=CARTESIAN_POINT ( 'NONE',  ( 81.02178482187500208, -32.65312499938548996, 102.3871387122750889 ) ) ;
#2983=CARTESIAN_POINT ( 'NONE',  ( 80.90000000000000568, -32.04374999877096997, 97.40192378864668399 ) ) ;
#2985=CARTESIAN_POINT ( 'NONE',  ( -81.02178482187500208, -32.80312499938548854, 102.3871387122750889 ) ) ;
#2986=CARTESIAN_POINT ( 'NONE',  ( -79.64356964375001269, -32.31562499938548427, -98.40857419181659793 ) ) ;
#2987=VECTOR ( 'NONE', #16966, 1000.000000000000000 ) ;
#2988=VERTEX_POINT ( 'NONE', #9141 ) ;
#2989=CARTESIAN_POINT ( 'NONE',  ( 85.40000000000000568, -34.93124999877096570, 101.7320508075688679 ) ) ;
#2992=CARTESIAN_POINT ( 'NONE',  ( 82.39999999999999147, -32.36250000000000426, -96.99999999999998579 ) ) ;
#2993=CARTESIAN_POINT ( 'NONE',  ( -81.02178482187500208, -31.45312499938549067, 102.3871387122750889 ) ) ;
#2994=CARTESIAN_POINT ( 'NONE',  ( 82.40000000000001990, -33.88124999877096855, -103.0000000000000000 ) ) ;
#2995=ORIENTED_EDGE ( 'NONE', *, *, #5185, .F. ) ;
#2996=CARTESIAN_POINT ( 'NONE',  ( -80.90000000000000568, -31.50000000000000000, -102.5980762113533018 ) ) ;
#2999=CARTESIAN_POINT ( 'NONE',  ( -85.15643035624999868, -33.36562499938548854, -98.40857419181659793 ) ) ;
#3002=CARTESIAN_POINT ( 'NONE',  ( -85.40000000000000568, -30.84374999877096712, -99.99999999999998579 ) ) ;
#3007=CARTESIAN_POINT ( 'NONE',  ( 81.02178482187500208, -33.59062499938548285, 97.61286128772489690 ) ) ;
#3008=CARTESIAN_POINT ( 'NONE',  ( 79.39999999999999147, -32.43750000000000000, -98.26794919243110371 ) ) ;
#3009=LINE ( 'NONE', #295, #13323 ) ;
#3010=CARTESIAN_POINT ( 'NONE',  ( 79.39999999999999147, -35.11874999877096570, -99.99999999999998579 ) ) ;
#3019=VERTEX_POINT ( 'NONE', #81 ) ;
#3022=DIRECTION ( 'NONE',  ( 0.000000000000000000, -1.000000000000000000, 0.000000000000000000 ) ) ;
#3023=CARTESIAN_POINT ( 'NONE',  ( -83.90000000000000568, -32.26874999877097139, 97.40192378864668399 ) ) ;
#3025=LINE ( 'NONE', #1574, #12339 ) ;
#3026=MECHANICAL_DESIGN_GEOMETRIC_PRESENTATION_REPRESENTATION('',(#8945),#15212);
#3027=FACE_OUTER_BOUND ( 'NONE', #11912, .T. ) ;
#3029=CARTESIAN_POINT ( 'NONE',  ( -85.15643035624999868, -32.99062499938548854, 98.40857419181659793 ) ) ;
#3033=DIRECTION ( 'NONE',  ( -1.000000000000000000, 0.000000000000000000, 0.000000000000000000 ) ) ;
#3034=CARTESIAN_POINT ( 'NONE',  ( 82.40000000000000568, -30.00000000000000355, 99.99999999999998579 ) ) ;
#3037=CARTESIAN_POINT ( 'NONE',  ( -83.90000000000000568, -34.42500000000000426, -97.40192378864668399 ) ) ;
#3039=VECTOR ( 'NONE', #11839, 1000.000000000000000 ) ;
#3040=CARTESIAN_POINT ( 'NONE',  ( -82.39999999999999147, -32.72812499938548569, -96.81714838363319586 ) ) ;
#3043=CARTESIAN_POINT ( 'NONE',  ( 81.44948931429642869, -35.00000000000001421, -102.5934467159354284 ) ) ;
#3045=CARTESIAN_POINT ( 'NONE',  ( 82.40000000000001990, -32.13750000000000284, -103.0000000000000000 ) ) ;
#3049=VERTEX_POINT ( 'NONE', #2992 ) ;
#3050=CARTESIAN_POINT ( 'NONE',  ( -83.90000000000000568, -34.87500000000000000, -97.40192378864668399 ) ) ;
#3052=CARTESIAN_POINT ( 'NONE',  ( -85.40000000000000568, -31.29374999877096997, 99.99999999999998579 ) ) ;
#3053=CARTESIAN_POINT ( 'NONE',  ( 85.40000000000000568, -31.35000000000000142, 99.99999999999998579 ) ) ;
#3055=CARTESIAN_POINT ( 'NONE',  ( -82.15584532983336885, -31.99999999999999289, -97.13032736203112449 ) ) ;
#3057=CARTESIAN_POINT ( 'NONE',  ( 82.40000000000000568, -32.08124999877097139, 97.00000000000000000 ) ) ;
#3060=CARTESIAN_POINT ( 'NONE',  ( 81.02178482187500208, -30.89062499938548711, -102.3871387122750889 ) ) ;
#3063=CARTESIAN_POINT ( 'NONE',  ( 82.39999999999999147, -34.33124999877097139, 97.00000000000000000 ) ) ;
#3064=CARTESIAN_POINT ( 'NONE',  ( 79.64356964374999848, -33.06562499938548427, -99.99999999999998579 ) ) ;
#3066=ADVANCED_FACE ( 'NONE', ( #1631 ), #4764, .F. ) ;
#3068=CARTESIAN_POINT ( 'NONE',  ( -85.40000000000000568, -31.31250000000000000, 101.7320508075688679 ) ) ;
#3069=ORIENTED_EDGE ( 'NONE', *, *, #12723, .F. ) ;
#3070=CARTESIAN_POINT ( 'NONE',  ( -82.40000000000000568, -33.03750000000000142, 102.9999999999999858 ) ) ;
#3076=CARTESIAN_POINT ( 'NONE',  ( -83.20384757729337366, -32.34240381056766722, 97.00000000000000000 ) ) ;
#3079=CARTESIAN_POINT ( 'NONE',  ( 79.64356964375001269, -33.14062499938548711, 101.5914258081833879 ) ) ;
#3080=CARTESIAN_POINT ( 'NONE',  ( 79.64356964375001269, -30.44062499938548783, -98.40857419181659793 ) ) ;
#3082=CARTESIAN_POINT ( 'NONE',  ( -82.39999999999999147, -32.39062499938548711, 103.1828516163667899 ) ) ;
#3083=CARTESIAN_POINT ( 'NONE',  ( -79.64356964375001269, -30.96562499938548640, -98.40857419181659793 ) ) ;
#3085=CARTESIAN_POINT ( 'NONE',  ( 83.90000000000000568, -34.96874999877096712, 102.5980762113533018 ) ) ;
#3088=CARTESIAN_POINT ( 'NONE',  ( -85.15643035625001289, -32.50312499938548427, 99.99999999999998579 ) ) ;
#3089=DIRECTION ( 'NONE',  ( -0.000000000000000000, -0.000000000000000000, -1.000000000000000000 ) ) ;
#3091=CARTESIAN_POINT ( 'NONE',  ( -80.90000000000000568, -30.75000000000000355, -97.40192378864668399 ) ) ;
#3093=CARTESIAN_POINT ( 'NONE',  ( -83.90000000000000568, -34.96874999877096712, -102.5980762113533018 ) ) ;
#3095=CARTESIAN_POINT ( 'NONE',  ( -85.15643035624999868, -33.89062499938548711, -101.5914258081833879 ) ) ;
#3103=CARTESIAN_POINT ( 'NONE',  ( 81.02178482187500208, -34.04062499938548569, 97.61286128772489690 ) ) ;
#3106=CARTESIAN_POINT ( 'NONE',  ( 79.39999999999999147, -33.80624999877097281, -101.7320508075688537 ) ) ;
#3115=CARTESIAN_POINT ( 'NONE',  ( -81.22643902601926413, -32.00000000000000000, 97.33634050170186924 ) ) ;
#3121=( BOUNDED_CURVE ( )  B_SPLINE_CURVE ( 2, ( #4705, #5976, #15247, #6362, #321, #3127, #126, #9086, #6076 ),
 .UNSPECIFIED., .F., .F. ) 
 B_SPLINE_CURVE_WITH_KNOTS ( ( 3, 2, 2, 2, 3 ),
 ( 0.6041666666666666297, 0.6111111111111111605, 0.6250000000000000000, 0.6388888888888888395, 0.6458333333333332593 ),
 .UNSPECIFIED. ) 
 CURVE ( )  GEOMETRIC_REPRESENTATION_ITEM ( )  RATIONAL_B_SPLINE_CURVE ( ( 0.9330127018922192983, 0.9330127018922187432, 1.000000000000000000, 0.8660254037844387076, 1.000000000000000000, 0.8660254037844387076, 1.000000000000000000, 0.9330127018922198534, 0.9330127018922192983 ) ) 
 REPRESENTATION_ITEM ( '' )  );
#3122=CARTESIAN_POINT ( 'NONE',  ( -79.64356964375001269, -33.66562499938549280, 101.5914258081833879 ) ) ;
#3126=DIRECTION ( 'NONE',  ( 0.000000000000000000, -1.000000000000000000, 0.000000000000000000 ) ) ;
#3127=CARTESIAN_POINT ( 'NONE',  ( -79.39999999999999147, -33.41250000000000142, 101.7320508075688537 ) ) ;
#3128=CARTESIAN_POINT ( 'NONE',  ( -79.64057174634722003, -35.00000000000000000, -99.60353574117785058 ) ) ;
#3130=VERTEX_POINT ( 'NONE', #15012 ) ;
#3132=CARTESIAN_POINT ( 'NONE',  ( -82.39999999999999147, -34.30312499938548143, -103.1828516163667899 ) ) ;
#3141=PLANE ( 'NONE',  #15070 ) ;
#3144=CARTESIAN_POINT ( 'NONE',  ( -80.90000000000000568, -32.94374999877096855, 102.5980762113533018 ) ) ;
#3145=CARTESIAN_POINT ( 'NONE',  ( 79.39999999999999147, -31.53750000000000497, 101.7320508075688821 ) ) ;
#3149=CARTESIAN_POINT ( 'NONE',  ( 80.90000000000000568, -33.45000000000000284, -102.5980762113533018 ) ) ;
#3150=CARTESIAN_POINT ( 'NONE',  ( 85.15643035624999868, -32.35312499938549280, -101.5914258081833879 ) ) ;
#3153=EDGE_CURVE ( 'NONE', #7460, #6753, #5346, .T. ) ;
#3155=CARTESIAN_POINT ( 'NONE',  ( 83.77821517812500929, -32.31562499938548427, -102.3871387122750889 ) ) ;
#3156=ADVANCED_FACE ( 'NONE', ( #18725 ), #3279, .F. ) ;
#3157=FACE_OUTER_BOUND ( 'NONE', #15930, .T. ) ;
#3158=CARTESIAN_POINT ( 'NONE',  ( -79.39999999999999147, -34.63124999877096855, 98.26794919243110371 ) ) ;
#3160=ADVANCED_FACE ( 'NONE', ( #10873 ), #18215, .T. ) ;
#3161=CARTESIAN_POINT ( 'NONE',  ( -83.77821517812500929, -34.71562499938548285, 97.61286128772489690 ) ) ;
#3162=ORIENTED_EDGE ( 'NONE', *, *, #7927, .T. ) ;
#3164=MANIFOLD_SOLID_BREP ( 'M5 Clearance Hole1', #13153 ) ;
#3166=CARTESIAN_POINT ( 'NONE',  ( -94.79999999999999716, -3.000000000000000000, -150.0000000000000000 ) ) ;
#3167=( BOUNDED_CURVE ( )  B_SPLINE_CURVE ( 2, ( #15636, #16999, #2241, #4999, #17196, #3516, #9571, #9769, #3900 ),
 .UNSPECIFIED., .F., .F. ) 
 B_SPLINE_CURVE_WITH_KNOTS ( ( 3, 2, 2, 2, 3 ),
 ( 0.6875000000000000000, 0.6944444444444444198, 0.7083333333333333703, 0.7222222222222222099, 0.7291666666666666297 ),
 .UNSPECIFIED. ) 
 CURVE ( )  GEOMETRIC_REPRESENTATION_ITEM ( )  RATIONAL_B_SPLINE_CURVE ( ( 0.9330127018922194093, 0.9330127018922194093, 1.000000000000000000, 0.8660254037844387076, 1.000000000000000000, 0.8660254037844387076, 1.000000000000000000, 0.9330127018922198534, 0.9330127018922192983 ) ) 
 REPRESENTATION_ITEM ( '' )  );
#3169=CARTESIAN_POINT ( 'NONE',  ( 94.79999999999984084, 0.000000000000000000, -150.0000000000000000 ) ) ;
#3170=EDGE_CURVE ( 'NONE', #1228, #7532, #8516, .T. ) ;
#3171=CARTESIAN_POINT ( 'NONE',  ( -82.39999999999999147, -32.36250000000000426, 96.99999999999997158 ) ) ;
#3172=CARTESIAN_POINT ( 'NONE',  ( 82.39999999999999147, -30.70312499938548711, 103.1828516163667899 ) ) ;
#3176=CARTESIAN_POINT ( 'NONE',  ( -85.15643035624999868, -32.09062499938548996, -101.5914258081833879 ) ) ;
#3178=CARTESIAN_POINT ( 'NONE',  ( 82.39999999999999147, -31.49062499938548854, 96.81714838363319586 ) ) ;
#3180=AXIS2_PLACEMENT_3D ( 'NONE', #15910, #8669, #8472 ) ;
#3183=CARTESIAN_POINT ( 'NONE',  ( -85.15643035625001289, -31.60312499938548569, 99.99999999999998579 ) ) ;
#3184=CARTESIAN_POINT ( 'NONE',  ( 83.20384757729333103, -33.18615380933863435, 103.0000000000000000 ) ) ;
#3187=CARTESIAN_POINT ( 'NONE',  ( -83.90000000000000568, -32.32500000000000284, -102.5980762113533018 ) ) ;
#3189=CARTESIAN_POINT ( 'NONE',  ( -85.40000000000000568, -34.89374999877097139, -99.99999999999998579 ) ) ;
#3190=CARTESIAN_POINT ( 'NONE',  ( -82.39999999999999147, -33.29062499938549280, -96.81714838363319586 ) ) ;
#3197=CARTESIAN_POINT ( 'NONE',  ( 83.77821517812500929, -32.91562499938547859, 102.3871387122750889 ) ) ;
#3200=LINE ( 'NONE', #7506, #12695 ) ;
#3201=CARTESIAN_POINT ( 'NONE',  ( 85.40000000000000568, -33.58124999877097139, -98.26794919243111792 ) ) ;
#3203=ORIENTED_EDGE ( 'NONE', *, *, #5324, .T. ) ;
#3213=AXIS2_PLACEMENT_3D ( 'NONE', #8648, #15988, #18834 ) ;
#3214=FACE_BOUND ( 'NONE', #6954, .T. ) ;
#3215=CARTESIAN_POINT ( 'NONE',  ( -79.39999999999999147, -34.72500000000000142, 99.99999999999998579 ) ) ;
#3219=CARTESIAN_POINT ( 'NONE',  ( -82.39999999999999147, -33.74062499938548854, 103.1828516163667899 ) ) ;
#3229=CARTESIAN_POINT ( 'NONE',  ( -79.64356964374999848, -32.16562499938548569, -99.99999999999998579 ) ) ;
#3231=CARTESIAN_POINT ( 'NONE',  ( -85.40000000000000568, -32.64374999877097139, 99.99999999999998579 ) ) ;
#3233=DIRECTION ( 'NONE',  ( -1.000000000000000000, 0.000000000000000000, 0.000000000000000000 ) ) ;
#3234=( BOUNDED_CURVE ( )  B_SPLINE_CURVE ( 2, ( #1623, #1340, #15005, #6118, #4362, #13623, #10322, #19214, #19318 ),
 .UNSPECIFIED., .F., .F. ) 
 B_SPLINE_CURVE_WITH_KNOTS ( ( 3, 2, 2, 2, 3 ),
 ( 0.4791666666666666297, 0.4861111111111111049, 0.5000000000000000000, 0.5138888888888888395, 0.5208333333333333703 ),
 .UNSPECIFIED. ) 
 CURVE ( )  GEOMETRIC_REPRESENTATION_ITEM ( )  RATIONAL_B_SPLINE_CURVE ( ( 0.9330127018922194093, 0.9330127018922190762, 1.000000000000000000, 0.8660254037844387076, 1.000000000000000000, 0.8660254037844387076, 1.000000000000000000, 0.9330127018922187432, 0.9330127018922192983 ) ) 
 REPRESENTATION_ITEM ( '' )  );
#3235=ORIENTED_EDGE ( 'NONE', *, *, #13289, .F. ) ;
#3236=ORIENTED_EDGE ( 'NONE', *, *, #4702, .T. ) ;
#3238=CARTESIAN_POINT ( 'NONE',  ( 79.39999999999999147, -33.28124999877096712, -98.26794919243110371 ) ) ;
#3240=CARTESIAN_POINT ( 'NONE',  ( -82.39999999999999147, -32.98124999877096997, 103.4641016151377499 ) ) ;
#3241=CARTESIAN_POINT ( 'NONE',  ( 85.40000000000000568, -30.86250000000000071, 98.26794919243111792 ) ) ;
#3242=CARTESIAN_POINT ( 'NONE',  ( -69.99999999999998579, -32.00000000000000000, -150.0000000000000000 ) ) ;
#3244=CARTESIAN_POINT ( 'NONE',  ( 81.22643902596138332, -31.99999999999999289, -97.33634050172426555 ) ) ;
#3246=CARTESIAN_POINT ( 'NONE',  ( 82.39999999999999147, -34.52812499938548996, -103.1828516163667899 ) ) ;
#3249=CARTESIAN_POINT ( 'NONE',  ( -85.40000000000000568, -34.01250000000000284, 101.7320508075688821 ) ) ;
#3250=CARTESIAN_POINT ( 'NONE',  ( 81.02178482187500208, -34.04062499938548569, -102.3871387122750889 ) ) ;
#3251=EDGE_CURVE ( 'NONE', #3695, #11212, #1200, .T. ) ;
#3252=ADVANCED_FACE ( 'NONE', ( #18889 ), #10179, .F. ) ;
#3256=CARTESIAN_POINT ( 'NONE',  ( -85.15643035624999868, -35.05312499938548143, 101.5914258081833879 ) ) ;
#3266=CARTESIAN_POINT ( 'NONE',  ( 84.82992844608111227, -32.00000000000000000, 101.3134070403133080 ) ) ;
#3267=CARTESIAN_POINT ( 'NONE',  ( 85.15643035625001289, -35.20312499938548711, 99.99999999999998579 ) ) ;
#3268=EDGE_CURVE ( 'NONE', #11655, #14259, #4127, .T. ) ;
#3269=CARTESIAN_POINT ( 'NONE',  ( 85.15643035625001289, -32.05312499938548854, -99.99999999999998579 ) ) ;
#3271=CARTESIAN_POINT ( 'NONE',  ( -85.12124608221316180, -32.00000000000002132, -100.4735569575799445 ) ) ;
#3272=CARTESIAN_POINT ( 'NONE',  ( -83.77821517812500929, -33.47812499938548569, -102.3871387122750889 ) ) ;
#3273=ORIENTED_EDGE ( 'NONE', *, *, #12900, .T. ) ;
#3274=CARTESIAN_POINT ( 'NONE',  ( 79.39999999999999147, -34.66874999877096997, 99.99999999999998579 ) ) ;
#3277=DIRECTION ( 'NONE',  ( 0.000000000000000000, 0.000000000000000000, 1.000000000000000000 ) ) ;
#3278=CARTESIAN_POINT ( 'NONE',  ( -81.02178482187500208, -31.90312499938548996, 102.3871387122750889 ) ) ;
#3279=( BOUNDED_SURFACE ( )  B_SPLINE_SURFACE ( 1, 2, ( 
 ( #3570, #12756, #14310, #3861, #9430, #13921, #658, #2007, #14023, #2296, #15495, #18428, #6706, #14210, #5048, #5243, #11286, #17255, #6606, #6810, #8165, #847, #10897, #948, #9823, #3763, #15397, #7967, #11088, #3670, #12653, #3471, #2394, #10992, #16959, #751, #9530, #17155, #6903, #2108, #18625, #8356, #8069, #12851, #12555, #4956, #9635, #17057, #11192, #15596, #16865, #2204, #14114, #17541, #8449, #14792, #16175, #4159, #10309, #2785, #5632, #8737, #5725, #16267, #15886, #8638, #8836, #13229, #19102, #14595, #18916, #2878, #5819, #18823, #14691, #1325, #11767, #7182, #1419, #3959, #9925, #5535, #7372, #16072, #5445, #10117, #2491, #12944, #11578, #14401, #2681, #1040, #7275, #14495, #19203, #6993, #1227, #13131, #17743, #11483, #4349, #11383, #17349, #11674, #17449, #4060, #10020, #15979, #2583, #17638, #8544, #1128, #7085, #13041, #19012, #4253, #10212, #4537, #1520, #355, #14992, #10595, #3161, #6209, #4740, #9314, #7654, #4645, #2972, #15178, #1795, #3256, #9121, #10400, #10686, #9030, #7471 ),
 ( #4442, #58, #15085, #16362, #12157, #15278, #13428, #1702, #4838, #10497, #7759, #8928, #13328, #18221, #6302, #16653, #9212, #18125, #13610, #16559, #252, #11958, #7563, #17928, #13714, #12252, #13519, #16744, #10781, #156, #6107, #14890, #3357, #1893, #19304, #3068, #5917, #11863, #17830, #6007, #16461, #1614, #12056, #18032, #6396, #12443, #5031, #15476, #448, #12536, #12349, #3453, #2089, #18315, #14002, #14096, #9410, #8044, #2188, #1992, #5126, #4934, #7851, #8144, #15575, #11069, #17039, #6589, #640, #9510, #18508, #15375, #18411, #7948, #9614, #3650, #10971, #735, #6689, #16941, #3553, #13806, #10878, #16849, #13901, #538, #6494, #3621, #17033, #2081, #1985, #15664, #3643, #18406, #11164, #9605, #6486, #15570, #6584, #17131, #16739, #9503, #9702, #14091, #634, #15471, #443, #3737, #6684, #351, #2181, #8139, #12627, #8038, #2274, #4834, #10775, #6389, #8238, #16937, #6297, #10967, #3349, #13800, #12438, #9309, #3548, #15272, #731, #15370, #18601, #1887, #5026, #13994, #5216, #7846, #12248 ) ),
 .UNSPECIFIED., .F., .F., .F. ) 
 B_SPLINE_SURFACE_WITH_KNOTS ( ( 2, 2 ),
 ( 3, 2, 2, 2, 2, 2, 2, 2, 2, 2, 2, 2, 2, 2, 2, 2, 2, 2, 2, 2, 2, 2, 2, 2, 2, 2, 2, 2, 2, 2, 2, 2, 2, 2, 2, 2, 2, 2, 2, 2, 2, 2, 2, 2, 2, 2, 2, 2, 2, 2, 2, 2, 2, 2, 2, 2, 2, 2, 2, 2, 2, 2, 2, 2, 2, 2, 2, 2, 3 ),
 ( 0.000000000000000000, 1.000000000000000000 ),
 ( 0.000000000000000000, 0.01388888888888888812, 0.02777777777777777624, 0.04166666666666666435, 0.05555555555555555247, 0.06944444444444444753, 0.08333333333333332871, 0.09722222222222222376, 0.1111111111111111049, 0.1250000000000000000, 0.1388888888888888951, 0.1527777777777777901, 0.1666666666666666574, 0.1805555555555555525, 0.1944444444444444475, 0.2083333333333333426, 0.2222222222222222099, 0.2361111111111111049, 0.2500000000000000000, 0.2638888888888888951, 0.2777777777777777901, 0.2916666666666666852, 0.3055555555555555802, 0.3194444444444444198, 0.3333333333333333148, 0.3472222222222222099, 0.3611111111111111049, 0.3750000000000000000, 0.3888888888888888951, 0.4027777777777777901, 0.4166666666666666852, 0.4305555555555555802, 0.4444444444444444198, 0.4583333333333333148, 0.4722222222222222099, 0.4861111111111111049, 0.5000000000000000000, 0.5138888888888888395, 0.5277777777777777901, 0.5416666666666666297, 0.5555555555555555802, 0.5694444444444444198, 0.5833333333333333703, 0.5972222222222222099, 0.6111111111111111605, 0.6250000000000000000, 0.6388888888888888395, 0.6527777777777777901, 0.6666666666666666297, 0.6805555555555555802, 0.6944444444444444198, 0.7083333333333333703, 0.7222222222222222099, 0.7361111111111111605, 0.7500000000000000000, 0.7638888888888888395, 0.7777777777777777901, 0.7916666666666666297, 0.8055555555555555802, 0.8194444444444444198, 0.8333333333333333703, 0.8472222222222222099, 0.8611111111111111605, 0.8750000000000000000, 0.8888888888888888395, 0.9027777777777777901, 0.9166666666666666297, 0.9258785066912882389, 0.9351372917582011501 ),
 .UNSPECIFIED. ) 
 GEOMETRIC_REPRESENTATION_ITEM ( )  RATIONAL_B_SPLINE_SURFACE ( (
 ( 1.000000000000000000, 0.8660254037844387076, 1.000000000000000000, 0.8660254037844387076, 1.000000000000000000, 0.8660254037844387076, 1.000000000000000000, 0.8660254037844387076, 1.000000000000000000, 0.8660254037844387076, 1.000000000000000000, 0.8660254037844387076, 1.000000000000000000, 0.8660254037844387076, 1.000000000000000000, 0.8660254037844387076, 1.000000000000000000, 0.8660254037844387076, 1.000000000000000000, 0.8660254037844387076, 1.000000000000000000, 0.8660254037844387076, 1.000000000000000000, 0.8660254037844387076, 1.000000000000000000, 0.8660254037844387076, 1.000000000000000000, 0.8660254037844387076, 1.000000000000000000, 0.8660254037844387076, 1.000000000000000000, 0.8660254037844387076, 1.000000000000000000, 0.8660254037844387076, 1.000000000000000000, 0.8660254037844387076, 1.000000000000000000, 0.8660254037844387076, 1.000000000000000000, 0.8660254037844387076, 1.000000000000000000, 0.8660254037844387076, 1.000000000000000000, 0.8660254037844387076, 1.000000000000000000, 0.8660254037844387076, 1.000000000000000000, 0.8660254037844387076, 1.000000000000000000, 0.8660254037844387076, 1.000000000000000000, 0.8660254037844387076, 1.000000000000000000, 0.8660254037844387076, 1.000000000000000000, 0.8660254037844387076, 1.000000000000000000, 0.8660254037844387076, 1.000000000000000000, 0.8660254037844387076, 1.000000000000000000, 0.8660254037844387076, 1.000000000000000000, 0.8660254037844387076, 1.000000000000000000, 0.8660254037844387076, 1.000000000000000000, 0.8660254037844387076, 1.000000000000000000, 0.8660254037844387076, 1.000000000000000000, 0.8660254037844387076, 1.000000000000000000, 0.8660254037844387076, 1.000000000000000000, 0.8660254037844387076, 1.000000000000000000, 0.8660254037844387076, 1.000000000000000000, 0.8660254037844387076, 1.000000000000000000, 0.8660254037844387076, 1.000000000000000000, 0.8660254037844387076, 1.000000000000000000, 0.8660254037844387076, 1.000000000000000000, 0.8660254037844387076, 1.000000000000000000, 0.8660254037844387076, 1.000000000000000000, 0.8660254037844387076, 1.000000000000000000, 0.8660254037844387076, 1.000000000000000000, 0.8660254037844387076, 1.000000000000000000, 0.8660254037844387076, 1.000000000000000000, 0.8660254037844387076, 1.000000000000000000, 0.8660254037844387076, 1.000000000000000000, 0.8660254037844387076, 1.000000000000000000, 0.8660254037844387076, 1.000000000000000000, 0.8660254037844387076, 1.000000000000000000, 0.8660254037844387076, 1.000000000000000000, 0.8660254037844387076, 1.000000000000000000, 0.8660254037844387076, 1.000000000000000000, 0.8660254037844387076, 1.000000000000000000, 0.8660254037844387076, 1.000000000000000000, 0.8660254037844387076, 1.000000000000000000, 0.8660254037844387076, 1.000000000000000000, 0.8660254037844387076, 1.000000000000000000, 0.8660254037844387076, 1.000000000000000000, 0.8660254037844387076, 1.000000000000000000, 0.8660254037844387076, 1.000000000000000000, 0.8660254037844387076, 1.000000000000000000, 0.9111410165655264848, 0.9401539157124900736, 0.9401539157124900736, 0.9401539157124900736),
 ( 1.000000000000000000, 0.8660254037844387076, 1.000000000000000000, 0.8660254037844387076, 1.000000000000000000, 0.8660254037844387076, 1.000000000000000000, 0.8660254037844387076, 1.000000000000000000, 0.8660254037844387076, 1.000000000000000000, 0.8660254037844387076, 1.000000000000000000, 0.8660254037844387076, 1.000000000000000000, 0.8660254037844387076, 1.000000000000000000, 0.8660254037844387076, 1.000000000000000000, 0.8660254037844387076, 1.000000000000000000, 0.8660254037844387076, 1.000000000000000000, 0.8660254037844387076, 1.000000000000000000, 0.8660254037844387076, 1.000000000000000000, 0.8660254037844387076, 1.000000000000000000, 0.8660254037844387076, 1.000000000000000000, 0.8660254037844387076, 1.000000000000000000, 0.8660254037844387076, 1.000000000000000000, 0.8660254037844387076, 1.000000000000000000, 0.8660254037844387076, 1.000000000000000000, 0.8660254037844387076, 1.000000000000000000, 0.8660254037844387076, 1.000000000000000000, 0.8660254037844387076, 1.000000000000000000, 0.8660254037844387076, 1.000000000000000000, 0.8660254037844387076, 1.000000000000000000, 0.8660254037844387076, 1.000000000000000000, 0.8660254037844387076, 1.000000000000000000, 0.8660254037844387076, 1.000000000000000000, 0.8660254037844387076, 1.000000000000000000, 0.8660254037844387076, 1.000000000000000000, 0.8660254037844387076, 1.000000000000000000, 0.8660254037844387076, 1.000000000000000000, 0.8660254037844387076, 1.000000000000000000, 0.8660254037844387076, 1.000000000000000000, 0.8660254037844387076, 1.000000000000000000, 0.8660254037844387076, 1.000000000000000000, 0.8660254037844387076, 1.000000000000000000, 0.8660254037844387076, 1.000000000000000000, 0.8660254037844387076, 1.000000000000000000, 0.8660254037844387076, 1.000000000000000000, 0.8660254037844387076, 1.000000000000000000, 0.8660254037844387076, 1.000000000000000000, 0.8660254037844387076, 1.000000000000000000, 0.8660254037844387076, 1.000000000000000000, 0.8660254037844387076, 1.000000000000000000, 0.8660254037844387076, 1.000000000000000000, 0.8660254037844387076, 1.000000000000000000, 0.8660254037844387076, 1.000000000000000000, 0.8660254037844387076, 1.000000000000000000, 0.8660254037844387076, 1.000000000000000000, 0.8660254037844387076, 1.000000000000000000, 0.8660254037844387076, 1.000000000000000000, 0.8660254037844387076, 1.000000000000000000, 0.8660254037844387076, 1.000000000000000000, 0.8660254037844387076, 1.000000000000000000, 0.8660254037844387076, 1.000000000000000000, 0.8660254037844387076, 1.000000000000000000, 0.8660254037844387076, 1.000000000000000000, 0.8660254037844387076, 1.000000000000000000, 0.8660254037844387076, 1.000000000000000000, 0.8660254037844387076, 1.000000000000000000, 0.8660254037844387076, 1.000000000000000000, 0.8660254037844387076, 1.000000000000000000, 0.8660254037844387076, 1.000000000000000000, 0.8660254037844387076, 1.000000000000000000, 0.8660254037844387076, 1.000000000000000000, 0.8660254037844387076, 1.000000000000000000, 0.9111410165655264848, 0.9401539157124900736, 0.9401539157124900736, 0.9401539157124900736) ) ) 
 REPRESENTATION_ITEM ( '' )  SURFACE ( )  );
#3282=CARTESIAN_POINT ( 'NONE',  ( -82.39999999999999147, -31.46250000000000568, -103.4641016151377499 ) ) ;
#3290=CARTESIAN_POINT ( 'NONE',  ( 85.40000000000000568, -32.25000000000000000, 99.99999999999998579 ) ) ;
#3291=CARTESIAN_POINT ( 'NONE',  ( 82.39999999999999147, -32.27812499938548285, 96.81714838363319586 ) ) ;
#3294=EDGE_CURVE ( 'NONE', #17606, #16850, #8423, .T. ) ;
#3295=CARTESIAN_POINT ( 'NONE',  ( -82.40000000000000568, -30.00000000000000355, -99.99999999999998579 ) ) ;
#3297=CARTESIAN_POINT ( 'NONE',  ( 82.39999999999999147, -33.65624999877096712, -96.53589838486223584 ) ) ;
#3305=ORIENTED_EDGE ( 'NONE', *, *, #6502, .F. ) ;
#3307=ORIENTED_EDGE ( 'NONE', *, *, #17732, .F. ) ;
#3311=ORIENTED_EDGE ( 'NONE', *, *, #13489, .T. ) ;
#3316=( BOUNDED_CURVE ( )  B_SPLINE_CURVE ( 2, ( #6775, #2360, #3823, #18593, #9696, #7051, #5409, #18696, #14371 ),
 .UNSPECIFIED., .F., .T. ) 
 B_SPLINE_CURVE_WITH_KNOTS ( ( 3, 2, 2, 2, 3 ),
 ( 0.6458333333333333703, 0.6527777777777777901, 0.6666666666666666297, 0.6805555555555555802, 0.6875000000000000000 ),
 .UNSPECIFIED. ) 
 CURVE ( )  GEOMETRIC_REPRESENTATION_ITEM ( )  RATIONAL_B_SPLINE_CURVE ( ( 0.9330127018922192983, 0.9330127018922198534, 1.000000000000000000, 0.8660254037844387076, 1.000000000000000000, 0.8660254037844387076, 1.000000000000000000, 0.9330127018922194093, 0.9330127018922194093 ) ) 
 REPRESENTATION_ITEM ( '' )  );
#3324=CARTESIAN_POINT ( 'NONE',  ( -85.15643035624999868, -32.42812499938548854, -101.5914258081833879 ) ) ;
#3326=ORIENTED_EDGE ( 'NONE', *, *, #6826, .F. ) ;
#3327=CARTESIAN_POINT ( 'NONE',  ( -81.59615242270665192, -33.28259618943233278, -103.0000000000000000 ) ) ;
#3332=ORIENTED_EDGE ( 'NONE', *, *, #5431, .T. ) ;
#3335=CARTESIAN_POINT ( 'NONE',  ( 83.90000000000000568, -30.52500000000000213, -97.40192378864668399 ) ) ;
#3337=CARTESIAN_POINT ( 'NONE',  ( -85.15643035625001289, -30.25312499938548783, 99.99999999999998579 ) ) ;
#3338=CARTESIAN_POINT ( 'NONE',  ( 85.40000000000000568, -31.80000000000000071, 99.99999999999998579 ) ) ;
#3341=CARTESIAN_POINT ( 'NONE',  ( 82.39999999999999147, -32.61562499938548854, -96.81714838363319586 ) ) ;
#3344=FACE_OUTER_BOUND ( 'NONE', #6841, .T. ) ;
#3346=CARTESIAN_POINT ( 'NONE',  ( 79.64356964375001269, -34.00312499938549138, -101.5914258081833879 ) ) ;
#3347=ORIENTED_EDGE ( 'NONE', *, *, #404, .F. ) ;
#3349=CARTESIAN_POINT ( 'NONE',  ( -83.90000000000000568, -34.57500000000000284, 97.40192378864668399 ) ) ;
#3352=CARTESIAN_POINT ( 'NONE',  ( 83.90000000000000568, -33.46874999877096712, -102.5980762113533018 ) ) ;
#3353=UNCERTAINTY_MEASURE_WITH_UNIT (LENGTH_MEASURE( 1.000000000000000082E-05 ), #9798, 'distance_accuracy_value', 'NONE');
#3354=DIRECTION ( 'NONE',  ( -0.000000000000000000, -1.000000000000000000, -0.000000000000000000 ) ) ;
#3357=CARTESIAN_POINT ( 'NONE',  ( -80.90000000000000568, -31.20000000000000284, 102.5980762113533018 ) ) ;
#3360=VECTOR ( 'NONE', #6757, 1000.000000000000000 ) ;
#3362=CARTESIAN_POINT ( 'NONE',  ( 79.64356964375001269, -31.22812499938548925, 101.5914258081833879 ) ) ;
#3365=B_SPLINE_CURVE_WITH_KNOTS ( 'NONE', 3,
 ( #18436, #8075, #8172, #12858, #6614, #18828, #11391, #18632, #5056, #2117 ),
 .UNSPECIFIED., .F., .F.,
 ( 4, 2, 2, 2, 4 ),
 ( 0.3612006186103786654, 0.3925526867148934063, 0.4239047548194081472, 0.4552568229239228881, 0.4866088910284376290 ),
 .UNSPECIFIED. ) ;
#3367=CARTESIAN_POINT ( 'NONE',  ( 84.28136653320187577, -32.00000000000000000, -97.98546077809228905 ) ) ;
#3370=CARTESIAN_POINT ( 'NONE',  ( 83.77821517812500929, -30.96562499938548640, 97.61286128772489690 ) ) ;
#3371=CARTESIAN_POINT ( 'NONE',  ( 83.77821517812500929, -31.52812499938548996, -102.3871387122750889 ) ) ;
#3373=CARTESIAN_POINT ( 'NONE',  ( -85.15643035625001289, -32.95312499938548711, 99.99999999999998579 ) ) ;
#3374=CARTESIAN_POINT ( 'NONE',  ( -79.64356964375001269, -32.69062499938548427, -101.5914258081833879 ) ) ;
#3377=CARTESIAN_POINT ( 'NONE',  ( 85.15643035624999868, -30.74062499938548143, 101.5914258081833879 ) ) ;
#3382=CARTESIAN_POINT ( 'NONE',  ( -81.02178482187500208, -33.10312499938548569, 97.61286128772489690 ) ) ;
#3385=CARTESIAN_POINT ( 'NONE',  ( -79.39999999999999147, -30.67500000000000071, -99.99999999999998579 ) ) ;
#3386=CARTESIAN_POINT ( 'NONE',  ( 79.39999999999999147, -34.72500000000000142, -99.99999999999998579 ) ) ;
#3388=CARTESIAN_POINT ( 'NONE',  ( -82.39999999999999147, -34.64062499938548711, -96.81714838363319586 ) ) ;
#3394=CARTESIAN_POINT ( 'NONE',  ( 99.99999999999994316, -21.80000000000003268, -137.3499999999999943 ) ) ;
#3396=CARTESIAN_POINT ( 'NONE',  ( 83.77821517812500929, -34.56562499938548427, 97.61286128772489690 ) ) ;
#3397=DIRECTION ( 'NONE',  ( -0.000000000000000000, -1.000000000000000000, -0.000000000000000000 ) ) ;
#3399=CARTESIAN_POINT ( 'NONE',  ( 79.64356964374999848, -31.37812499938548427, -99.99999999999998579 ) ) ;
#3409=CARTESIAN_POINT ( 'NONE',  ( -80.24181665645332373, -32.00000000000000711, 97.97695283456452842 ) ) ;
#3411=FACE_OUTER_BOUND ( 'NONE', #1796, .T. ) ;
#3412=CARTESIAN_POINT ( 'NONE',  ( -82.40000000000001990, -34.16250000000000853, -103.0000000000000000 ) ) ;
#3415=CARTESIAN_POINT ( 'NONE',  ( -83.90000000000000568, -34.51874999877097139, -102.5980762113533018 ) ) ;
#3419=CARTESIAN_POINT ( 'NONE',  ( 85.16220480609065646, -34.99999999999999289, -98.91314642826793602 ) ) ;
#3421=EDGE_CURVE ( 'NONE', #12300, #13090, #7280, .T. ) ;
#3423=FACE_OUTER_BOUND ( 'NONE', #14442, .T. ) ;
#3426=ORIENTED_EDGE ( 'NONE', *, *, #8204, .F. ) ;
#3430=CARTESIAN_POINT ( 'NONE',  ( 82.40000000000000568, -30.00000000000000355, 103.0000000000000000 ) ) ;
#3431=CARTESIAN_POINT ( 'NONE',  ( 82.49978216248241836, -35.00000000000000711, -102.7603866155199910 ) ) ;
#3432=CARTESIAN_POINT ( 'NONE',  ( 82.40000000000000568, -33.03750000000000142, -102.9999999999999858 ) ) ;
#3438=CARTESIAN_POINT ( 'NONE',  ( -82.15584532983329780, -32.00000000000000000, 102.8696726379688329 ) ) ;
#3439=CARTESIAN_POINT ( 'NONE',  ( 82.39999999999999147, -30.33750000000000213, -103.4641016151377499 ) ) ;
#3441=CARTESIAN_POINT ( 'NONE',  ( -80.90000000000000568, -34.74374999877097281, 102.5980762113533018 ) ) ;
#3443=CARTESIAN_POINT ( 'NONE',  ( 81.59615242270662350, -33.22634618820330843, 102.9999999999999858 ) ) ;
#3444=CARTESIAN_POINT ( 'NONE',  ( 83.77821517812500929, -33.77812499938548285, -102.3871387122750889 ) ) ;
#3445=CARTESIAN_POINT ( 'NONE',  ( 81.90908125315206689, -31.99999999999999289, -97.16185054499327123 ) ) ;
#3446=CARTESIAN_POINT ( 'NONE',  ( -81.02178482187500208, -32.54062499938548569, 97.61286128772489690 ) ) ;
#3447=CARTESIAN_POINT ( 'NONE',  ( 81.02178482187500208, -34.34062499938548285, -97.61286128772489690 ) ) ;
#3448=ORIENTED_EDGE ( 'NONE', *, *, #18470, .F. ) ;
#3453=CARTESIAN_POINT ( 'NONE',  ( -82.39999999999999147, -31.91250000000000497, 96.53589838486223584 ) ) ;
#3455=CARTESIAN_POINT ( 'NONE',  ( -85.00132729414809774, -35.00000000000000000, 101.2112556745012881 ) ) ;
#3456=CARTESIAN_POINT ( 'NONE',  ( 82.32247963938024782, -34.99999999999998579, 97.23891671615865562 ) ) ;
#3457=CARTESIAN_POINT ( 'NONE',  ( 82.39999999999999147, -31.82812499938548356, 96.81714838363319586 ) ) ;
#3458=CARTESIAN_POINT ( 'NONE',  ( 83.90000000000000568, -32.56874999877096855, -102.5980762113533018 ) ) ;
#3460=CARTESIAN_POINT ( 'NONE',  ( 79.79666399293472523, -31.99999999999999289, 98.51078102784474311 ) ) ;
#3461=CARTESIAN_POINT ( 'NONE',  ( 83.77821517812500929, -34.37812499938548427, 102.3871387122750889 ) ) ;
#3463=CARTESIAN_POINT ( 'NONE',  ( 82.39999999999999147, -30.81562499938548427, -96.81714838363319586 ) ) ;
#3465=CARTESIAN_POINT ( 'NONE',  ( -79.64356964374999848, -33.17812499938548854, 99.99999999999998579 ) ) ;
#3466=CARTESIAN_POINT ( 'NONE',  ( -79.64356964374999848, -32.72812499938548569, -99.99999999999998579 ) ) ;
#3468=ORIENTED_EDGE ( 'NONE', *, *, #10593, .F. ) ;
#3469=CARTESIAN_POINT ( 'NONE',  ( 83.77821517812500929, -33.77812499938548285, 97.61286128772489690 ) ) ;
#3471=CARTESIAN_POINT ( 'NONE',  ( -79.64356964375001269, -31.30312499938548854, 101.5914258081833879 ) ) ;
#3472=CARTESIAN_POINT ( 'NONE',  ( -82.39999999999999147, -33.74062499938548854, 103.1828516163667899 ) ) ;
#3473=CARTESIAN_POINT ( 'NONE',  ( 83.90000000000000568, -33.01874999877097139, 97.40192378864668399 ) ) ;
#3475=CARTESIAN_POINT ( 'NONE',  ( -79.39999999999999147, -33.82500000000000284, -99.99999999999998579 ) ) ;
#3477=CARTESIAN_POINT ( 'NONE',  ( 82.39999999999999147, -33.65624999877097423, 103.0000000000000000 ) ) ;
#3486=CYLINDRICAL_SURFACE ( 'NONE', #15828, 3.000000000000002665 ) ;
#3487=CARTESIAN_POINT ( 'NONE',  ( 85.15643035624999868, -32.54062499938548569, -98.40857419181659793 ) ) ;
#3503=DIRECTION ( 'NONE',  ( 0.000000000000000000, -0.000000000000000000, -1.000000000000000000 ) ) ;
#3506=CARTESIAN_POINT ( 'NONE',  ( -79.39999999999999147, -33.28124999877096712, -101.7320508075688821 ) ) ;
#3509=DIRECTION ( 'NONE',  ( -0.000000000000000000, -1.000000000000000000, -0.000000000000000000 ) ) ;
#3513=B_SPLINE_CURVE_WITH_KNOTS ( 'NONE', 3,
 ( #5404, #17409, #10077, #4023, #16132, #5686, #18972, #1000, #16234, #7234, #11634, #15938, #2541, #14455, #1087, #7045, #18779, #10169 ),
 .UNSPECIFIED., .F., .F.,
 ( 4, 2, 2, 2, 2, 2, 2, 2, 4 ),
 ( 0.000000000000000000, 0.0007106627595359784168, 0.001421325519071956834, 0.002131988278607935359, 0.002842651038143913667, 0.003553313797679891976, 0.004263976557215870718, 0.004974639316751849026, 0.005685302076287827334 ),
 .UNSPECIFIED. ) ;
#3515=CARTESIAN_POINT ( 'NONE',  ( -79.77811200999879304, -35.00000000000000000, -99.14934632385212865 ) ) ;
#3516=CARTESIAN_POINT ( 'NONE',  ( -79.39999999999999147, -34.25624999877096855, 101.7320508075688537 ) ) ;
#3520=CARTESIAN_POINT ( 'NONE',  ( -85.15643035624999868, -34.60312499938548569, -98.40857419181659793 ) ) ;
#3525=DIRECTION ( 'NONE',  ( 1.000000000000000000, -4.625929269271494788E-16, 0.000000000000000000 ) ) ;
#3529=CARTESIAN_POINT ( 'NONE',  ( 79.39999999999999147, -32.06250000000000000, 98.26794919243113213 ) ) ;
#3530=ORIENTED_EDGE ( 'NONE', *, *, #11184, .T. ) ;
#3531=CYLINDRICAL_SURFACE ( 'NONE', #15707, 3.000000000000002665 ) ;
#3534=CARTESIAN_POINT ( 'NONE',  ( 80.90000000000000568, -34.59374999877096712, 102.5980762113533018 ) ) ;
#3536=CARTESIAN_POINT ( 'NONE',  ( 80.90000000000000568, -30.75000000000000355, -102.5980762113533018 ) ) ;
#3538=CARTESIAN_POINT ( 'NONE',  ( -82.39999999999999147, -35.00624999877097565, 96.53589838486223584 ) ) ;
#3539=CARTESIAN_POINT ( 'NONE',  ( -83.20384757729338787, -32.10134618820330132, -97.00000000000000000 ) ) ;
#3541=CARTESIAN_POINT ( 'NONE',  ( 79.64356964374998427, -32.31562499938548427, -101.5914258081833879 ) ) ;
#3543=CARTESIAN_POINT ( 'NONE',  ( -82.39999999999999147, -32.27812499938548285, 103.1828516163667899 ) ) ;
#3544=CARTESIAN_POINT ( 'NONE',  ( 83.77821517812500929, -33.21562499938548285, -102.3871387122750889 ) ) ;
#3547=EDGE_CURVE ( 'NONE', #4006, #18536, #1866, .T. ) ;
#3548=CARTESIAN_POINT ( 'NONE',  ( -79.39999999999999147, -34.72500000000000142, 99.99999999999998579 ) ) ;
#3553=CARTESIAN_POINT ( 'NONE',  ( -80.90000000000000568, -33.00000000000000000, 102.5980762113533018 ) ) ;
#3555=CARTESIAN_POINT ( 'NONE',  ( 94.79999999999984084, 0.000000000000000000, 150.0000000000000000 ) ) ;
#3556=EDGE_CURVE ( 'NONE', #11655, #8657, #2027, .T. ) ;
#3557=CARTESIAN_POINT ( 'NONE',  ( 81.79008970393682887, -35.00000000000001421, 97.30603528924578427 ) ) ;
#3558=CARTESIAN_POINT ( 'NONE',  ( 85.15643035625001289, -31.49062499938548498, 99.99999999999998579 ) ) ;
#3561=CARTESIAN_POINT ( 'NONE',  ( 79.68596062386927770, -32.00000000000000000, 98.72172371342817598 ) ) ;
#3562=CARTESIAN_POINT ( 'NONE',  ( 79.64356964374999848, -30.36562499938548498, 99.99999999999998579 ) ) ;
#3563=CARTESIAN_POINT ( 'NONE',  ( 79.64356964375001269, -31.41562499938548569, -101.5914258081833879 ) ) ;
#3565=CARTESIAN_POINT ( 'NONE',  ( -85.15643035625001289, -33.44062499938548427, 98.40857419181659793 ) ) ;
#3566=CARTESIAN_POINT ( 'NONE',  ( -85.15643035624999868, -32.46562499938548996, -98.40857419181659793 ) ) ;
#3568=CARTESIAN_POINT ( 'NONE',  ( 79.64356964375001269, -31.79062499938548569, 101.5914258081833879 ) ) ;
#3570=CARTESIAN_POINT ( 'NONE',  ( -85.15643035625001289, -30.14062499938548711, 99.99999999999998579 ) ) ;
#3571=CARTESIAN_POINT ( 'NONE',  ( -85.15643035624999868, -34.79062499938548569, 98.40857419181659793 ) ) ;
#3573=ORIENTED_EDGE ( 'NONE', *, *, #10096, .T. ) ;
#3574=CARTESIAN_POINT ( 'NONE',  ( -80.90000000000000568, -33.75000000000000000, -102.5980762113533018 ) ) ;
#3577=CARTESIAN_POINT ( 'NONE',  ( -82.40000000000000568, -30.00000000000000355, 96.99999999999998579 ) ) ;
#3584=CARTESIAN_POINT ( 'NONE',  ( 85.15643035625001289, -34.64062499938548711, 99.99999999999998579 ) ) ;
#3585=FACE_OUTER_BOUND ( 'NONE', #1484, .T. ) ;
#3587=CARTESIAN_POINT ( 'NONE',  ( 79.64356964375001269, -30.89062499938548711, -98.40857419181659793 ) ) ;
#3588=CARTESIAN_POINT ( 'NONE',  ( 79.39999999999999147, -34.72500000000000142, 99.99999999999998579 ) ) ;
#3590=CARTESIAN_POINT ( 'NONE',  ( 82.39999999999999147, -31.40624999877097068, 103.4641016151377499 ) ) ;
#3595=CARTESIAN_POINT ( 'NONE',  ( -79.39999999999999147, -32.88750000000000284, -101.7320508075688963 ) ) ;
#3597=ORIENTED_EDGE ( 'NONE', *, *, #12577, .F. ) ;
#3598=CARTESIAN_POINT ( 'NONE',  ( -82.39999999999999147, -31.37812499938548427, -96.81714838363319586 ) ) ;
#3599=CARTESIAN_POINT ( 'NONE',  ( 82.40000000000000568, -33.03750000000000142, 96.99999999999998579 ) ) ;
#3601=CARTESIAN_POINT ( 'NONE',  ( 83.77821517812500929, -32.42812499938548854, 97.61286128772489690 ) ) ;
#3602=CARTESIAN_POINT ( 'NONE',  ( -79.39999999999999147, -33.76874999877097139, -99.99999999999998579 ) ) ;
#3610=CARTESIAN_POINT ( 'NONE',  ( 81.59615242270662350, -34.31115380933863435, -102.9999999999999716 ) ) ;
#3614=CARTESIAN_POINT ( 'NONE',  ( 79.64356964374998427, -32.20312499938548711, -101.5914258081833879 ) ) ;
#3615=CARTESIAN_POINT ( 'NONE',  ( -81.02178482187500208, -34.49062499938548854, -97.61286128772489690 ) ) ;
#3619=CARTESIAN_POINT ( 'NONE',  ( -79.39999999999999147, -33.33749999999999858, -101.7320508075688963 ) ) ;
#3621=CARTESIAN_POINT ( 'NONE',  ( -82.39999999999999147, -33.26250000000000284, 96.53589838486223584 ) ) ;
#3626=ORIENTED_EDGE ( 'NONE', *, *, #1534, .F. ) ;
#3627=CARTESIAN_POINT ( 'NONE',  ( 79.39999999999999147, -34.66874999877096997, 99.99999999999998579 ) ) ;
#3628=CARTESIAN_POINT ( 'NONE',  ( 82.39999999999999147, -34.52812499938548996, -103.1828516163667899 ) ) ;
#3631=CARTESIAN_POINT ( 'NONE',  ( -79.39999999999999147, -34.66874999877096997, 99.99999999999998579 ) ) ;
#3633=CARTESIAN_POINT ( 'NONE',  ( -82.40000000000000568, -33.43124999877096570, 102.9999999999999858 ) ) ;
#3636=EDGE_CURVE ( 'NONE', #7020, #15108, #7919, .T. ) ;
#3637=CARTESIAN_POINT ( 'NONE',  ( 85.15643035625001289, -34.30312499938548854, -99.99999999999998579 ) ) ;
#3638=CARTESIAN_POINT ( 'NONE',  ( -82.39999999999999147, -33.65624999877097423, 97.00000000000000000 ) ) ;
#3639=CARTESIAN_POINT ( 'NONE',  ( -85.15643035625001289, -34.19062499938548427, 99.99999999999998579 ) ) ;
#3640=CARTESIAN_POINT ( 'NONE',  ( 81.02178482187500208, -34.49062499938548854, -102.3871387122750889 ) ) ;
#3641=ORIENTED_EDGE ( 'NONE', *, *, #5907, .T. ) ;
#3643=CARTESIAN_POINT ( 'NONE',  ( -80.90000000000000568, -33.45000000000000284, 102.5980762113533018 ) ) ;
#3645=CARTESIAN_POINT ( 'NONE',  ( 83.20384757729335945, -33.45134618820330985, -102.9999999999999858 ) ) ;
#3649=AXIS2_PLACEMENT_3D ( 'NONE', #2665, #10746, #15244 ) ;
#3650=CARTESIAN_POINT ( 'NONE',  ( -82.39999999999999147, -32.81250000000000000, 96.53589838486223584 ) ) ;
#3652=CARTESIAN_POINT ( 'NONE',  ( -82.39999999999999147, -33.43124999877097281, -96.99999999999998579 ) ) ;
#3654=CARTESIAN_POINT ( 'NONE',  ( 85.15643035624999868, -33.25312499938548427, 98.40857419181659793 ) ) ;
#3656=CARTESIAN_POINT ( 'NONE',  ( -99.99999999999998579, -29.80000000000000426, 150.0000000000000000 ) ) ;
#3659=CARTESIAN_POINT ( 'NONE',  ( -82.39999999999999147, -32.84062499938548996, -96.81714838363319586 ) ) ;
#3660=CARTESIAN_POINT ( 'NONE',  ( 79.64356964375001269, -32.20312499938548001, 98.40857419181659793 ) ) ;
#3661=CARTESIAN_POINT ( 'NONE',  ( 82.39999999999999147, -32.39062499938548001, -103.1828516163667899 ) ) ;
#3662=EDGE_CURVE ( 'NONE', #800, #12300, #15738, .T. ) ;
#3664=CARTESIAN_POINT ( 'NONE',  ( -82.39999999999999147, -33.29062499938548569, 103.1828516163667899 ) ) ;
#3665=CARTESIAN_POINT ( 'NONE',  ( -85.15643035624999868, -33.44062499938548427, -101.5914258081833879 ) ) ;
#3666=ORIENTED_EDGE ( 'NONE', *, *, #6947, .T. ) ;
#3667=CARTESIAN_POINT ( 'NONE',  ( 85.15643035624999868, -32.46562499938548996, 98.40857419181659793 ) ) ;
#3670=CARTESIAN_POINT ( 'NONE',  ( -79.64356964375001269, -31.22812499938548925, 98.40857419181659793 ) ) ;
#3671=CARTESIAN_POINT ( 'NONE',  ( -81.02178482187500208, -35.05312499938548854, 102.3871387122750889 ) ) ;
#3673=ORIENTED_EDGE ( 'NONE', *, *, #4882, .T. ) ;
#3674=CARTESIAN_POINT ( 'NONE',  ( -79.39999999999999147, -32.88750000000000284, -101.7320508075688821 ) ) ;
#3682=VECTOR ( 'NONE', #15107, 1000.000000000000000 ) ;
#3684=CARTESIAN_POINT ( 'NONE',  ( -82.40000000000001990, -32.75624999877096855, -103.0000000000000000 ) ) ;
#3685=CARTESIAN_POINT ( 'NONE',  ( -94.79999999999999716, -35.00000000000000000, -150.0000000000000000 ) ) ;
#3687=CARTESIAN_POINT ( 'NONE',  ( 81.02178482187500208, -30.85312499938548569, -97.61286128772489690 ) ) ;
#3688=DIRECTION ( 'NONE',  ( 0.000000000000000000, 0.000000000000000000, 1.000000000000000000 ) ) ;
#3690=VERTEX_POINT ( 'NONE', #17104 ) ;
#3695=VERTEX_POINT ( 'NONE', #6945 ) ;
#3697=CARTESIAN_POINT ( 'NONE',  ( -81.02178482187500208, -31.19062499938548427, -102.3871387122750889 ) ) ;
#3699=ORIENTED_EDGE ( 'NONE', *, *, #13345, .F. ) ;
#3700=CARTESIAN_POINT ( 'NONE',  ( 83.77821517812500929, -33.47812499938548569, 102.3871387122750889 ) ) ;
#3701=CARTESIAN_POINT ( 'NONE',  ( -80.90000000000000568, -33.69374999877096855, -102.5980762113533018 ) ) ;
#3702=AXIS2_PLACEMENT_3D ( 'NONE', #4457, #16477, #12071 ) ;
#3703=CARTESIAN_POINT ( 'NONE',  ( 82.39999999999999147, -34.61250000000000426, 103.4641016151377499 ) ) ;
#3707=CARTESIAN_POINT ( 'NONE',  ( 85.32499745258125756, -35.00000000000000711, -99.84129707245892860 ) ) ;
#3709=CARTESIAN_POINT ( 'NONE',  ( 82.40000000000000568, -30.00000000000000355, 96.99999999999998579 ) ) ;
#3712=CARTESIAN_POINT ( 'NONE',  ( 82.39999999999999147, -32.95312499938548711, -96.81714838363319586 ) ) ;
#3716=ORIENTED_EDGE ( 'NONE', *, *, #9335, .F. ) ;
#3718=CARTESIAN_POINT ( 'NONE',  ( -82.40000000000000568, -30.00000000000000355, 99.99999999999998579 ) ) ;
#3721=CARTESIAN_POINT ( 'NONE',  ( -85.40000000000000568, -33.99374999877097281, -99.99999999999998579 ) ) ;
#3725=CARTESIAN_POINT ( 'NONE',  ( 85.40000000000000568, -30.93750000000000355, -98.26794919243111792 ) ) ;
#3727=CARTESIAN_POINT ( 'NONE',  ( -85.40000000000000568, -34.89374999877097139, 99.99999999999998579 ) ) ;
#3731=CARTESIAN_POINT ( 'NONE',  ( 85.15643035625001289, -34.71562499938548285, -101.5914258081833879 ) ) ;
#3733=CARTESIAN_POINT ( 'NONE',  ( -79.64356964375001269, -34.37812499938548427, 98.40857419181659793 ) ) ;
#3735=ORIENTED_EDGE ( 'NONE', *, *, #10245, .T. ) ;
#3736=CARTESIAN_POINT ( 'NONE',  ( 82.39999999999999147, -32.81250000000000000, 103.0000000000000000 ) ) ;
#3737=CARTESIAN_POINT ( 'NONE',  ( -85.40000000000000568, -34.01250000000000284, 101.7320508075688679 ) ) ;
#3739=CARTESIAN_POINT ( 'NONE',  ( 82.39999999999999147, -33.48750000000000426, 97.00000000000000000 ) ) ;
#3742=ADVANCED_FACE ( 'NONE', ( #3806 ), #5585, .F. ) ;
#3745=CARTESIAN_POINT ( 'NONE',  ( 80.17984880387892588, -34.99999999999998579, 98.35655086105387568 ) ) ;
#3746=CARTESIAN_POINT ( 'NONE',  ( 85.15643035624999868, -32.87812499938549138, 101.5914258081833879 ) ) ;
#3752=CARTESIAN_POINT ( 'NONE',  ( 83.77821517812500929, -32.46562499938548285, 102.3871387122750889 ) ) ;
#3753=EDGE_CURVE ( 'NONE', #13349, #7832, #678, .T. ) ;
#3754=CARTESIAN_POINT ( 'NONE',  ( 85.15643035625001289, -30.14062499938548711, -99.99999999999998579 ) ) ;
#3756=CARTESIAN_POINT ( 'NONE',  ( -85.15643035625001289, -34.75312499938548427, 99.99999999999998579 ) ) ;
#3757=CARTESIAN_POINT ( 'NONE',  ( -82.39999999999999147, -31.82812499938548356, -96.81714838363319586 ) ) ;
#3759=ORIENTED_EDGE ( 'NONE', *, *, #3769, .F. ) ;
#3760=CARTESIAN_POINT ( 'NONE',  ( 85.15643035624999868, -32.01562499938548711, 98.40857419181659793 ) ) ;
#3763=CARTESIAN_POINT ( 'NONE',  ( -85.15643035624999868, -31.07812499938548356, 98.40857419181659793 ) ) ;
#3764=CARTESIAN_POINT ( 'NONE',  ( -85.15643035625001289, -34.75312499938548427, 99.99999999999998579 ) ) ;
#3765=CARTESIAN_POINT ( 'NONE',  ( 84.70388354820681798, -35.00002705695767702, 101.9214814096700934 ) ) ;
#3767=CARTESIAN_POINT ( 'NONE',  ( -85.40000000000000568, -33.14999999999999858, -99.99999999999998579 ) ) ;
#3769=EDGE_CURVE ( 'NONE', #8657, #13128, #11883, .T. ) ;
#3772=CARTESIAN_POINT ( 'NONE',  ( -83.04276107155152431, -35.00000000000000000, 97.06242906295996420 ) ) ;
#3773=CARTESIAN_POINT ( 'NONE',  ( -79.39999999999999147, -33.28124999877096712, -101.7320508075688963 ) ) ;
#3775=FACE_OUTER_BOUND ( 'NONE', #4438, .T. ) ;
#3778=CARTESIAN_POINT ( 'NONE',  ( 83.77821517812500929, -30.77812499938548640, -97.61286128772489690 ) ) ;
#3787=CARTESIAN_POINT ( 'NONE',  ( 85.40000000000000568, -34.05000000000000426, 99.99999999999998579 ) ) ;
#3789=CARTESIAN_POINT ( 'NONE',  ( -83.77821517812500929, -32.76562499938548711, -97.61286128772489690 ) ) ;
#3792=CARTESIAN_POINT ( 'NONE',  ( 82.39999999999999147, -33.51562499938548711, 103.1828516163667899 ) ) ;
#3793=CARTESIAN_POINT ( 'NONE',  ( -83.90000000000000568, -33.61874999877097281, -102.5980762113533018 ) ) ;
#3794=CARTESIAN_POINT ( 'NONE',  ( 79.39999999999999147, -34.68750000000000000, 101.7320508075688821 ) ) ;
#3798=CARTESIAN_POINT ( 'NONE',  ( -83.77821517812500929, -32.31562499938548427, -97.61286128772489690 ) ) ;
#3800=CARTESIAN_POINT ( 'NONE',  ( 96.99999999999997158, -5.200000000000003730, -150.0000000000000000 ) ) ;
#3804=CARTESIAN_POINT ( 'NONE',  ( 83.77821517812500929, -32.31562499938548427, -102.3871387122750889 ) ) ;
#3805=CARTESIAN_POINT ( 'NONE',  ( -82.39999999999999147, -34.97812499938547859, -96.81714838363319586 ) ) ;
#3806=FACE_OUTER_BOUND ( 'NONE', #2608, .T. ) ;
#3810=CARTESIAN_POINT ( 'NONE',  ( 81.59615242270663771, -32.11740381056766580, 96.99999999999998579 ) ) ;
#3811=ORIENTED_EDGE ( 'NONE', *, *, #8428, .T. ) ;
#3814=AXIS2_PLACEMENT_3D ( 'NONE', #11860, #1415, #9118 ) ;
#3817=CARTESIAN_POINT ( 'NONE',  ( 85.40000000000000568, -33.63750000000000284, -98.26794919243111792 ) ) ;
#3818=FACE_OUTER_BOUND ( 'NONE', #13329, .T. ) ;
#3819=CARTESIAN_POINT ( 'NONE',  ( -85.15643035625001289, -32.05312499938548854, 99.99999999999998579 ) ) ;
#3821=CARTESIAN_POINT ( 'NONE',  ( -69.99999999999998579, -35.00000000000000000, -150.0000000000000000 ) ) ;
#3823=CARTESIAN_POINT ( 'NONE',  ( 83.90000000000000568, -33.91874999877096997, 97.40192378864668399 ) ) ;
#3824=CARTESIAN_POINT ( 'NONE',  ( 80.90000000000000568, -33.89999999999999858, 97.40192378864668399 ) ) ;
#3825=CARTESIAN_POINT ( 'NONE',  ( -82.39999999999999147, -32.50312499938548427, 96.81714838363319586 ) ) ;
#3829=ORIENTED_EDGE ( 'NONE', *, *, #12104, .T. ) ;
#3830=CARTESIAN_POINT ( 'NONE',  ( 79.39999999999999147, -32.88750000000000284, 101.7320508075688963 ) ) ;
#3842=CARTESIAN_POINT ( 'NONE',  ( 85.15643035625001289, -33.29062499938547859, 99.99999999999998579 ) ) ;
#3844=ADVANCED_FACE ( 'NONE', ( #1151 ), #13149, .T. ) ;
#3845=CARTESIAN_POINT ( 'NONE',  ( 82.40000000000001990, -32.75624999877096855, -97.00000000000000000 ) ) ;
#3847=CARTESIAN_POINT ( 'NONE',  ( -85.15643035625001289, -34.34062499938548285, -101.5914258081833879 ) ) ;
#3848=CARTESIAN_POINT ( 'NONE',  ( 82.39999999999999147, -31.15312499938548640, 103.1828516163667899 ) ) ;
#3852=CARTESIAN_POINT ( 'NONE',  ( 83.77821517812500929, -33.77812499938548285, -102.3871387122750889 ) ) ;
#3854=CARTESIAN_POINT ( 'NONE',  ( -79.64356964374998427, -32.20312499938548711, 101.5914258081833879 ) ) ;
#3855=CARTESIAN_POINT ( 'NONE',  ( 79.64356964375001269, -30.77812499938548285, -98.40857419181659793 ) ) ;
#3857=CARTESIAN_POINT ( 'NONE',  ( 83.77821517812500929, -32.87812499938548427, 97.61286128772489690 ) ) ;
#3859=B_SPLINE_CURVE_WITH_KNOTS ( 'NONE', 3,
 ( #2044, #18466, #8003, #11520, #7122, #16109, #14245, #3893, #11325, #6742, #11226, #2615, #12885, #5281, #15915, #18758, #14531, #12689 ),
 .UNSPECIFIED., .F., .F.,
 ( 4, 2, 2, 2, 2, 2, 2, 2, 4 ),
 ( 0.000000000000000000, 0.0007106627595358718397, 0.001421325519071743679, 0.002131988278607615736, 0.002842651038143487359, 0.003553313797679358982, 0.004263976557215231472, 0.004974639316751103095, 0.005685302076286974718 ),
 .UNSPECIFIED. ) ;
#3861=CARTESIAN_POINT ( 'NONE',  ( -82.39999999999999147, -30.25312499938548783, 96.81714838363319586 ) ) ;
#3862=CARTESIAN_POINT ( 'NONE',  ( -83.77821517812500929, -30.96562499938548640, 102.3871387122750889 ) ) ;
#3865=CARTESIAN_POINT ( 'NONE',  ( -80.90000000000000568, -33.45000000000000284, -97.40192378864668399 ) ) ;
#3870=EDGE_CURVE ( 'NONE', #4219, #10782, #7908, .T. ) ;
#3872=CARTESIAN_POINT ( 'NONE',  ( -83.60689295392862164, -35.00000000000000000, 97.24646917567288540 ) ) ;
#3877=DIRECTION ( 'NONE',  ( 0.000000000000000000, -1.000000000000000000, 0.000000000000000000 ) ) ;
#3878=CARTESIAN_POINT ( 'NONE',  ( 85.15643035624999868, -34.71562499938548285, -101.5914258081833879 ) ) ;
#3879=CARTESIAN_POINT ( 'NONE',  ( -83.20384757729335945, -33.00134618820329990, 102.9999999999999858 ) ) ;
#3880=EDGE_LOOP ( 'NONE', ( #7043, #429, #14545, #8264 ) ) ;
#3881=CARTESIAN_POINT ( 'NONE',  ( 85.40000000000000568, -30.84374999877096712, 99.99999999999998579 ) ) ;
#3887=CARTESIAN_POINT ( 'NONE',  ( -82.39999999999999147, -30.70312499938548711, -103.1828516163667899 ) ) ;
#3890=CARTESIAN_POINT ( 'NONE',  ( 81.02178482187500208, -33.25312499938548427, 97.61286128772489690 ) ) ;
#3891=CARTESIAN_POINT ( 'NONE',  ( -79.64356964375001269, -31.86562499938548143, -98.40857419181659793 ) ) ;
#3892=CARTESIAN_POINT ( 'NONE',  ( 79.39999999999999147, -33.41250000000000142, 98.26794919243113213 ) ) ;
#3893=CARTESIAN_POINT ( 'NONE',  ( -80.48808202378405952, -34.99999999999999289, 97.80480077079599255 ) ) ;
#3895=B_SPLINE_CURVE_WITH_KNOTS ( 'NONE', 3,
 ( #16154, #7066, #18802, #10100, #12927, #8722, #6886, #5706, #4137, #4044 ),
 .UNSPECIFIED., .F., .F.,
 ( 4, 2, 2, 2, 4 ),
 ( 0.3612006186103786654, 0.3925526867148934063, 0.4239047548194081472, 0.4552568229239228881, 0.4866088910284376290 ),
 .UNSPECIFIED. ) ;
#3897=CARTESIAN_POINT ( 'NONE',  ( -85.15643035625001289, -32.35312499938548569, -98.40857419181659793 ) ) ;
#3900=CARTESIAN_POINT ( 'NONE',  ( -82.39999999999999147, -34.33124999877097139, 103.0000000000000000 ) ) ;
#3903=CARTESIAN_POINT ( 'NONE',  ( 79.64356964374999848, -32.16562499938548569, -99.99999999999998579 ) ) ;
#3908=CARTESIAN_POINT ( 'NONE',  ( 83.90000000000000568, -32.77499999999999858, 102.5980762113533018 ) ) ;
#3912=CARTESIAN_POINT ( 'NONE',  ( -82.40000000000000568, -34.10624999877096997, -102.9999999999999858 ) ) ;
#3915=VERTEX_POINT ( 'NONE', #6970 ) ;
#3918=CARTESIAN_POINT ( 'NONE',  ( 85.40000000000000568, -31.83750000000000568, -98.26794919243111792 ) ) ;
#3920=CARTESIAN_POINT ( 'NONE',  ( -81.02178482187500208, -30.55312499938548854, 102.3871387122750889 ) ) ;
#3922=CARTESIAN_POINT ( 'NONE',  ( -80.90000000000000568, -34.64999999999999858, -102.5980762113533018 ) ) ;
#3926=CARTESIAN_POINT ( 'NONE',  ( -79.39999999999999147, -33.73124999877096997, 98.26794919243110371 ) ) ;
#3930=ORIENTED_EDGE ( 'NONE', *, *, #695, .F. ) ;
#3933=CARTESIAN_POINT ( 'NONE',  ( -96.99999999999998579, -29.80000000000000426, -150.0000000000000000 ) ) ;
#3941=FACE_OUTER_BOUND ( 'NONE', #10610, .T. ) ;
#3942=CARTESIAN_POINT ( 'NONE',  ( 80.90000000000000568, -30.60000000000000142, 102.5980762113533018 ) ) ;
#3946=( BOUNDED_CURVE ( )  B_SPLINE_CURVE ( 2, ( #1852, #7810, #13765, #402, #8000, #7904, #4991, #16901, #15429, #2041, #18558, #17287, #3601, #14241, #6643, #14431, #12879, #6931, #14338, #1065, #18851, #17088, #14056, #784, #14150, #17379, #5173, #9759, #12590, #11418, #5374, #8103, #2233, #11120, #3890, #12975, #690, #7021, #976, #15722, #3700, #3792, #8387, #15627, #15819, #9667, #8199, #2427, #6739, #5473, #12685, #18946, #16989, #9857, #11223, #2328, #3992, #18658, #8474, #9958, #15912, #2517, #11026, #5277, #879, #8291, #17188, #6842, #12786, #9563, #15528, #18755, #11321, #2145, #14922, #14720, #2712, #19038, #1260, #4184, #2612, #16207, #17573 ),
 .UNSPECIFIED., .F., .F. ) 
 B_SPLINE_CURVE_WITH_KNOTS ( ( 3, 2, 2, 2, 2, 2, 2, 2, 2, 2, 2, 2, 2, 2, 2, 2, 2, 2, 2, 2, 2, 2, 2, 2, 2, 2, 2, 2, 2, 2, 2, 2, 2, 2, 2, 2, 2, 2, 2, 2, 2, 3 ),
 ( 0.3495698921800945436, 0.3600184345287981147, 0.3750192026341647167, 0.3900199707395312632, 0.4050207388448978651, 0.4200215069502644671, 0.4350222750556310691, 0.4500230431609976156, 0.4650238112663642176, 0.4800245793717307086, 0.4950253474770973661, 0.5100261155824639125, 0.5250268836878304590, 0.5400276517931971165, 0.5550284198985636630, 0.5700291880039303205, 0.5850299561092967560, 0.6000307242146634135, 0.6150314923200299599, 0.6300322604253966174, 0.6450330285307631639, 0.6600337966361298214, 0.6750345647414963679, 0.6900353328468629144, 0.7050361009522294609, 0.7200368690575960073, 0.7350376371629626648, 0.7500384052683293223, 0.7650391733736958688, 0.7800399414790624153, 0.7950407095844290728, 0.8100414776897955083, 0.8250422457951621658, 0.8400430139005288233, 0.8550437820058953697, 0.8700445501112619162, 0.8850453182166284627, 0.9000460863219952312, 0.9150468544273615557, 0.9300476225327283242, 0.9450483906380948707, 0.9496006163947576795 ),
 .UNSPECIFIED. ) 
 CURVE ( )  GEOMETRIC_REPRESENTATION_ITEM ( )  RATIONAL_B_SPLINE_CURVE ( ( 0.9433623850486869689, 0.9066821623815414233, 1.000000000000000000, 0.8660254037844387076, 1.000000000000000000, 0.8660254037844387076, 1.000000000000000000, 0.8660254037844387076, 1.000000000000000000, 0.8660254037844387076, 1.000000000000000000, 0.8660254037844387076, 1.000000000000000000, 0.8660254037844387076, 1.000000000000000000, 0.8660254037844387076, 1.000000000000000000, 0.8660254037844387076, 1.000000000000000000, 0.8660254037844387076, 1.000000000000000000, 0.8660254037844387076, 1.000000000000000000, 0.8660254037844387076, 1.000000000000000000, 0.8660254037844387076, 1.000000000000000000, 0.8660254037844387076, 1.000000000000000000, 0.8660254037844387076, 1.000000000000000000, 0.8660254037844387076, 1.000000000000000000, 0.8660254037844387076, 1.000000000000000000, 0.8660254037844387076, 1.000000000000000000, 0.8660254037844387076, 1.000000000000000000, 0.8660254037844387076, 1.000000000000000000, 0.8660254037844387076, 1.000000000000000000, 0.8660254037844387076, 1.000000000000000000, 0.8660254037844387076, 1.000000000000000000, 0.8660254037844387076, 1.000000000000000000, 0.8660254037844387076, 1.000000000000000000, 0.8660254037844387076, 1.000000000000000000, 0.8660254037844387076, 1.000000000000000000, 0.8660254037844387076, 1.000000000000000000, 0.8660254037844387076, 1.000000000000000000, 0.8660254037844387076, 1.000000000000000000, 0.8660254037844387076, 1.000000000000000000, 0.8660254037844387076, 1.000000000000000000, 0.8660254037844387076, 1.000000000000000000, 0.8660254037844387076, 1.000000000000000000, 0.8660254037844387076, 1.000000000000000000, 0.8660254037844387076, 1.000000000000000000, 0.8660254037844387076, 1.000000000000000000, 0.8660254037844387076, 1.000000000000000000, 0.8660254037844387076, 1.000000000000000000, 0.8660254037844387076, 1.000000000000000000, 0.9593432414028981725, 0.9433623850486876350 ) ) 
 REPRESENTATION_ITEM ( '' )  );
#3948=CARTESIAN_POINT ( 'NONE',  ( -83.77821517812500929, -34.67812499938548854, -97.61286128772489690 ) ) ;
#3949=CARTESIAN_POINT ( 'NONE',  ( 82.39999999999999147, -32.27812499938548285, 96.81714838363319586 ) ) ;
#3951=CARTESIAN_POINT ( 'NONE',  ( 83.77821517812500929, -33.02812499938548285, -97.61286128772489690 ) ) ;
#3953=CARTESIAN_POINT ( 'NONE',  ( -85.15643035625001289, -33.74062499938548854, 99.99999999999998579 ) ) ;
#3954=CARTESIAN_POINT ( 'NONE',  ( 81.02178482187500208, -31.34062499938548996, -102.3871387122750889 ) ) ;
#3956=CARTESIAN_POINT ( 'NONE',  ( 79.64356964375001269, -34.94062499938549138, 101.5914258081833879 ) ) ;
#3959=CARTESIAN_POINT ( 'NONE',  ( -79.64356964375001269, -33.10312499938549280, 101.5914258081833879 ) ) ;
#3960=CARTESIAN_POINT ( 'NONE',  ( -79.64356964374999848, -31.71562499938548285, 99.99999999999998579 ) ) ;
#3966=VECTOR ( 'NONE', #6825, 1000.000000000000000 ) ;
#3970=CARTESIAN_POINT ( 'NONE',  ( -79.39999999999999147, -32.38124999877096855, -101.7320508075688963 ) ) ;
#3974=CARTESIAN_POINT ( 'NONE',  ( -82.40000000000000568, -30.00000000000000355, 103.0000000000000000 ) ) ;
#3975=CARTESIAN_POINT ( 'NONE',  ( 79.64356964375001269, -34.94062499938549138, -98.40857419181659793 ) ) ;
#3978=EDGE_CURVE ( 'NONE', #15550, #2447, #4545, .T. ) ;
#3980=CARTESIAN_POINT ( 'NONE',  ( 79.39999999999999147, -32.41874999877096997, 99.99999999999998579 ) ) ;
#3985=CARTESIAN_POINT ( 'NONE',  ( 85.40000000000000568, -34.53750000000000142, 101.7320508075688821 ) ) ;
#3986=LINE ( 'NONE', #14426, #6820 ) ;
#3988=CARTESIAN_POINT ( 'NONE',  ( -85.15643035625001289, -32.39062499938548711, -99.99999999999998579 ) ) ;
#3989=DIRECTION ( 'NONE',  ( -0.000000000000000000, -0.000000000000000000, -1.000000000000000000 ) ) ;
#3991=ORIENTED_EDGE ( 'NONE', *, *, #7428, .T. ) ;
#3992=CARTESIAN_POINT ( 'NONE',  ( 79.64356964374999848, -34.07812499938548711, 99.99999999999998579 ) ) ;
#3994=CARTESIAN_POINT ( 'NONE',  ( -85.40000000000000568, -35.36739044046696279, -101.0919052301551204 ) ) ;
#3995=CARTESIAN_POINT ( 'NONE',  ( 85.40000000000000568, -33.60000000000000142, 99.99999999999998579 ) ) ;
#3996=CARTESIAN_POINT ( 'NONE',  ( 81.59615242270662350, -34.57634618820329564, -96.99999999999997158 ) ) ;
#4000=CARTESIAN_POINT ( 'NONE',  ( -83.77821517812500929, -32.01562499938548001, -102.3871387122750889 ) ) ;
#4003=CARTESIAN_POINT ( 'NONE',  ( 85.40000000000000568, -31.74374999877096926, -99.99999999999998579 ) ) ;
#4005=EDGE_CURVE ( 'NONE', #13667, #13807, #12725, .T. ) ;
#4006=VERTEX_POINT ( 'NONE', #15154 ) ;
#4015=ORIENTED_EDGE ( 'NONE', *, *, #15676, .T. ) ;
#4019=DIRECTION ( 'NONE',  ( -1.000000000000000000, 4.625929269271494788E-16, 0.000000000000000000 ) ) ;
#4022=CARTESIAN_POINT ( 'NONE',  ( 83.90000000000000568, -32.77499999999999858, -97.40192378864668399 ) ) ;
#4023=CARTESIAN_POINT ( 'NONE',  ( 80.24533121543018410, -31.99999999999997868, -102.0417045141622339 ) ) ;
#4024=CARTESIAN_POINT ( 'NONE',  ( -82.39999999999999147, -31.94062499938548427, 103.1828516163667899 ) ) ;
#4026=EDGE_CURVE ( 'NONE', #17606, #11560, #10534, .T. ) ;
#4027=DIRECTION ( 'NONE',  ( -0.000000000000000000, -1.000000000000000000, -0.000000000000000000 ) ) ;
#4028=LINE ( 'NONE', #11731, #2567 ) ;
#4029=CARTESIAN_POINT ( 'NONE',  ( 81.02178482187500208, -34.45312499938548711, -97.61286128772489690 ) ) ;
#4031=CARTESIAN_POINT ( 'NONE',  ( -82.39999999999999147, -34.97812499938547859, 103.1828516163667899 ) ) ;
#4032=LINE ( 'NONE', #2365, #11774 ) ;
#4033=EDGE_LOOP ( 'NONE', ( #14337, #18163, #9294, #4682 ) ) ;
#4036=DIRECTION ( 'NONE',  ( 0.000000000000000000, 0.000000000000000000, -1.000000000000000000 ) ) ;
#4040=EDGE_CURVE ( 'NONE', #1717, #7460, #6182, .T. ) ;
#4042=ORIENTED_EDGE ( 'NONE', *, *, #9244, .F. ) ;
#4044=CARTESIAN_POINT ( 'NONE',  ( -84.70388354820684640, -35.00002705695768412, -101.9214814096701076 ) ) ;
#4045=CARTESIAN_POINT ( 'NONE',  ( 85.15643035624999868, -34.67812499938548143, 101.5914258081833879 ) ) ;
#4050=CARTESIAN_POINT ( 'NONE',  ( -82.39999999999999147, -34.41562499938548569, -103.1828516163667899 ) ) ;
#4051=CARTESIAN_POINT ( 'NONE',  ( 85.15643035624999868, -33.25312499938548427, 98.40857419181659793 ) ) ;
#4052=CARTESIAN_POINT ( 'NONE',  ( 79.64356964375001269, -34.04062499938549280, -98.40857419181659793 ) ) ;
#4054=CARTESIAN_POINT ( 'NONE',  ( -81.02178482187500208, -33.89062499938548711, 97.61286128772489690 ) ) ;
#4055=CARTESIAN_POINT ( 'NONE',  ( 85.15643035625001289, -31.04062499938548569, -99.99999999999998579 ) ) ;
#4060=CARTESIAN_POINT ( 'NONE',  ( -82.39999999999999147, -34.07812499938548711, 103.1828516163667899 ) ) ;
#4061=CARTESIAN_POINT ( 'NONE',  ( -85.15643035625001289, -30.59062499938548285, 99.99999999999998579 ) ) ;
#4065=( BOUNDED_CURVE ( )  B_SPLINE_CURVE ( 2, ( #5298, #11440, #11244, #18481, #3721, #9782, #18774, #17306, #3912 ),
 .UNSPECIFIED., .F., .F. ) 
 B_SPLINE_CURVE_WITH_KNOTS ( ( 3, 2, 2, 2, 3 ),
 ( 0.6458333333333333703, 0.6527777777777777901, 0.6666666666666666297, 0.6805555555555555802, 0.6875000000000000000 ),
 .UNSPECIFIED. ) 
 CURVE ( )  GEOMETRIC_REPRESENTATION_ITEM ( )  RATIONAL_B_SPLINE_CURVE ( ( 0.9330127018922192983, 0.9330127018922198534, 1.000000000000000000, 0.8660254037844387076, 1.000000000000000000, 0.8660254037844387076, 1.000000000000000000, 0.9330127018922194093, 0.9330127018922194093 ) ) 
 REPRESENTATION_ITEM ( '' )  );
#4069=CARTESIAN_POINT ( 'NONE',  ( -85.40000000000000568, -34.93124999877096570, 98.26794919243111792 ) ) ;
#4070=CARTESIAN_POINT ( 'NONE',  ( -80.90000000000000568, -33.39374999877097139, -97.40192378864668399 ) ) ;
#4072=CARTESIAN_POINT ( 'NONE',  ( 79.64356964375001269, -30.44062499938548783, 101.5914258081833879 ) ) ;
#4073=CARTESIAN_POINT ( 'NONE',  ( -83.20395887649183919, -35.00000000000001421, -97.36341917746362640 ) ) ;
#4074=CARTESIAN_POINT ( 'NONE',  ( -85.40000000000000568, -32.68124999877097281, -101.7320508075688821 ) ) ;
#4075=CARTESIAN_POINT ( 'NONE',  ( 82.39999999999999147, -34.19062499938548427, -103.1828516163667899 ) ) ;
#4076=CARTESIAN_POINT ( 'NONE',  ( -85.40000000000000568, -33.05624999877097281, 101.7320508075688821 ) ) ;
#4078=CARTESIAN_POINT ( 'NONE',  ( 85.40000000000000568, -33.95624999877097139, 98.26794919243111792 ) ) ;
#4083=EDGE_LOOP ( 'NONE', ( #12988, #12112, #208, #13069 ) ) ;
#4084=CARTESIAN_POINT ( 'NONE',  ( -83.77821517812500929, -33.21562499938548285, -97.61286128772489690 ) ) ;
#4086=EDGE_LOOP ( 'NONE', ( #9878, #19172, #19075, #15593 ) ) ;
#4088=CARTESIAN_POINT ( 'NONE',  ( -85.15643035624999868, -32.01562499938548711, -98.40857419181659793 ) ) ;
#4089=CARTESIAN_POINT ( 'NONE',  ( 82.39999999999999147, -33.48750000000000426, 96.53589838486223584 ) ) ;
#4093=CARTESIAN_POINT ( 'NONE',  ( -81.02178482187500208, -33.14062499938548711, -97.61286128772489690 ) ) ;
#4094=EDGE_CURVE ( 'NONE', #10447, #14621, #17807, .T. ) ;
#4096=CARTESIAN_POINT ( 'NONE',  ( 85.40000000000000568, -31.29374999877096997, -99.99999999999998579 ) ) ;
#4100=ORIENTED_EDGE ( 'NONE', *, *, #4005, .T. ) ;
#4107=ORIENTED_EDGE ( 'NONE', *, *, #7315, .F. ) ;
#4113=CARTESIAN_POINT ( 'NONE',  ( 79.39999999999999147, -32.02500000000000568, -99.99999999999998579 ) ) ;
#4116=CARTESIAN_POINT ( 'NONE',  ( -83.77821517812500929, -30.62812499938548783, 102.3871387122750889 ) ) ;
#4118=CARTESIAN_POINT ( 'NONE',  ( -79.39999999999999147, -34.72500000000000142, -99.99999999999998579 ) ) ;
#4121=CARTESIAN_POINT ( 'NONE',  ( 94.79999999999991189, -3.000000000000000000, 150.0000000000000000 ) ) ;
#4122=CARTESIAN_POINT ( 'NONE',  ( 85.23110191009456571, -35.00000000000000000, 100.8575180188180269 ) ) ;
#4123=CARTESIAN_POINT ( 'NONE',  ( 85.15643035624999868, -35.11426555956768425, -98.99674139749697588 ) ) ;
#4124=ORIENTED_EDGE ( 'NONE', *, *, #3421, .T. ) ;
#4125=FILL_AREA_STYLE ('',( #13106 ) ) ;
#4126=CARTESIAN_POINT ( 'NONE',  ( -85.15643035624999868, -31.90312499938548285, -98.40857419181659793 ) ) ;
#4127=LINE ( 'NONE', #14187, #880 ) ;
#4128=AXIS2_PLACEMENT_3D ( 'NONE', #18082, #3022, #12010 ) ;
#4133=CARTESIAN_POINT ( 'NONE',  ( 110.9999999999999574, -21.80000000000003268, -137.3499999999999943 ) ) ;
#4137=CARTESIAN_POINT ( 'NONE',  ( -84.57144699476174310, -35.00000000000000000, -102.0792695867486657 ) ) ;
#4138=CARTESIAN_POINT ( 'NONE',  ( 85.40000000000000568, -30.45000000000000284, 99.99999999999998579 ) ) ;
#4139=CARTESIAN_POINT ( 'NONE',  ( 96.99999999999994316, -21.80000000000003268, -142.6499999999999773 ) ) ;
#4143=CARTESIAN_POINT ( 'NONE',  ( 82.40000000000000568, -30.00000000000000355, 103.0000000000000000 ) ) ;
#4146=CARTESIAN_POINT ( 'NONE',  ( -85.15643035625001289, -33.36562499938548854, -98.40857419181659793 ) ) ;
#4148=CARTESIAN_POINT ( 'NONE',  ( 83.77821517812500929, -34.22812499938549280, -102.3871387122750889 ) ) ;
#4150=CARTESIAN_POINT ( 'NONE',  ( -82.39999999999999147, -34.30312499938548143, 96.81714838363319586 ) ) ;
#4151=CARTESIAN_POINT ( 'NONE',  ( 85.15643035624999868, -30.55312499938548854, -101.5914258081833879 ) ) ;
#4153=CARTESIAN_POINT ( 'NONE',  ( 85.15643035625001289, -35.22676544108147567, 101.0032535741825654 ) ) ;
#4155=EDGE_CURVE ( 'NONE', #6638, #14213, #1885, .T. ) ;
#4157=VECTOR ( 'NONE', #16971, 1000.000000000000000 ) ;
#4158=( BOUNDED_CURVE ( )  B_SPLINE_CURVE ( 2, ( #12461, #1911, #3473, #4666, #10615, #15399, #16867, #3184, #16674 ),
 .UNSPECIFIED., .F., .F. ) 
 B_SPLINE_CURVE_WITH_KNOTS ( ( 3, 2, 2, 2, 3 ),
 ( 0.4791666666666666297, 0.4861111111111111049, 0.5000000000000000000, 0.5138888888888888395, 0.5208333333333334814 ),
 .UNSPECIFIED. ) 
 CURVE ( )  GEOMETRIC_REPRESENTATION_ITEM ( )  RATIONAL_B_SPLINE_CURVE ( ( 0.9330127018922194093, 0.9330127018922190762, 1.000000000000000000, 0.8660254037844387076, 1.000000000000000000, 0.8660254037844387076, 1.000000000000000000, 0.9330127018922177440, 0.9330127018922194093 ) ) 
 REPRESENTATION_ITEM ( '' )  );
#4159=CARTESIAN_POINT ( 'NONE',  ( -82.39999999999999147, -32.27812499938548285, 103.1828516163667899 ) ) ;
#4160=CARTESIAN_POINT ( 'NONE',  ( -83.77821517812500929, -31.86562499938548498, 102.3871387122750889 ) ) ;
#4161=ORIENTED_EDGE ( 'NONE', *, *, #1374, .T. ) ;
#4162=CARTESIAN_POINT ( 'NONE',  ( -83.20384757729335945, -34.08615380933863293, 96.99999999999998579 ) ) ;
#4165=CARTESIAN_POINT ( 'NONE',  ( 83.20384757729335945, -33.69240381056766154, -96.99999999999998579 ) ) ;
#4170=CARTESIAN_POINT ( 'NONE',  ( 83.77821517812500929, -33.47812499938548569, 102.3871387122750889 ) ) ;
#4172=CARTESIAN_POINT ( 'NONE',  ( 82.39999999999999147, -32.84062499938548996, -103.1828516163667899 ) ) ;
#4173=ORIENTED_EDGE ( 'NONE', *, *, #13656, .T. ) ;
#4174=CARTESIAN_POINT ( 'NONE',  ( 79.39999999999999147, -31.96874999877096712, 99.99999999999998579 ) ) ;
#4178=DIRECTION ( 'NONE',  ( 1.000000000000000000, -0.000000000000000000, -2.407412430484046130E-31 ) ) ;
#4179=CARTESIAN_POINT ( 'NONE',  ( -84.44763168836716716, -32.00000000000000000, 101.8452947671445799 ) ) ;
#4180=ORIENTED_EDGE ( 'NONE', *, *, #17417, .T. ) ;
#4181=CARTESIAN_POINT ( 'NONE',  ( -82.39999999999999147, -34.75312499938549138, -103.1828516163667899 ) ) ;
#4184=CARTESIAN_POINT ( 'NONE',  ( 79.64356964374998427, -34.94062499938548427, 101.5914258081833879 ) ) ;
#4185=CARTESIAN_POINT ( 'NONE',  ( -85.15643035625001289, -30.70312499938548711, -99.99999999999998579 ) ) ;
#4186=CARTESIAN_POINT ( 'NONE',  ( -83.90000000000000568, -30.91874999877096997, -102.5980762113533018 ) ) ;
#4187=DIRECTION ( 'NONE',  ( -0.000000000000000000, 1.000000000000000000, -0.000000000000000000 ) ) ;
#4190=CARTESIAN_POINT ( 'NONE',  ( -84.28136653320150629, -32.00000000000001421, -102.0145392219080378 ) ) ;
#4192=CARTESIAN_POINT ( 'NONE',  ( 80.90000000000000568, -32.79374999877096997, -97.40192378864668399 ) ) ;
#4194=ORIENTED_EDGE ( 'NONE', *, *, #16083, .T. ) ;
#4195=CARTESIAN_POINT ( 'NONE',  ( 81.02178482187500208, -34.79062499938548569, -97.61286128772489690 ) ) ;
#4199=CARTESIAN_POINT ( 'NONE',  ( 84.44763168836732348, -32.00000000000002132, 98.15470523285560489 ) ) ;
#4201=VERTEX_POINT ( 'NONE', #5193 ) ;
#4205=ORIENTED_EDGE ( 'NONE', *, *, #14141, .T. ) ;
#4206=CARTESIAN_POINT ( 'NONE',  ( 79.39999999999999147, -32.38124999877096855, -98.26794919243110371 ) ) ;
#4207=CARTESIAN_POINT ( 'NONE',  ( 85.40000000000000568, -33.56250000000000000, -101.7320508075688679 ) ) ;
#4208=DIRECTION ( 'NONE',  ( 0.000000000000000000, 0.000000000000000000, -1.000000000000000000 ) ) ;
#4210=ADVANCED_FACE ( 'NONE', ( #13975 ), #1870, .F. ) ;
#4211=CARTESIAN_POINT ( 'NONE',  ( -85.15643035624999868, -32.01562499938548711, 101.5914258081833879 ) ) ;
#4216=CARTESIAN_POINT ( 'NONE',  ( 80.03686793005718414, -35.00000000000000000, 101.6462804658012828 ) ) ;
#4217=PLANE ( 'NONE',  #7427 ) ;
#4219=VERTEX_POINT ( 'NONE', #15445 ) ;
#4220=CARTESIAN_POINT ( 'NONE',  ( -82.39999999999999147, -30.47812499938548569, -96.81714838363319586 ) ) ;
#4230=ORIENTED_EDGE ( 'NONE', *, *, #3662, .T. ) ;
#4232=CARTESIAN_POINT ( 'NONE',  ( -84.44763168836716716, -32.00000000000000000, 101.8452947671445799 ) ) ;
#4235=CARTESIAN_POINT ( 'NONE',  ( -80.90000000000000568, -33.89999999999999858, -97.40192378864668399 ) ) ;
#4236=CARTESIAN_POINT ( 'NONE',  ( 85.15643035624999868, -33.77812499938548285, 101.5914258081833879 ) ) ;
#4237=DIRECTION ( 'NONE',  ( 1.000000000000000000, 0.000000000000000000, -0.000000000000000000 ) ) ;
#4242=CARTESIAN_POINT ( 'NONE',  ( 85.40000000000000568, -33.13124999877096855, -98.26794919243111792 ) ) ;
#4243=CARTESIAN_POINT ( 'NONE',  ( 82.39999999999999147, -31.60312499938548569, -96.81714838363319586 ) ) ;
#4246=CARTESIAN_POINT ( 'NONE',  ( -81.02178482187500208, -32.54062499938548569, 97.61286128772489690 ) ) ;
#4247=CARTESIAN_POINT ( 'NONE',  ( 85.15643035625001289, -30.59062499938548285, -99.99999999999998579 ) ) ;
#4249=CARTESIAN_POINT ( 'NONE',  ( 85.15643035624999868, -34.26562499938548711, 98.40857419181659793 ) ) ;
#4250=CARTESIAN_POINT ( 'NONE',  ( -80.90000000000000568, -34.74374999877097281, 102.5980762113533018 ) ) ;
#4253=CARTESIAN_POINT ( 'NONE',  ( -79.64356964375001269, -34.45312499938548711, 101.5914258081833879 ) ) ;
#4254=ORIENTED_EDGE ( 'NONE', *, *, #9335, .T. ) ;
#4257=CARTESIAN_POINT ( 'NONE',  ( 79.60045861139944634, -34.99999999999999289, -99.68825842090971889 ) ) ;
#4261=CARTESIAN_POINT ( 'NONE',  ( -80.90000000000000568, -32.34374999877096712, 97.40192378864668399 ) ) ;
#4263=CARTESIAN_POINT ( 'NONE',  ( -79.39999999999999147, -32.41874999877096997, -99.99999999999998579 ) ) ;
#4264=CARTESIAN_POINT ( 'NONE',  ( 81.02178482187500208, -32.20312499938548711, 102.3871387122750889 ) ) ;
#4265=CARTESIAN_POINT ( 'NONE',  ( -99.99999999999998579, 0.000000000000000000, 150.0000000000000000 ) ) ;
#4266=CARTESIAN_POINT ( 'NONE',  ( 79.64356964374999848, -34.07812499938548711, -99.99999999999998579 ) ) ;
#4267=FACE_OUTER_BOUND ( 'NONE', #4810, .T. ) ;
#4268=( BOUNDED_CURVE ( )  B_SPLINE_CURVE ( 2, ( #12258, #13332, #4447, #9317, #17932, #7658, #10499, #1617, #18036 ),
 .UNSPECIFIED., .F., .F. ) 
 B_SPLINE_CURVE_WITH_KNOTS ( ( 3, 2, 2, 2, 3 ),
 ( 0.7708333333333332593, 0.7777777777777777901, 0.7916666666666666297, 0.8055555555555555802, 0.8125000000000000000 ),
 .UNSPECIFIED. ) 
 CURVE ( )  GEOMETRIC_REPRESENTATION_ITEM ( )  RATIONAL_B_SPLINE_CURVE ( ( 0.9330127018922192983, 0.9330127018922187432, 1.000000000000000000, 0.8660254037844387076, 1.000000000000000000, 0.8660254037844387076, 1.000000000000000000, 0.9330127018922194093, 0.9330127018922194093 ) ) 
 REPRESENTATION_ITEM ( '' )  );
#4269=ORIENTED_EDGE ( 'NONE', *, *, #11640, .T. ) ;
#4270=CARTESIAN_POINT ( 'NONE',  ( 82.39999999999999147, -34.10624999877096997, 103.4641016151377499 ) ) ;
#4276=CARTESIAN_POINT ( 'NONE',  ( -81.02178482187500208, -33.14062499938548711, -97.61286128772489690 ) ) ;
#4280=CARTESIAN_POINT ( 'NONE',  ( 99.99999999999997158, -5.200000000000008171, 150.0000000000000000 ) ) ;
#4281=CARTESIAN_POINT ( 'NONE',  ( -82.39999999999999147, -35.23124999877096997, -96.53589838486223584 ) ) ;
#4283=CARTESIAN_POINT ( 'NONE',  ( -82.39999999999999147, -31.18124999877096926, -96.53589838486223584 ) ) ;
#4291=CARTESIAN_POINT ( 'NONE',  ( 83.90000000000000568, -30.76874999877097139, -102.5980762113533018 ) ) ;
#4295=EDGE_LOOP ( 'NONE', ( #18241, #4301, #3641, #18199 ) ) ;
#4301=ORIENTED_EDGE ( 'NONE', *, *, #15701, .T. ) ;
#4307=CARTESIAN_POINT ( 'NONE',  ( 82.39999999999999147, -34.38750000000000284, -103.4641016151377499 ) ) ;
#4311=CARTESIAN_POINT ( 'NONE',  ( -79.64356964375001269, -34.56562499938549138, 101.5914258081833879 ) ) ;
#4316=CARTESIAN_POINT ( 'NONE',  ( 79.67114894419049165, -35.00000000000001421, 100.7768843408770181 ) ) ;
#4317=CARTESIAN_POINT ( 'NONE',  ( 84.06832524826147335, -34.99999999999999289, 97.74327260033980735 ) ) ;
#4318=CARTESIAN_POINT ( 'NONE',  ( -85.40000000000000568, -34.46249999999999858, -98.26794919243111792 ) ) ;
#4319=ORIENTED_EDGE ( 'NONE', *, *, #11532, .F. ) ;
#4320=SURFACE_SIDE_STYLE ('',( #14561 ) ) ;
#4321=CARTESIAN_POINT ( 'NONE',  ( -79.64356964374999848, -30.81562499938548427, -99.99999999999998579 ) ) ;
#4323=VECTOR ( 'NONE', #18883, 1000.000000000000000 ) ;
#4325=CARTESIAN_POINT ( 'NONE',  ( -83.20384757729337366, -32.55134618820330417, 103.0000000000000000 ) ) ;
#4327=CARTESIAN_POINT ( 'NONE',  ( 82.39999999999999147, -32.81250000000000000, 103.0000000000000000 ) ) ;
#4329=EDGE_LOOP ( 'NONE', ( #10415, #13849, #5051, #7916 ) ) ;
#4331=CARTESIAN_POINT ( 'NONE',  ( -84.74067385206564040, -32.00000000000000711, 98.53339280468568973 ) ) ;
#4333=CARTESIAN_POINT ( 'NONE',  ( 82.40000000000000568, -32.08124999877097139, -102.9999999999999858 ) ) ;
#4334=CARTESIAN_POINT ( 'NONE',  ( 83.77821517812500929, -33.81562499938548427, 102.3871387122750889 ) ) ;
#4338=PLANE ( 'NONE',  #3649 ) ;
#4339=CARTESIAN_POINT ( 'NONE',  ( 81.02178482187500208, -34.34062499938548285, 102.3871387122750889 ) ) ;
#4340=CARTESIAN_POINT ( 'NONE',  ( 85.15643035624999868, -30.55312499938548854, -101.5914258081833879 ) ) ;
#4343=CARTESIAN_POINT ( 'NONE',  ( 85.15643035625001289, -33.29062499938547859, -99.99999999999998579 ) ) ;
#4349=CARTESIAN_POINT ( 'NONE',  ( -81.02178482187500208, -33.89062499938548711, 97.61286128772489690 ) ) ;
#4352=CARTESIAN_POINT ( 'NONE',  ( 82.39999999999999147, -32.98124999877096286, -102.9999999999999858 ) ) ;
#4356=CARTESIAN_POINT ( 'NONE',  ( 82.39999999999999147, -34.33124999877097139, -103.0000000000000000 ) ) ;
#4359=CARTESIAN_POINT ( 'NONE',  ( -79.39999999999999147, -32.51250000000000284, 101.7320508075688537 ) ) ;
#4360=CARTESIAN_POINT ( 'NONE',  ( 82.39999999999999147, -32.16562499938549280, 103.1828516163667899 ) ) ;
#4361=ADVANCED_FACE ( 'NONE', ( #4815 ), #14168, .F. ) ;
#4362=CARTESIAN_POINT ( 'NONE',  ( -85.40000000000000568, -32.70000000000000284, 99.99999999999998579 ) ) ;
#4364=CARTESIAN_POINT ( 'NONE',  ( -82.39999999999999147, -32.16562499938548569, 96.81714838363319586 ) ) ;
#4365=CARTESIAN_POINT ( 'NONE',  ( -85.15643035624999868, -30.74062499938548143, -101.5914258081833879 ) ) ;
#4366=ORIENTED_EDGE ( 'NONE', *, *, #1350, .T. ) ;
#4367=CARTESIAN_POINT ( 'NONE',  ( 85.40000000000000568, -33.13124999877096855, 101.7320508075688679 ) ) ;
#4370=CARTESIAN_POINT ( 'NONE',  ( -82.39999999999999147, -31.94062499938548427, 103.1828516163667899 ) ) ;
#4374=CARTESIAN_POINT ( 'NONE',  ( -81.02178482187500208, -34.34062499938548285, -102.3871387122750889 ) ) ;
#4376=ORIENTED_EDGE ( 'NONE', *, *, #1121, .F. ) ;
#4378=CARTESIAN_POINT ( 'NONE',  ( -79.64356964375001269, -32.69062499938548427, -101.5914258081833879 ) ) ;
#4379=CARTESIAN_POINT ( 'NONE',  ( -79.68063642052034368, -32.00000000000000711, -101.2652131117249752 ) ) ;
#4380=CARTESIAN_POINT ( 'NONE',  ( -79.39999999999999147, -31.55624999877096926, -98.26794919243113213 ) ) ;
#4384=CARTESIAN_POINT ( 'NONE',  ( -83.77821517812500929, -34.71562499938548285, -102.3871387122750889 ) ) ;
#4388=CARTESIAN_POINT ( 'NONE',  ( 85.40000000000000568, -32.60624999877097707, -101.7320508075688679 ) ) ;
#4397=VERTEX_POINT ( 'NONE', #992 ) ;
#4399=CARTESIAN_POINT ( 'NONE',  ( -79.39999999999999147, -32.06250000000000000, 101.7320508075688537 ) ) ;
#4405=CARTESIAN_POINT ( 'NONE',  ( -82.39999999999999147, -33.29062499938549280, 103.1828516163667899 ) ) ;
#4409=CARTESIAN_POINT ( 'NONE',  ( 80.85389467647095785, -34.99999999999999289, 102.4890844034575395 ) ) ;
#4410=CARTESIAN_POINT ( 'NONE',  ( -79.59365286754817248, -34.99999999999999289, -100.0710144471396177 ) ) ;
#4412=ORIENTED_EDGE ( 'NONE', *, *, #4702, .F. ) ;
#4414=CARTESIAN_POINT ( 'NONE',  ( -79.64356964375001269, -31.22812499938548925, -101.5914258081833879 ) ) ;
#4416=CARTESIAN_POINT ( 'NONE',  ( 82.40000000000000568, -30.00000000000000355, -103.0000000000000000 ) ) ;
#4419=LINE ( 'NONE', #4133, #6938 ) ;
#4425=CARTESIAN_POINT ( 'NONE',  ( -80.90000000000000568, -31.44374999877096855, 97.40192378864668399 ) ) ;
#4426=CARTESIAN_POINT ( 'NONE',  ( 85.40000000000000568, -33.11250000000000426, 98.26794919243111792 ) ) ;
#4427=CARTESIAN_POINT ( 'NONE',  ( -79.68596062386970402, -32.00000000000002132, -98.72172371342720965 ) ) ;
#4429=CARTESIAN_POINT ( 'NONE',  ( 85.40000000000000568, -32.19374999877096855, 99.99999999999998579 ) ) ;
#4430=CARTESIAN_POINT ( 'NONE',  ( 83.77821517812500929, -33.66562499938548569, 97.61286128772489690 ) ) ;
#4432=CIRCLE ( 'NONE', #15351, 5.199999999999996625 ) ;
#4433=CARTESIAN_POINT ( 'NONE',  ( 79.64356964375001269, -31.75312499938548427, -101.5914258081833879 ) ) ;
#4434=EDGE_LOOP ( 'NONE', ( #9114, #12294, #4015, #3573 ) ) ;
#4436=CARTESIAN_POINT ( 'NONE',  ( 79.39999999999999147, -34.18124999877097281, 101.7320508075688963 ) ) ;
#4437=CARTESIAN_POINT ( 'NONE',  ( 83.77821517812500929, -33.66562499938548569, -102.3871387122750889 ) ) ;
#4438=EDGE_LOOP ( 'NONE', ( #15524, #15428, #18260, #13925 ) ) ;
#4439=CARTESIAN_POINT ( 'NONE',  ( -82.40000000000000568, -32.00000000000000000, 99.99999999999998579 ) ) ;
#4442=CARTESIAN_POINT ( 'NONE',  ( -85.40000000000000568, -30.00000000000000355, 99.99999999999998579 ) ) ;
#4446=VECTOR ( 'NONE', #7580, 1000.000000000000000 ) ;
#4447=CARTESIAN_POINT ( 'NONE',  ( -80.90000000000000568, -34.20000000000000284, 97.40192378864668399 ) ) ;
#4453=CARTESIAN_POINT ( 'NONE',  ( -79.39999999999999147, -32.41874999877096997, 99.99999999999998579 ) ) ;
#4455=CARTESIAN_POINT ( 'NONE',  ( 81.02178482187500208, -31.90312499938548996, 97.61286128772489690 ) ) ;
#4456=CARTESIAN_POINT ( 'NONE',  ( -82.39999999999999147, -34.83749999999999858, -97.00000000000000000 ) ) ;
#4457=CARTESIAN_POINT ( 'NONE',  ( -94.79999999999999716, -29.80000000000000426, 150.0000000000000000 ) ) ;
#4458=CARTESIAN_POINT ( 'NONE',  ( -84.28136653320150629, -32.00000000000001421, -102.0145392219080378 ) ) ;
#4459=CARTESIAN_POINT ( 'NONE',  ( -81.02178482187500208, -32.20312499938548711, -102.3871387122750889 ) ) ;
#4462=CARTESIAN_POINT ( 'NONE',  ( 85.15643035625001289, -31.15312499938548996, 99.99999999999998579 ) ) ;
#4464=CARTESIAN_POINT ( 'NONE',  ( 82.40000000000001990, -32.53124999877097423, 97.00000000000000000 ) ) ;
#4466=CARTESIAN_POINT ( 'NONE',  ( -79.64356964375001269, -30.89062499938548711, 98.40857419181659793 ) ) ;
#4468=VERTEX_POINT ( 'NONE', #12584 ) ;
#4469=EDGE_CURVE ( 'NONE', #14259, #13128, #799, .T. ) ;
#4470=CARTESIAN_POINT ( 'NONE',  ( -81.02178482187500208, -34.04062499938548569, -97.61286128772489690 ) ) ;
#4473=CARTESIAN_POINT ( 'NONE',  ( -79.64356964374999848, -33.17812499938548854, -99.99999999999998579 ) ) ;
#4474=CARTESIAN_POINT ( 'NONE',  ( -79.58826230849692251, -32.00000000000093792, -101.0460072438472139 ) ) ;
#4475=CARTESIAN_POINT ( 'NONE',  ( -79.39999999999999147, -31.93124999877096926, -101.7320508075688821 ) ) ;
#4480=CARTESIAN_POINT ( 'NONE',  ( 83.77821517812500929, -33.21562499938548285, 97.61286128772489690 ) ) ;
#4483=CARTESIAN_POINT ( 'NONE',  ( 79.39999999999999147, -34.18124999877097281, -98.26794919243110371 ) ) ;
#4491=VERTEX_POINT ( 'NONE', #18456 ) ;
#4497=CARTESIAN_POINT ( 'NONE',  ( 80.90000000000000568, -32.34374999877096712, -97.40192378864668399 ) ) ;
#4498=LINE ( 'NONE', #18176, #5818 ) ;
#4500=CARTESIAN_POINT ( 'NONE',  ( -82.39999999999999147, -35.09062499938548285, 103.1828516163667899 ) ) ;
#4504=EDGE_CURVE ( 'NONE', #12559, #15718, #8882, .T. ) ;
#4505=DIRECTION ( 'NONE',  ( 0.000000000000000000, -1.000000000000000000, 0.000000000000000000 ) ) ;
#4506=CARTESIAN_POINT ( 'NONE',  ( 82.39999999999999147, -33.65624999877097423, 103.0000000000000000 ) ) ;
#4507=CARTESIAN_POINT ( 'NONE',  ( -82.40000000000000568, -34.55624999877097281, -102.9999999999999858 ) ) ;
#4509=CARTESIAN_POINT ( 'NONE',  ( -83.77821517812500929, -33.21562499938548285, -97.61286128772489690 ) ) ;
#4512=CARTESIAN_POINT ( 'NONE',  ( 80.52691934816498076, -34.99999999999999289, -102.0537355158132868 ) ) ;
#4516=VERTEX_POINT ( 'NONE', #16894 ) ;
#4518=CARTESIAN_POINT ( 'NONE',  ( -80.90000000000000568, -34.80000000000000426, -97.40192378864668399 ) ) ;
#4520=CARTESIAN_POINT ( 'NONE',  ( -83.90000000000000568, -32.71874999877096712, 97.40192378864668399 ) ) ;
#4521=CARTESIAN_POINT ( 'NONE',  ( 80.90000000000000568, -31.05000000000000071, 102.5980762113533018 ) ) ;
#4527=CARTESIAN_POINT ( 'NONE',  ( 79.64356964375001269, -34.82812499938548711, 101.5914258081833879 ) ) ;
#4529=CARTESIAN_POINT ( 'NONE',  ( 83.77821517812500929, -32.31562499938548427, -102.3871387122750889 ) ) ;
#4532=CARTESIAN_POINT ( 'NONE',  ( -81.02178482187500208, -34.79062499938548569, 97.61286128772489690 ) ) ;
#4533=CARTESIAN_POINT ( 'NONE',  ( 85.15643035624999868, -33.32812499938548001, -98.40857419181659793 ) ) ;
#4534=DIRECTION ( 'NONE',  ( 0.000000000000000000, -1.000000000000000000, 0.000000000000000000 ) ) ;
#4537=CARTESIAN_POINT ( 'NONE',  ( -82.39999999999999147, -34.52812499938548996, 103.1828516163667899 ) ) ;
#4545=( BOUNDED_CURVE ( )  B_SPLINE_CURVE ( 2, ( #15953, #2556, #8519, #1101, #17710, #10659, #16535 ),
 .UNSPECIFIED., .F., .F. ) 
 B_SPLINE_CURVE_WITH_KNOTS ( ( 3, 2, 2, 3 ),
 ( 0.8958333333333333703, 0.9027777777777777901, 0.9166666666666666297, 0.9258785066912882389 ),
 .UNSPECIFIED. ) 
 CURVE ( )  GEOMETRIC_REPRESENTATION_ITEM ( )  RATIONAL_B_SPLINE_CURVE ( ( 0.9330127018922192983, 0.9330127018922198534, 1.000000000000000000, 0.8660254037844387076, 1.000000000000000000, 0.9111410165655264848, 0.9401539157124900736 ) ) 
 REPRESENTATION_ITEM ( '' )  );
#4547=CARTESIAN_POINT ( 'NONE',  ( -82.39999999999999147, -32.58749999999999858, -96.99999999999998579 ) ) ;
#4548=CARTESIAN_POINT ( 'NONE',  ( -83.90000000000000568, -32.17500000000000426, 102.5980762113533018 ) ) ;
#4550=CARTESIAN_POINT ( 'NONE',  ( 82.39999999999999147, -31.94062499938548427, 96.81714838363319586 ) ) ;
#4551=CARTESIAN_POINT ( 'NONE',  ( 81.02178482187500208, -30.40312499938548640, -97.61286128772489690 ) ) ;
#4552=DIRECTION ( 'NONE',  ( 0.000000000000000000, 1.000000000000000000, 0.000000000000000000 ) ) ;
#4553=LINE ( 'NONE', #10608, #4446 ) ;
#4554=CARTESIAN_POINT ( 'NONE',  ( -81.02178482187500208, -31.75312499938548427, -102.3871387122750889 ) ) ;
#4555=AXIS2_PLACEMENT_3D ( 'NONE', #1974, #15457, #12428 ) ;
#4557=CARTESIAN_POINT ( 'NONE',  ( 79.64356964375001269, -30.89062499938548711, 101.5914258081833879 ) ) ;
#4561=CARTESIAN_POINT ( 'NONE',  ( -85.15643035624999868, -32.46562499938548996, 101.5914258081833879 ) ) ;
#4564=CARTESIAN_POINT ( 'NONE',  ( -85.40000000000000568, -31.76249999999999929, -98.26794919243111792 ) ) ;
#4566=CARTESIAN_POINT ( 'NONE',  ( 80.90000000000000568, -33.69374999877096855, 102.5980762113533018 ) ) ;
#4567=CARTESIAN_POINT ( 'NONE',  ( -81.02178482187500208, -33.55312499938548854, -102.3871387122750889 ) ) ;
#4569=LINE ( 'NONE', #9056, #17996 ) ;
#4573=CARTESIAN_POINT ( 'NONE',  ( -85.15643035625001289, -34.64062499938548711, -99.99999999999998579 ) ) ;
#4574=CARTESIAN_POINT ( 'NONE',  ( 79.64356964374999848, -33.96562499938548285, 99.99999999999998579 ) ) ;
#4580=CARTESIAN_POINT ( 'NONE',  ( 79.39999999999999147, -34.25624999877096855, -101.7320508075688537 ) ) ;
#4594=CARTESIAN_POINT ( 'NONE',  ( -85.40000000000000568, -33.63750000000000284, -101.7320508075688821 ) ) ;
#4595=VERTEX_POINT ( 'NONE', #9851 ) ;
#4597=VECTOR ( 'NONE', #2853, 1000.000000000000000 ) ;
#4599=CARTESIAN_POINT ( 'NONE',  ( -82.39999999999999147, -34.64062499938548711, 103.1828516163667899 ) ) ;
#4604=ADVANCED_FACE ( 'NONE', ( #5656 ), #777, .F. ) ;
#4605=CARTESIAN_POINT ( 'NONE',  ( 80.90000000000000568, -34.80000000000000426, -102.5980762113533018 ) ) ;
#4610=ORIENTED_EDGE ( 'NONE', *, *, #413, .T. ) ;
#4612=CARTESIAN_POINT ( 'NONE',  ( -79.64356964375001269, -32.20312499938548001, -98.40857419181659793 ) ) ;
#4617=CARTESIAN_POINT ( 'NONE',  ( 83.90000000000000568, -33.07500000000000284, -102.5980762113533018 ) ) ;
#4619=AXIS2_PLACEMENT_3D ( 'NONE', #14912, #1541, #14709 ) ;
#4624=EDGE_CURVE ( 'NONE', #5649, #1717, #3986, .T. ) ;
#4626=CARTESIAN_POINT ( 'NONE',  ( -79.39999999999999147, -31.10624999877097352, 101.7320508075688537 ) ) ;
#4627=CARTESIAN_POINT ( 'NONE',  ( 85.40000000000000568, -32.28750000000000142, 101.7320508075688679 ) ) ;
#4628=VECTOR ( 'NONE', #2206, 1000.000000000000000 ) ;
#4629=DIRECTION ( 'NONE',  ( -0.000000000000000000, -0.000000000000000000, -1.000000000000000000 ) ) ;
#4634=VECTOR ( 'NONE', #4629, 1000.000000000000000 ) ;
#4636=CARTESIAN_POINT ( 'NONE',  ( 79.64356964375001269, -30.85312499938548569, -101.5914258081833879 ) ) ;
#4640=CARTESIAN_POINT ( 'NONE',  ( -85.15643035625001289, -34.60312499938548569, 101.5914258081833879 ) ) ;
#4641=CARTESIAN_POINT ( 'NONE',  ( 81.02178482187500208, -33.59062499938548285, -102.3871387122750889 ) ) ;
#4642=DIRECTION ( 'NONE',  ( -0.000000000000000000, -1.000000000000000000, -0.000000000000000000 ) ) ;
#4645=CARTESIAN_POINT ( 'NONE',  ( -79.64356964375001269, -34.90312499938548285, 101.5914258081833879 ) ) ;
#4647=CARTESIAN_POINT ( 'NONE',  ( 82.39999999999999147, -32.36250000000000426, 102.9999999999999858 ) ) ;
#4648=VECTOR ( 'NONE', #17272, 1000.000000000000000 ) ;
#4650=CARTESIAN_POINT ( 'NONE',  ( 82.39999999999999147, -30.92812499938548143, 96.81714838363319586 ) ) ;
#4655=CARTESIAN_POINT ( 'NONE',  ( 79.64356964375001269, -34.11562499938548854, 98.40857419181659793 ) ) ;
#4656=CARTESIAN_POINT ( 'NONE',  ( 79.64356964374999848, -30.47812499938548569, -99.99999999999998579 ) ) ;
#4659=CARTESIAN_POINT ( 'NONE',  ( -82.39999999999999147, -31.94062499938548427, -96.81714838363319586 ) ) ;
#4660=ORIENTED_EDGE ( 'NONE', *, *, #6043, .F. ) ;
#4661=CARTESIAN_POINT ( 'NONE',  ( 82.39999999999999147, -30.81562499938548427, 103.1828516163667899 ) ) ;
#4662=CARTESIAN_POINT ( 'NONE',  ( -83.20395887649198130, -35.00000000000002132, 102.6365808225363025 ) ) ;
#4664=CARTESIAN_POINT ( 'NONE',  ( -83.77821517812500929, -32.57812499938548711, 97.61286128772489690 ) ) ;
#4666=CARTESIAN_POINT ( 'NONE',  ( 85.40000000000000568, -33.05624999877097281, 98.26794919243111792 ) ) ;
#4668=CARTESIAN_POINT ( 'NONE',  ( -85.40000000000000568, -32.25000000000000000, -99.99999999999998579 ) ) ;
#4669=CARTESIAN_POINT ( 'NONE',  ( 83.90000000000000568, -34.42500000000000426, -102.5980762113533018 ) ) ;
#4670=CARTESIAN_POINT ( 'NONE',  ( 83.32052461991715120, -34.98323688327303671, -97.06736352196708140 ) ) ;
#4671=CARTESIAN_POINT ( 'NONE',  ( -82.39999999999999147, -32.84062499938548996, -96.81714838363319586 ) ) ;
#4676=CARTESIAN_POINT ( 'NONE',  ( -82.40000000000000568, -30.00000000000000355, -99.99999999999998579 ) ) ;
#4677=CARTESIAN_POINT ( 'NONE',  ( 85.15643035625001289, -33.29062499938547859, 99.99999999999998579 ) ) ;
#4679=CYLINDRICAL_SURFACE ( 'NONE', #15186, 3.000000000000002665 ) ;
#4680=CARTESIAN_POINT ( 'NONE',  ( 83.90000000000000568, -33.01874999877097139, -102.5980762113533018 ) ) ;
#4682=ORIENTED_EDGE ( 'NONE', *, *, #19070, .T. ) ;
#4687=ORIENTED_EDGE ( 'NONE', *, *, #17240, .F. ) ;
#4688=EDGE_LOOP ( 'NONE', ( #76, #7655, #11795, #13407 ) ) ;
#4692=EDGE_LOOP ( 'NONE', ( #10858, #18154, #4366, #2104 ) ) ;
#4696=CARTESIAN_POINT ( 'NONE',  ( -83.77821517812500929, -33.92812499938548854, 97.61286128772489690 ) ) ;
#4701=EDGE_CURVE ( 'NONE', #12847, #10833, #171, .T. ) ;
#4702=EDGE_CURVE ( 'NONE', #15327, #2447, #2369, .T. ) ;
#4705=CARTESIAN_POINT ( 'NONE',  ( -82.40000000000001990, -33.26250000000000284, 97.00000000000000000 ) ) ;
#4711=CARTESIAN_POINT ( 'NONE',  ( -82.39999999999999147, -32.27812499938548285, -96.81714838363319586 ) ) ;
#4714=CARTESIAN_POINT ( 'NONE',  ( -82.40000000000001990, -32.53124999877097423, 103.0000000000000000 ) ) ;
#4719=EDGE_LOOP ( 'NONE', ( #11046, #6665, #6259, #3347 ) ) ;
#4720=CARTESIAN_POINT ( 'NONE',  ( 82.40000000000000568, -34.78124999877096712, 96.99999999999998579 ) ) ;
#4724=CARTESIAN_POINT ( 'NONE',  ( -82.39999999999999147, -32.30624999877097281, 96.53589838486223584 ) ) ;
#4725=CARTESIAN_POINT ( 'NONE',  ( 82.39999999999999147, -32.13749999999999574, 96.53589838486223584 ) ) ;
#4726=CARTESIAN_POINT ( 'NONE',  ( 85.40000000000000568, -33.58124999877097139, 101.7320508075688821 ) ) ;
#4728=CARTESIAN_POINT ( 'NONE',  ( 81.02178482187500208, -33.25312499938548427, -102.3871387122750889 ) ) ;
#4729=DIRECTION ( 'NONE',  ( 0.000000000000000000, 0.000000000000000000, 1.000000000000000000 ) ) ;
#4730=CARTESIAN_POINT ( 'NONE',  ( 83.77821517812500929, -32.91562499938547859, -97.61286128772489690 ) ) ;
#4733=CARTESIAN_POINT ( 'NONE',  ( -83.20384757729338787, -33.95759618943233704, 102.9999999999999858 ) ) ;
#4734=CARTESIAN_POINT ( 'NONE',  ( 81.02178482187500208, -32.24062499938548854, -102.3871387122750889 ) ) ;
#4735=( BOUNDED_CURVE ( )  B_SPLINE_CURVE ( 2, ( #164, #5827, #4261, #13339, #4453, #17648, #16371, #7479, #9036 ),
 .UNSPECIFIED., .F., .F. ) 
 B_SPLINE_CURVE_WITH_KNOTS ( ( 3, 2, 2, 2, 3 ),
 ( 0.3541666666666666297, 0.3611111111111111049, 0.3750000000000000000, 0.3888888888888888951, 0.3958333333333334259 ),
 .UNSPECIFIED. ) 
 CURVE ( )  GEOMETRIC_REPRESENTATION_ITEM ( )  RATIONAL_B_SPLINE_CURVE ( ( 0.9330127018922194093, 0.9330127018922190762, 1.000000000000000000, 0.8660254037844387076, 1.000000000000000000, 0.8660254037844387076, 1.000000000000000000, 0.9330127018922185211, 0.9330127018922192983 ) ) 
 REPRESENTATION_ITEM ( '' )  );
#4736=CARTESIAN_POINT ( 'NONE',  ( 82.40000000000000568, -30.00000000000000355, 99.99999999999998579 ) ) ;
#4740=CARTESIAN_POINT ( 'NONE',  ( -81.02178482187500208, -34.79062499938548569, 97.61286128772489690 ) ) ;
#4749=AXIS2_PLACEMENT_3D ( 'NONE', #10853, #10573, #9007 ) ;
#4750=CARTESIAN_POINT ( 'NONE',  ( -82.39999999999999147, -34.33124999877097139, 103.0000000000000000 ) ) ;
#4752=CARTESIAN_POINT ( 'NONE',  ( 85.14613134194615895, -31.99999999999999289, 100.2978599400813806 ) ) ;
#4753=CARTESIAN_POINT ( 'NONE',  ( 79.64356964375001269, -34.49062499938548854, 101.5914258081833879 ) ) ;
#4754=CARTESIAN_POINT ( 'NONE',  ( 81.02178482187500208, -31.75312499938548427, -97.61286128772489690 ) ) ;
#4755=EDGE_CURVE ( 'NONE', #1228, #18284, #14243, .T. ) ;
#4757=CARTESIAN_POINT ( 'NONE',  ( -85.15643035625001289, -32.54062499938548569, 98.40857419181659793 ) ) ;
#4758=CARTESIAN_POINT ( 'NONE',  ( -81.02178482187500208, -33.25312499938548427, -97.61286128772489690 ) ) ;
#4761=CARTESIAN_POINT ( 'NONE',  ( 85.40000000000000568, -34.44374999877096855, 99.99999999999998579 ) ) ;
#4762=CARTESIAN_POINT ( 'NONE',  ( 82.40000000000000568, -30.00000000000000355, -99.99999999999998579 ) ) ;
#4764=CYLINDRICAL_SURFACE ( 'NONE', #2093, 3.000000000000002665 ) ;
#4766=CARTESIAN_POINT ( 'NONE',  ( -82.39999999999999147, -31.04062499938548569, 103.1828516163667899 ) ) ;
#4767=CARTESIAN_POINT ( 'NONE',  ( -82.40000000000000568, -30.00000000000000355, -99.99999999999998579 ) ) ;
#4768=ORIENTED_EDGE ( 'NONE', *, *, #13422, .T. ) ;
#4769=CARTESIAN_POINT ( 'NONE',  ( -85.40000000000000568, -31.31250000000000000, -98.26794919243111792 ) ) ;
#4771=CARTESIAN_POINT ( 'NONE',  ( -82.65333140691201663, -34.99995246259153703, -102.9892844631211943 ) ) ;
#4772=CARTESIAN_POINT ( 'NONE',  ( -79.64356964375001269, -34.11562499938548854, -98.40857419181659793 ) ) ;
#4778=CARTESIAN_POINT ( 'NONE',  ( 85.40000000000000568, -32.21250000000000568, 98.26794919243111792 ) ) ;
#4779=CARTESIAN_POINT ( 'NONE',  ( 79.64356964374999848, -33.06562499938548427, 99.99999999999998579 ) ) ;
#4781=VECTOR ( 'NONE', #8300, 1000.000000000000000 ) ;
#4783=CARTESIAN_POINT ( 'NONE',  ( 85.40000000000000568, -33.05624999877096570, -101.7320508075688679 ) ) ;
#4784=CARTESIAN_POINT ( 'NONE',  ( 79.39999999999999147, -34.68750000000000000, 101.7320508075688963 ) ) ;
#4791=ORIENTED_EDGE ( 'NONE', *, *, #17646, .F. ) ;
#4793=CARTESIAN_POINT ( 'NONE',  ( -82.39999999999999147, -30.25312499938548783, -103.1828516163667899 ) ) ;
#4798=VERTEX_POINT ( 'NONE', #4179 ) ;
#4800=EDGE_CURVE ( 'NONE', #2988, #15647, #1545, .T. ) ;
#4807=CARTESIAN_POINT ( 'NONE',  ( -82.40000000000000568, -30.00000000000000355, -103.0000000000000000 ) ) ;
#4808=CARTESIAN_POINT ( 'NONE',  ( -80.90000000000000568, -34.74374999877097281, -97.40192378864668399 ) ) ;
#4810=EDGE_LOOP ( 'NONE', ( #13781, #2165, #18706, #8786 ) ) ;
#4811=CARTESIAN_POINT ( 'NONE',  ( -79.64356964375001269, -33.47812499938547859, -101.5914258081833879 ) ) ;
#4812=DIRECTION ( 'NONE',  ( 0.000000000000000000, -1.000000000000000000, 0.000000000000000000 ) ) ;
#4815=FACE_OUTER_BOUND ( 'NONE', #14715, .T. ) ;
#4817=CARTESIAN_POINT ( 'NONE',  ( 96.99999999999994316, -29.80000000000000426, 150.0000000000000000 ) ) ;
#4818=EDGE_CURVE ( 'NONE', #6898, #14645, #16354, .T. ) ;
#4819=ORIENTED_EDGE ( 'NONE', *, *, #13543, .F. ) ;
#4820=ORIENTED_EDGE ( 'NONE', *, *, #19050, .F. ) ;
#4821=CARTESIAN_POINT ( 'NONE',  ( 81.59615242270662350, -33.41115380933863577, -102.9999999999999858 ) ) ;
#4822=CARTESIAN_POINT ( 'NONE',  ( 83.77821517812500929, -35.01562499938548711, -102.3871387122750889 ) ) ;
#4823=CARTESIAN_POINT ( 'NONE',  ( -79.39999999999999147, -32.00624999877096855, 101.7320508075688537 ) ) ;
#4824=CARTESIAN_POINT ( 'NONE',  ( 82.39999999999999147, -32.81250000000000000, 103.4641016151377499 ) ) ;
#4827=CARTESIAN_POINT ( 'NONE',  ( 79.64356964374998427, -33.59062499938548285, -98.40857419181659793 ) ) ;
#4828=ADVANCED_FACE ( 'NONE', ( #5938 ), #17856, .F. ) ;
#4829=CARTESIAN_POINT ( 'NONE',  ( -80.08630547029561342, -32.02340763552836478, -97.87171054440962337 ) ) ;
#4831=CARTESIAN_POINT ( 'NONE',  ( 82.39999999999999147, -34.07812499938548711, -103.1828516163667899 ) ) ;
#4832=VERTEX_POINT ( 'NONE', #10708 ) ;
#4834=CARTESIAN_POINT ( 'NONE',  ( -79.39999999999999147, -34.31250000000000000, 101.7320508075688537 ) ) ;
#4835=DIRECTION ( 'NONE',  ( -0.000000000000000000, -0.000000000000000000, -1.000000000000000000 ) ) ;
#4838=CARTESIAN_POINT ( 'NONE',  ( -80.90000000000000568, -30.30000000000000426, 102.5980762113533018 ) ) ;
#4843=CARTESIAN_POINT ( 'NONE',  ( 85.15643035624999868, -31.00312499938548072, 98.40857419181659793 ) ) ;
#4846=CARTESIAN_POINT ( 'NONE',  ( 81.02178482187500208, -30.89062499938548711, 97.61286128772489690 ) ) ;
#4848=CARTESIAN_POINT ( 'NONE',  ( 79.64356964375001269, -31.79062499938548569, -98.40857419181659793 ) ) ;
#4850=CARTESIAN_POINT ( 'NONE',  ( -82.39999999999999147, -32.05312499938548854, 96.81714838363319586 ) ) ;
#4851=CARTESIAN_POINT ( 'NONE',  ( -85.15643035624999868, -33.89062499938548711, -101.5914258081833879 ) ) ;
#4853=CARTESIAN_POINT ( 'NONE',  ( 82.39999999999999147, -30.59062499938548640, 96.81714838363319586 ) ) ;
#4857=CARTESIAN_POINT ( 'NONE',  ( -82.39999999999999147, -35.09062499938548285, 103.1828516163667899 ) ) ;
#4860=CARTESIAN_POINT ( 'NONE',  ( -82.39999999999999147, -30.11250000000000426, -103.4641016151377499 ) ) ;
#4861=CARTESIAN_POINT ( 'NONE',  ( 83.90000000000000568, -34.12500000000000000, -97.40192378864668399 ) ) ;
#4863=EDGE_CURVE ( 'NONE', #17884, #4491, #4158, .T. ) ;
#4864=CYLINDRICAL_SURFACE ( 'NONE', #11420, 3.000000000000002665 ) ;
#4869=CARTESIAN_POINT ( 'NONE',  ( 82.40000000000000568, -30.00000000000000355, 96.99999999999998579 ) ) ;
#4870=CARTESIAN_POINT ( 'NONE',  ( 81.59615242270662350, -32.96115380933864003, -103.0000000000000000 ) ) ;
#4871=CARTESIAN_POINT ( 'NONE',  ( 81.02178482187500208, -34.34062499938548285, 102.3871387122750889 ) ) ;
#4873=VECTOR ( 'NONE', #1423, 1000.000000000000000 ) ;
#4874=CARTESIAN_POINT ( 'NONE',  ( -83.90000000000000568, -34.51874999877097139, 97.40192378864668399 ) ) ;
#4875=CARTESIAN_POINT ( 'NONE',  ( 85.40000000000000568, -34.85624999877096997, -101.7320508075688679 ) ) ;
#4876=CARTESIAN_POINT ( 'NONE',  ( 80.90000000000000568, -34.80000000000000426, 97.40192378864668399 ) ) ;
#4882=EDGE_CURVE ( 'NONE', #15349, #4832, #5050, .T. ) ;
#4884=ORIENTED_EDGE ( 'NONE', *, *, #13096, .F. ) ;
#4887=CARTESIAN_POINT ( 'NONE',  ( -82.39999999999999147, -32.36250000000000426, -102.9999999999999858 ) ) ;
#4891=CARTESIAN_POINT ( 'NONE',  ( -80.90000000000000568, -34.14374999877097139, -102.5980762113533018 ) ) ;
#4896=CYLINDRICAL_SURFACE ( 'NONE', #17698, 3.000000000000002665 ) ;
#4902=CARTESIAN_POINT ( 'NONE',  ( -79.39999999999999147, -32.83124999877097139, -101.7320508075688963 ) ) ;
#4903=( BOUNDED_CURVE ( )  B_SPLINE_CURVE ( 2, ( #2425, #7116, #974, #10142, #6929, #16102, #17859, #16296, #7591 ),
 .UNSPECIFIED., .F., .F. ) 
 B_SPLINE_CURVE_WITH_KNOTS ( ( 3, 2, 2, 2, 3 ),
 ( 0.3541666666666666297, 0.3611111111111111049, 0.3750000000000000000, 0.3888888888888888951, 0.3958333333333334259 ),
 .UNSPECIFIED. ) 
 CURVE ( )  GEOMETRIC_REPRESENTATION_ITEM ( )  RATIONAL_B_SPLINE_CURVE ( ( 0.9330127018922194093, 0.9330127018922190762, 1.000000000000000000, 0.8660254037844387076, 1.000000000000000000, 0.8660254037844387076, 1.000000000000000000, 0.9330127018922185211, 0.9330127018922192983 ) ) 
 REPRESENTATION_ITEM ( '' )  );
#4905=CARTESIAN_POINT ( 'NONE',  ( -80.90000000000000568, -33.30000000000000426, -102.5980762113533018 ) ) ;
#4907=AXIS2_PLACEMENT_3D ( 'NONE', #2469, #11260, #5418 ) ;
#4913=ORIENTED_EDGE ( 'NONE', *, *, #3153, .F. ) ;
#4914=CARTESIAN_POINT ( 'NONE',  ( -84.12306224665888976, -31.99999999999999289, 102.1915028381727382 ) ) ;
#4915=CARTESIAN_POINT ( 'NONE',  ( 81.02178482187500208, -34.94062499938548427, -102.3871387122750889 ) ) ;
#4916=DIRECTION ( 'NONE',  ( 0.000000000000000000, -1.000000000000000000, 0.000000000000000000 ) ) ;
#4917=CARTESIAN_POINT ( 'NONE',  ( -85.40000000000000568, -34.85624999877096997, 101.7320508075688679 ) ) ;
#4919=CARTESIAN_POINT ( 'NONE',  ( 82.39999999999999147, -33.43124999877097281, 96.99999999999998579 ) ) ;
#4920=CARTESIAN_POINT ( 'NONE',  ( 83.77821517812500929, -32.87812499938548427, -102.3871387122750889 ) ) ;
#4923=CARTESIAN_POINT ( 'NONE',  ( 79.39999999999999147, -33.41250000000000142, -101.7320508075688537 ) ) ;
#4924=CARTESIAN_POINT ( 'NONE',  ( -85.15643035624999868, -33.25312499938548427, 101.5914258081833879 ) ) ;
#4925=CARTESIAN_POINT ( 'NONE',  ( 85.15643035624999868, -32.80312499938548854, -101.5914258081833879 ) ) ;
#4930=CYLINDRICAL_SURFACE ( 'NONE', #18872, 2.199999999999993516 ) ;
#4934=CARTESIAN_POINT ( 'NONE',  ( -85.40000000000000568, -32.28750000000000142, 98.26794919243111792 ) ) ;
#4935=ORIENTED_EDGE ( 'NONE', *, *, #4469, .T. ) ;
#4938=FACE_OUTER_BOUND ( 'NONE', #11814, .T. ) ;
#4939=VECTOR ( 'NONE', #17898, 1000.000000000000000 ) ;
#4940=VECTOR ( 'NONE', #11546, 1000.000000000000000 ) ;
#4943=CARTESIAN_POINT ( 'NONE',  ( 84.29633955546293578, -32.00000000000002132, 97.97042480180311941 ) ) ;
#4944=CARTESIAN_POINT ( 'NONE',  ( 82.39999999999999147, -34.64062499938548711, 96.81714838363319586 ) ) ;
#4945=B_SPLINE_CURVE_WITH_KNOTS ( 'NONE', 3,
 ( #17458, #6821, #3772, #9834, #3872, #7096, #17265, #15987, #8270, #12954 ),
 .UNSPECIFIED., .F., .F.,
 ( 4, 2, 2, 2, 4 ),
 ( 0.3612006186103786654, 0.3925526867148934063, 0.4239047548194081472, 0.4552568229239228881, 0.4866088910284376290 ),
 .UNSPECIFIED. ) ;
#4947=CARTESIAN_POINT ( 'NONE',  ( 85.15643035624999868, -32.01562499938548711, -101.5914258081833879 ) ) ;
#4948=VECTOR ( 'NONE', #11090, 1000.000000000000000 ) ;
#4950=CARTESIAN_POINT ( 'NONE',  ( -79.64356964374998427, -34.56562499938548427, 101.5914258081833879 ) ) ;
#4951=CARTESIAN_POINT ( 'NONE',  ( -81.02178482187500208, -34.45312499938548711, -102.3871387122750889 ) ) ;
#4953=CARTESIAN_POINT ( 'NONE',  ( 83.77821517812500929, -32.42812499938548854, 97.61286128772489690 ) ) ;
#4956=CARTESIAN_POINT ( 'NONE',  ( -82.39999999999999147, -31.82812499938548356, 103.1828516163667899 ) ) ;
#4957=CARTESIAN_POINT ( 'NONE',  ( -79.64356964375001269, -34.11562499938548854, 101.5914258081833879 ) ) ;
#4958=CARTESIAN_POINT ( 'NONE',  ( -82.40000000000000568, -30.00000000000000355, 99.99999999999998579 ) ) ;
#4960=CARTESIAN_POINT ( 'NONE',  ( -80.90000000000000568, -32.55000000000000426, -97.40192378864668399 ) ) ;
#4964=CYLINDRICAL_SURFACE ( 'NONE', #7359, 3.000000000000002665 ) ;
#4965=ADVANCED_FACE ( 'NONE', ( #6229 ), #8071, .F. ) ;
#4970=EDGE_LOOP ( 'NONE', ( #17911, #2314, #14959, #431 ) ) ;
#4974=CARTESIAN_POINT ( 'NONE',  ( 85.40000000000000568, -34.44374999877096855, -99.99999999999998579 ) ) ;
#4976=CARTESIAN_POINT ( 'NONE',  ( 83.77821517812500929, -32.42812499938548854, -102.3871387122750889 ) ) ;
#4979=CARTESIAN_POINT ( 'NONE',  ( 80.90000000000000568, -30.69374999877097210, 97.40192378864668399 ) ) ;
#4989=CARTESIAN_POINT ( 'NONE',  ( -83.20384757729338787, -33.95759618943233704, -97.00000000000000000 ) ) ;
#4990=VERTEX_POINT ( 'NONE', #6325 ) ;
#4991=CARTESIAN_POINT ( 'NONE',  ( 81.02178482187500208, -32.20312499938548711, 102.3871387122750889 ) ) ;
#4992=CARTESIAN_POINT ( 'NONE',  ( -83.90000000000000568, -33.01874999877097139, -97.40192378864668399 ) ) ;
#4997=CARTESIAN_POINT ( 'NONE',  ( 84.75088379147460671, -34.99999999999999289, -101.6079878054130035 ) ) ;
#4999=CARTESIAN_POINT ( 'NONE',  ( -79.39999999999999147, -34.18124999877097281, 98.26794919243110371 ) ) ;
#5006=ORIENTED_EDGE ( 'NONE', *, *, #8397, .F. ) ;
#5008=DIRECTION ( 'NONE',  ( 0.000000000000000000, -1.000000000000000000, 0.000000000000000000 ) ) ;
#5010=ORIENTED_EDGE ( 'NONE', *, *, #3978, .F. ) ;
#5013=ORIENTED_EDGE ( 'NONE', *, *, #4818, .T. ) ;
#5014=CARTESIAN_POINT ( 'NONE',  ( -80.42036527867318796, -31.99999999999998579, 102.1983759483903924 ) ) ;
#5015=CARTESIAN_POINT ( 'NONE',  ( 79.39999999999999147, -30.18750000000000355, -98.26794919243110371 ) ) ;
#5017=CARTESIAN_POINT ( 'NONE',  ( -80.90000000000000568, -34.29374999877096997, 102.5980762113533018 ) ) ;
#5018=DIRECTION ( 'NONE',  ( 1.000000000000000000, 0.000000000000000000, 0.000000000000000000 ) ) ;
#5020=CARTESIAN_POINT ( 'NONE',  ( 83.77821517812500929, -33.02812499938548285, -97.61286128772489690 ) ) ;
#5022=CARTESIAN_POINT ( 'NONE',  ( -83.77821517812500929, -32.31562499938548427, 102.3871387122750889 ) ) ;
#5023=CARTESIAN_POINT ( 'NONE',  ( 81.02178482187500208, -34.04062499938548569, -102.3871387122750889 ) ) ;
#5024=ORIENTED_EDGE ( 'NONE', *, *, #11145, .F. ) ;
#5026=CARTESIAN_POINT ( 'NONE',  ( -85.40000000000000568, -34.95000000000000284, 99.99999999999998579 ) ) ;
#5027=CARTESIAN_POINT ( 'NONE',  ( 82.39999999999999147, -33.48750000000000426, -103.0000000000000000 ) ) ;
#5031=CARTESIAN_POINT ( 'NONE',  ( -83.90000000000000568, -31.72500000000000142, 102.5980762113533018 ) ) ;
#5035=CARTESIAN_POINT ( 'NONE',  ( 79.64356964375001269, -33.10312499938549280, 98.40857419181659793 ) ) ;
#5036=CARTESIAN_POINT ( 'NONE',  ( 84.85729912020865129, -31.99999999999998579, -101.2614033343868414 ) ) ;
#5038=CARTESIAN_POINT ( 'NONE',  ( -83.77821517812500929, -32.57812499938548711, -102.3871387122750889 ) ) ;
#5039=CARTESIAN_POINT ( 'NONE',  ( 82.39999999999999147, -30.25312499938548783, 103.1828516163667899 ) ) ;
#5040=B_SPLINE_CURVE_WITH_KNOTS ( 'NONE', 3,
 ( #10265, #14743, #1378, #7324, #19252, #5870, #11821, #13760, #113, #10735, #3115, #10929, #9363, #3409, #10830, #16897, #15324, #16512 ),
 .UNSPECIFIED., .F., .F.,
 ( 4, 2, 2, 2, 2, 2, 2, 2, 4 ),
 ( 0.000000000000000000, 0.0007089252359835698227, 0.001417850471967139645, 0.002126775707950709360, 0.002835700943934279291, 0.003544626179917849222, 0.004253551415901418720, 0.004962476651884989085, 0.005671401887868558582 ),
 .UNSPECIFIED. ) ;
#5041=CARTESIAN_POINT ( 'NONE',  ( 85.15643035624999868, -31.64062499938548356, -98.40857419181659793 ) ) ;
#5043=CARTESIAN_POINT ( 'NONE',  ( -79.64356964374998427, -33.14062499938548711, 98.40857419181659793 ) ) ;
#5044=CARTESIAN_POINT ( 'NONE',  ( -85.15643035624999868, -32.99062499938548854, -101.5914258081833879 ) ) ;
#5045=VERTEX_POINT ( 'NONE', #11194 ) ;
#5046=CARTESIAN_POINT ( 'NONE',  ( 81.02178482187500208, -32.35312499938548569, 97.61286128772489690 ) ) ;
#5048=CARTESIAN_POINT ( 'NONE',  ( -83.77821517812500929, -30.66562499938548569, 97.61286128772489690 ) ) ;
#5049=CARTESIAN_POINT ( 'NONE',  ( -82.39999999999999147, -33.51562499938548001, 96.81714838363319586 ) ) ;
#5050=LINE ( 'NONE', #15200, #3682 ) ;
#5051=ORIENTED_EDGE ( 'NONE', *, *, #5069, .T. ) ;
#5052=CARTESIAN_POINT ( 'NONE',  ( -85.40000000000000568, -33.63750000000000284, -101.7320508075688679 ) ) ;
#5055=CARTESIAN_POINT ( 'NONE',  ( 82.40000000000000568, -30.00000000000000355, -99.99999999999998579 ) ) ;
#5056=CARTESIAN_POINT ( 'NONE',  ( 84.57144699476174310, -35.00000000000000000, -97.92073041325133431 ) ) ;
#5057=LINE ( 'NONE', #5149, #2987 ) ;
#5060=ORIENTED_EDGE ( 'NONE', *, *, #7076, .F. ) ;
#5064=CARTESIAN_POINT ( 'NONE',  ( 82.39999999999999147, -34.33124999877097139, -103.0000000000000000 ) ) ;
#5065=CARTESIAN_POINT ( 'NONE',  ( 82.39999999999999147, -30.36562499938549209, -96.81714838363319586 ) ) ;
#5069=EDGE_CURVE ( 'NONE', #16231, #16006, #17452, .T. ) ;
#5071=CARTESIAN_POINT ( 'NONE',  ( 82.39999999999999147, -30.73124999877096641, 96.53589838486223584 ) ) ;
#5078=VERTEX_POINT ( 'NONE', #5348 ) ;
#5080=CARTESIAN_POINT ( 'NONE',  ( -82.39999999999999147, -32.27812499938548285, -96.81714838363319586 ) ) ;
#5081=CARTESIAN_POINT ( 'NONE',  ( -85.40000000000000568, -32.28750000000000142, -101.7320508075688821 ) ) ;
#5084=CARTESIAN_POINT ( 'NONE',  ( -85.40000000000000568, -34.03124999877096712, -101.7320508075688679 ) ) ;
#5089=CARTESIAN_POINT ( 'NONE',  ( 96.99999999999997158, -5.200000000000003730, -150.0000000000000000 ) ) ;
#5091=CARTESIAN_POINT ( 'NONE',  ( 85.40000000000000568, -30.43124999877096926, -98.26794919243111792 ) ) ;
#5094=CARTESIAN_POINT ( 'NONE',  ( 82.39999999999999147, -32.05312499938548854, -96.81714838363319586 ) ) ;
#5103=CARTESIAN_POINT ( 'NONE',  ( 99.99999999999994316, -29.80000000000000782, -150.0000000000000000 ) ) ;
#5107=VERTEX_POINT ( 'NONE', #1131 ) ;
#5108=CARTESIAN_POINT ( 'NONE',  ( -79.79666399293490997, -31.99999999999999289, 101.4892189721554416 ) ) ;
#5109=CARTESIAN_POINT ( 'NONE',  ( 82.39999999999999147, -34.75312499938549138, -96.81714838363319586 ) ) ;
#5111=CARTESIAN_POINT ( 'NONE',  ( -83.77821517812500929, -30.32812499938548711, 97.61286128772489690 ) ) ;
#5115=CARTESIAN_POINT ( 'NONE',  ( 79.39999999999999147, -33.28124999877096712, 101.7320508075688963 ) ) ;
#5116=CARTESIAN_POINT ( 'NONE',  ( 85.15643035625001289, -32.05312499938548854, -99.99999999999998579 ) ) ;
#5117=LINE ( 'NONE', #11057, #4323 ) ;
#5118=CARTESIAN_POINT ( 'NONE',  ( -83.77821517812500929, -34.11562499938548854, 102.3871387122750889 ) ) ;
#5119=CARTESIAN_POINT ( 'NONE',  ( 85.15643035624999868, -34.60312499938548569, -101.5914258081833879 ) ) ;
#5126=CARTESIAN_POINT ( 'NONE',  ( -85.40000000000000568, -32.25000000000000000, 99.99999999999998579 ) ) ;
#5130=CARTESIAN_POINT ( 'NONE',  ( 81.02178482187500208, -33.44062499938548427, 102.3871387122750889 ) ) ;
#5131=CARTESIAN_POINT ( 'NONE',  ( 79.39999999999999147, -32.06250000000000000, -101.7320508075688537 ) ) ;
#5133=CARTESIAN_POINT ( 'NONE',  ( 80.80636817121803972, -32.00000000000000000, 97.53037344451318802 ) ) ;
#5134=CARTESIAN_POINT ( 'NONE',  ( 83.77821517812500929, -31.11562499938548498, 102.3871387122750889 ) ) ;
#5135=CARTESIAN_POINT ( 'NONE',  ( 85.15643035624999868, -30.74062499938548143, -98.40857419181659793 ) ) ;
#5137=CARTESIAN_POINT ( 'NONE',  ( -79.64356964374999848, -33.62812499938548427, 99.99999999999998579 ) ) ;
#5138=CARTESIAN_POINT ( 'NONE',  ( -81.02178482187500208, -34.00312499938548427, -102.3871387122750889 ) ) ;
#5140=CARTESIAN_POINT ( 'NONE',  ( 81.02178482187500208, -31.90312499938548996, 97.61286128772489690 ) ) ;
#5142=CARTESIAN_POINT ( 'NONE',  ( -85.15643035624999868, -33.36562499938548854, 101.5914258081833879 ) ) ;
#5146=CARTESIAN_POINT ( 'NONE',  ( -83.90000000000000568, -34.42500000000000426, -97.40192378864668399 ) ) ;
#5148=DIRECTION ( 'NONE',  ( -0.000000000000000000, -1.000000000000000000, -0.000000000000000000 ) ) ;
#5149=CARTESIAN_POINT ( 'NONE',  ( 99.99999999999994316, -32.00000000000000000, 150.0000000000000000 ) ) ;
#5152=ORIENTED_EDGE ( 'NONE', *, *, #8633, .F. ) ;
#5155=CARTESIAN_POINT ( 'NONE',  ( -85.40000000000000568, -33.18750000000000000, 98.26794919243111792 ) ) ;
#5156=CARTESIAN_POINT ( 'NONE',  ( 83.77821517812500929, -30.77812499938548640, 102.3871387122750889 ) ) ;
#5157=CARTESIAN_POINT ( 'NONE',  ( -82.40000000000000568, -30.00000000000000355, 99.99999999999998579 ) ) ;
#5158=CARTESIAN_POINT ( 'NONE',  ( 85.15643035624999868, -31.56562499938548427, -101.5914258081833879 ) ) ;
#5162=CARTESIAN_POINT ( 'NONE',  ( 85.40000000000000568, -31.78124999877096712, 101.7320508075688679 ) ) ;
#5168=VERTEX_POINT ( 'NONE', #14498 ) ;
#5170=CARTESIAN_POINT ( 'NONE',  ( -82.39999999999999147, -30.92812499938548143, -96.81714838363319586 ) ) ;
#5171=DIRECTION ( 'NONE',  ( 1.000000000000000000, 0.000000000000000000, 0.000000000000000000 ) ) ;
#5172=VERTEX_POINT ( 'NONE', #6812 ) ;
#5173=CARTESIAN_POINT ( 'NONE',  ( 85.15643035625001289, -32.95312499938548711, 99.99999999999998579 ) ) ;
#5174=CARTESIAN_POINT ( 'NONE',  ( -80.90000000000000568, -33.84374999877096712, -97.40192378864668399 ) ) ;
#5176=FACE_OUTER_BOUND ( 'NONE', #139, .T. ) ;
#5177=LINE ( 'NONE', #11123, #2881 ) ;
#5183=CARTESIAN_POINT ( 'NONE',  ( 82.39999999999999147, -30.50624999877097210, -96.53589838486223584 ) ) ;
#5185=EDGE_CURVE ( 'NONE', #13728, #18169, #14403, .T. ) ;
#5187=CARTESIAN_POINT ( 'NONE',  ( 83.77821517812500929, -33.66562499938548569, -102.3871387122750889 ) ) ;
#5189=CARTESIAN_POINT ( 'NONE',  ( -82.39999999999999147, -32.98124999877096286, -96.99999999999998579 ) ) ;
#5193=CARTESIAN_POINT ( 'NONE',  ( 79.58826230851033756, -31.99999999999998579, -98.95399275611669054 ) ) ;
#5200=ADVANCED_FACE ( 'NONE', ( #5539 ), #18825, .F. ) ;
#5201=CARTESIAN_POINT ( 'NONE',  ( 85.40000000000000568, -30.86250000000000071, -101.7320508075688679 ) ) ;
#5204=EDGE_CURVE ( 'NONE', #4595, #10520, #12770, .T. ) ;
#5205=CARTESIAN_POINT ( 'NONE',  ( -85.40000000000000568, -33.50624999877096855, 101.7320508075688679 ) ) ;
#5207=CARTESIAN_POINT ( 'NONE',  ( -83.90000000000000568, -32.26874999877097139, -102.5980762113533018 ) ) ;
#5210=CARTESIAN_POINT ( 'NONE',  ( 79.64356964374998427, -34.56562499938548427, -101.5914258081833879 ) ) ;
#5211=CARTESIAN_POINT ( 'NONE',  ( -80.90000000000000568, -33.69374999877096855, 97.40192378864668399 ) ) ;
#5212=CARTESIAN_POINT ( 'NONE',  ( -85.15643035625001289, -33.29062499938547859, 99.99999999999998579 ) ) ;
#5216=CARTESIAN_POINT ( 'NONE',  ( -84.69814068649969840, -35.00052333152936512, 98.07164593887567605 ) ) ;
#5222=VECTOR ( 'NONE', #3126, 1000.000000000000000 ) ;
#5227=CARTESIAN_POINT ( 'NONE',  ( 85.15643035624999868, -31.90312499938548285, 98.40857419181659793 ) ) ;
#5229=CARTESIAN_POINT ( 'NONE',  ( 82.40000000000001990, -32.13750000000000284, -103.0000000000000000 ) ) ;
#5234=CARTESIAN_POINT ( 'NONE',  ( 79.64356964374999848, -31.71562499938548285, 99.99999999999998579 ) ) ;
#5235=CARTESIAN_POINT ( 'NONE',  ( 85.15643035624999868, -34.26562499938548711, -101.5914258081833879 ) ) ;
#5237=CARTESIAN_POINT ( 'NONE',  ( -79.64356964374999848, -34.52812499938548285, 99.99999999999998579 ) ) ;
#5238=CARTESIAN_POINT ( 'NONE',  ( -82.39999999999999147, -31.15312499938548640, -103.1828516163667899 ) ) ;
#5240=CARTESIAN_POINT ( 'NONE',  ( 81.02178482187500208, -32.20312499938548711, 102.3871387122750889 ) ) ;
#5243=CARTESIAN_POINT ( 'NONE',  ( -82.39999999999999147, -30.70312499938548711, 96.81714838363319586 ) ) ;
#5244=CARTESIAN_POINT ( 'NONE',  ( -85.15643035624999868, -32.91562499938549280, 101.5914258081833879 ) ) ;
#5245=ORIENTED_EDGE ( 'NONE', *, *, #13574, .F. ) ;
#5246=CARTESIAN_POINT ( 'NONE',  ( -85.40000000000000568, -33.60000000000000142, -99.99999999999998579 ) ) ;
#5247=VECTOR ( 'NONE', #1252, 1000.000000000000000 ) ;
#5248=( BOUNDED_CURVE ( )  B_SPLINE_CURVE ( 2, ( #9278, #11757, #13679, #13121, #12123, #19092, #16524, #18093, #13772 ),
 .UNSPECIFIED., .F., .T. ) 
 B_SPLINE_CURVE_WITH_KNOTS ( ( 3, 2, 2, 2, 3 ),
 ( 0.6875000000000000000, 0.6944444444444444198, 0.7083333333333333703, 0.7222222222222222099, 0.7291666666666668517 ),
 .UNSPECIFIED. ) 
 CURVE ( )  GEOMETRIC_REPRESENTATION_ITEM ( )  RATIONAL_B_SPLINE_CURVE ( ( 0.9330127018922194093, 0.9330127018922194093, 1.000000000000000000, 0.8660254037844387076, 1.000000000000000000, 0.8660254037844387076, 1.000000000000000000, 0.9330127018922177440, 0.9330127018922194093 ) ) 
 REPRESENTATION_ITEM ( '' )  );
#5251=CARTESIAN_POINT ( 'NONE',  ( 80.90000000000000568, -33.00000000000000000, -102.5980762113533018 ) ) ;
#5252=DIRECTION ( 'NONE',  ( 1.000000000000000000, -1.577021341797101948E-15, 0.000000000000000000 ) ) ;
#5258=CARTESIAN_POINT ( 'NONE',  ( -83.32052461991715120, -34.98323688327303671, 97.06736352196708140 ) ) ;
#5261=CARTESIAN_POINT ( 'NONE',  ( 85.15643035624999868, -30.29062499938548925, 101.5914258081833879 ) ) ;
#5262=CARTESIAN_POINT ( 'NONE',  ( -85.40000000000000568, -34.44374999877096855, 99.99999999999998579 ) ) ;
#5263=LINE ( 'NONE', #12772, #16194 ) ;
#5264=CARTESIAN_POINT ( 'NONE',  ( 85.15643035624999868, -32.09062499938548996, -98.40857419181659793 ) ) ;
#5266=CARTESIAN_POINT ( 'NONE',  ( 82.40000000000001990, -32.75624999877096855, 103.0000000000000000 ) ) ;
#5268=CARTESIAN_POINT ( 'NONE',  ( 85.40000000000000568, -31.74374999877096926, 99.99999999999998579 ) ) ;
#5273=ORIENTED_EDGE ( 'NONE', *, *, #12360, .F. ) ;
#5274=CARTESIAN_POINT ( 'NONE',  ( -79.64356964375001269, -32.65312499938548285, -98.40857419181659793 ) ) ;
#5275=LINE ( 'NONE', #14623, #17545 ) ;
#5277=CARTESIAN_POINT ( 'NONE',  ( 85.15643035625001289, -34.34062499938548285, 101.5914258081833879 ) ) ;
#5278=CARTESIAN_POINT ( 'NONE',  ( -85.40000000000000568, -34.48124999877096997, -101.7320508075688679 ) ) ;
#5280=CARTESIAN_POINT ( 'NONE',  ( 85.40000000000000568, -34.50000000000000000, 99.99999999999998579 ) ) ;
#5281=CARTESIAN_POINT ( 'NONE',  ( -79.60045861139941792, -35.00000000000000000, 99.68825842090977574 ) ) ;
#5289=CARTESIAN_POINT ( 'NONE',  ( 84.28136653320188998, -32.00000000000000000, -97.98546077809228905 ) ) ;
#5293=ORIENTED_EDGE ( 'NONE', *, *, #16453, .F. ) ;
#5294=CARTESIAN_POINT ( 'NONE',  ( 82.39999999999999147, -32.58749999999999858, 96.99999999999998579 ) ) ;
#5298=CARTESIAN_POINT ( 'NONE',  ( -82.40000000000001990, -33.88124999877096855, -97.00000000000000000 ) ) ;
#5299=EDGE_CURVE ( 'NONE', #13270, #4516, #12883, .T. ) ;
#5301=ORIENTED_EDGE ( 'NONE', *, *, #430, .F. ) ;
#5302=( BOUNDED_CURVE ( )  B_SPLINE_CURVE ( 2, ( #5294, #11337, #15740, #17302, #2346, #5391, #3908, #9975, #2531 ),
 .UNSPECIFIED., .F., .F. ) 
 B_SPLINE_CURVE_WITH_KNOTS ( ( 3, 2, 2, 2, 3 ),
 ( 0.4791666666666666297, 0.4861111111111111049, 0.5000000000000000000, 0.5138888888888888395, 0.5208333333333333703 ),
 .UNSPECIFIED. ) 
 CURVE ( )  GEOMETRIC_REPRESENTATION_ITEM ( )  RATIONAL_B_SPLINE_CURVE ( ( 0.9330127018922194093, 0.9330127018922190762, 1.000000000000000000, 0.8660254037844387076, 1.000000000000000000, 0.8660254037844387076, 1.000000000000000000, 0.9330127018922187432, 0.9330127018922192983 ) ) 
 REPRESENTATION_ITEM ( '' )  );
#5304=CARTESIAN_POINT ( 'NONE',  ( 82.39999999999999147, -33.48750000000000426, -103.4641016151377499 ) ) ;
#5306=EDGE_CURVE ( 'NONE', #7789, #13728, #57, .T. ) ;
#5308=CARTESIAN_POINT ( 'NONE',  ( -79.64356964375001269, -31.41562499938548569, 101.5914258081833879 ) ) ;
#5312=CARTESIAN_POINT ( 'NONE',  ( -99.99999999999998579, 0.000000000000000000, -150.0000000000000000 ) ) ;
#5313=CARTESIAN_POINT ( 'NONE',  ( 79.77811200999867935, -34.99999999999999289, -100.8506536761476156 ) ) ;
#5315=CARTESIAN_POINT ( 'NONE',  ( -79.64356964375001269, -32.57812499938548001, 98.40857419181659793 ) ) ;
#5317=VERTEX_POINT ( 'NONE', #11960 ) ;
#5319=( NAMED_UNIT ( * ) PLANE_ANGLE_UNIT ( ) SI_UNIT ( $, .RADIAN. ) );
#5324=EDGE_CURVE ( 'NONE', #15108, #13408, #19306, .T. ) ;
#5330=CARTESIAN_POINT ( 'NONE',  ( 80.52691934816499497, -34.99999999999999289, 97.94626448418664211 ) ) ;
#5331=CARTESIAN_POINT ( 'NONE',  ( 81.02178482187500208, -31.34062499938548996, 97.61286128772489690 ) ) ;
#5334=ADVANCED_BREP_SHAPE_REPRESENTATION ( '', ( #3164, #10540 ), #11151 ) ;
#5337=CARTESIAN_POINT ( 'NONE',  ( -85.15643035625001289, -32.95312499938548711, -99.99999999999998579 ) ) ;
#5338=CARTESIAN_POINT ( 'NONE',  ( 81.02178482187500208, -33.14062499938548711, 97.61286128772489690 ) ) ;
#5339=CARTESIAN_POINT ( 'NONE',  ( 82.39999999999999147, -33.06562499938548427, -96.81714838363319586 ) ) ;
#5341=CARTESIAN_POINT ( 'NONE',  ( -79.64356964374998427, -32.12812499938548427, 98.40857419181659793 ) ) ;
#5342=EDGE_LOOP ( 'NONE', ( #10734, #16760, #5634, #16827 ) ) ;
#5343=CARTESIAN_POINT ( 'NONE',  ( 79.64356964375001269, -31.86562499938548143, 98.40857419181659793 ) ) ;
#5346=LINE ( 'NONE', #15787, #16762 ) ;
#5347=CARTESIAN_POINT ( 'NONE',  ( -81.02178482187500208, -31.19062499938548427, 97.61286128772489690 ) ) ;
#5348=CARTESIAN_POINT ( 'NONE',  ( 94.79999999999984084, 0.000000000000000000, -150.0000000000000000 ) ) ;
#5349=ORIENTED_EDGE ( 'NONE', *, *, #15583, .F. ) ;
#5350=CARTESIAN_POINT ( 'NONE',  ( -79.39999999999999147, -32.96250000000000568, -98.26794919243113213 ) ) ;
#5353=CARTESIAN_POINT ( 'NONE',  ( 83.20384757729337366, -33.50759618943233420, -103.0000000000000000 ) ) ;
#5356=CARTESIAN_POINT ( 'NONE',  ( -83.20384757729337366, -34.80134618820331127, 103.0000000000000000 ) ) ;
#5358=CARTESIAN_POINT ( 'NONE',  ( 83.77821517812500929, -34.71562499938548285, 102.3871387122750889 ) ) ;
#5359=PLANE ( 'NONE',  #13674 ) ;
#5361=CARTESIAN_POINT ( 'NONE',  ( 81.02178482187500208, -31.90312499938548996, -102.3871387122750889 ) ) ;
#5362=CARTESIAN_POINT ( 'NONE',  ( 79.39999999999999147, -32.83124999877097139, 101.7320508075688963 ) ) ;
#5364=CARTESIAN_POINT ( 'NONE',  ( 85.40000000000000568, -31.25624999877096855, 98.26794919243111792 ) ) ;
#5367=( BOUNDED_CURVE ( )  B_SPLINE_CURVE ( 2, ( #5722, #18030, #13326, #14989, #8735, #1518, #1324, #5915, #7468 ),
 .UNSPECIFIED., .F., .F. ) 
 B_SPLINE_CURVE_WITH_KNOTS ( ( 3, 2, 2, 2, 3 ),
 ( 0.6875000000000000000, 0.6944444444444444198, 0.7083333333333333703, 0.7222222222222222099, 0.7291666666666668517 ),
 .UNSPECIFIED. ) 
 CURVE ( )  GEOMETRIC_REPRESENTATION_ITEM ( )  RATIONAL_B_SPLINE_CURVE ( ( 0.9330127018922194093, 0.9330127018922194093, 1.000000000000000000, 0.8660254037844387076, 1.000000000000000000, 0.8660254037844387076, 1.000000000000000000, 0.9330127018922177440, 0.9330127018922194093 ) ) 
 REPRESENTATION_ITEM ( '' )  );
#5370=ORIENTED_EDGE ( 'NONE', *, *, #5299, .F. ) ;
#5371=CARTESIAN_POINT ( 'NONE',  ( -85.15643035624999868, -30.55312499938548854, -98.40857419181659793 ) ) ;
#5373=ORIENTED_EDGE ( 'NONE', *, *, #14122, .T. ) ;
#5374=CARTESIAN_POINT ( 'NONE',  ( 81.02178482187500208, -33.10312499938548569, 102.3871387122750889 ) ) ;
#5375=CARTESIAN_POINT ( 'NONE',  ( -79.64356964375001269, -31.79062499938548569, -101.5914258081833879 ) ) ;
#5376=CARTESIAN_POINT ( 'NONE',  ( 79.39999999999999147, -33.82500000000000284, 99.99999999999998579 ) ) ;
#5377=CARTESIAN_POINT ( 'NONE',  ( 79.39999999999999147, -34.70624999877097139, -101.7320508075688537 ) ) ;
#5380=CARTESIAN_POINT ( 'NONE',  ( -81.02178482187500208, -32.24062499938548854, -97.61286128772489690 ) ) ;
#5381=VECTOR ( 'NONE', #10112, 1000.000000000000000 ) ;
#5387=CARTESIAN_POINT ( 'NONE',  ( 81.02178482187500208, -33.44062499938548427, -97.61286128772489690 ) ) ;
#5390=ORIENTED_EDGE ( 'NONE', *, *, #10777, .F. ) ;
#5391=CARTESIAN_POINT ( 'NONE',  ( 85.40000000000000568, -32.73750000000000426, 101.7320508075688821 ) ) ;
#5395=ORIENTED_EDGE ( 'NONE', *, *, #18087, .T. ) ;
#5397=VECTOR ( 'NONE', #15463, 1000.000000000000000 ) ;
#5400=ORIENTED_EDGE ( 'NONE', *, *, #7252, .T. ) ;
#5401=CARTESIAN_POINT ( 'NONE',  ( -79.39999999999997726, -32.01330983656956164, -100.5399455202751966 ) ) ;
#5403=CARTESIAN_POINT ( 'NONE',  ( 83.90000000000000568, -33.22500000000000142, -97.40192378864668399 ) ) ;
#5404=CARTESIAN_POINT ( 'NONE',  ( 79.68596062386910717, -31.99999999999998579, -101.2782762865714972 ) ) ;
#5405=CARTESIAN_POINT ( 'NONE',  ( -85.15643035624999868, -32.54062499938548569, 98.40857419181659793 ) ) ;
#5407=CARTESIAN_POINT ( 'NONE',  ( -81.59615242270665192, -34.81740381056767575, -97.00000000000000000 ) ) ;
#5409=CARTESIAN_POINT ( 'NONE',  ( 83.90000000000000568, -34.06874999877096855, 102.5980762113533018 ) ) ;
#5410=DIRECTION ( 'NONE',  ( -1.000000000000000000, -0.000000000000000000, 0.000000000000000000 ) ) ;
#5411=CARTESIAN_POINT ( 'NONE',  ( 85.32499745258149915, -34.99999999999999289, 100.1587029275220857 ) ) ;
#5413=CARTESIAN_POINT ( 'NONE',  ( -84.28136653320150629, -32.00000000000001421, -102.0145392219080378 ) ) ;
#5415=CARTESIAN_POINT ( 'NONE',  ( 80.90000000000000568, -32.85000000000000142, 102.5980762113533018 ) ) ;
#5416=DIRECTION ( 'NONE',  ( 0.000000000000000000, -1.000000000000000000, 0.000000000000000000 ) ) ;
#5418=DIRECTION ( 'NONE',  ( 0.000000000000000000, 0.000000000000000000, 1.000000000000000000 ) ) ;
#5419=( BOUNDED_CURVE ( )  B_SPLINE_CURVE ( 2, ( #12902, #18869, #17206, #3529, #9483, #3810, #8120 ),
 .UNSPECIFIED., .F., .F. ) 
 B_SPLINE_CURVE_WITH_KNOTS ( ( 3, 2, 2, 3 ),
 ( 0.3702305174531529963, 0.3750000000000000000, 0.3888888888888888951, 0.3958333333333334259 ),
 .UNSPECIFIED. ) 
 CURVE ( )  GEOMETRIC_REPRESENTATION_ITEM ( )  RATIONAL_B_SPLINE_CURVE ( ( 0.9395835397632832375, 0.9539927561172885095, 1.000000000000000000, 0.8660254037844387076, 1.000000000000000000, 0.9330127018922185211, 0.9330127018922192983 ) ) 
 REPRESENTATION_ITEM ( '' )  );
#5424=CARTESIAN_POINT ( 'NONE',  ( -80.07894310789832559, -34.99999999999998579, -98.50261820439553162 ) ) ;
#5428=CARTESIAN_POINT ( 'NONE',  ( 83.20384757729338787, -32.10134618820330132, -102.9999999999999858 ) ) ;
#5429=CARTESIAN_POINT ( 'NONE',  ( 85.15643035624999868, -31.45312499938548356, 98.40857419181659793 ) ) ;
#5431=EDGE_CURVE ( 'NONE', #16462, #15718, #14014, .T. ) ;
#5434=CARTESIAN_POINT ( 'NONE',  ( -79.64356964374998427, -34.49062499938548854, -101.5914258081833879 ) ) ;
#5435=CARTESIAN_POINT ( 'NONE',  ( 79.64356964375001269, -32.57812499938548001, 101.5914258081833879 ) ) ;
#5436=CARTESIAN_POINT ( 'NONE',  ( 81.02178482187500208, -34.90312499938548285, -97.61286128772489690 ) ) ;
#5438=CARTESIAN_POINT ( 'NONE',  ( -83.77821517812500929, -33.81562499938548427, 97.61286128772489690 ) ) ;
#5439=CARTESIAN_POINT ( 'NONE',  ( 81.02178482187500208, -31.19062499938548427, -97.61286128772489690 ) ) ;
#5445=CARTESIAN_POINT ( 'NONE',  ( -85.15643035625001289, -33.29062499938547859, 99.99999999999998579 ) ) ;
#5446=CARTESIAN_POINT ( 'NONE',  ( -79.64356964375001269, -30.40312499938548285, 101.5914258081833879 ) ) ;
#5448=CARTESIAN_POINT ( 'NONE',  ( -85.03799702444352704, -32.00000000000000000, 99.18121545504318703 ) ) ;
#5455=CARTESIAN_POINT ( 'NONE',  ( -81.59615242270665192, -32.77634618820330559, 97.00000000000000000 ) ) ;
#5460=CARTESIAN_POINT ( 'NONE',  ( -79.68596062386970402, -32.00000000000002132, -98.72172371342720965 ) ) ;
#5461=CARTESIAN_POINT ( 'NONE',  ( 83.77821517812500929, -34.82812499938548711, -97.61286128772489690 ) ) ;
#5463=VERTEX_POINT ( 'NONE', #4647 ) ;
#5464=CARTESIAN_POINT ( 'NONE',  ( 83.90000000000000568, -33.61874999877097281, 102.5980762113533018 ) ) ;
#5470=CARTESIAN_POINT ( 'NONE',  ( -81.02178482187500208, -32.09062499938548285, -102.3871387122750889 ) ) ;
#5473=CARTESIAN_POINT ( 'NONE',  ( 85.15643035625001289, -33.81562499938548427, 98.40857419181659793 ) ) ;
#5474=CARTESIAN_POINT ( 'NONE',  ( -81.02178482187500208, -31.75312499938548427, -102.3871387122750889 ) ) ;
#5475=CARTESIAN_POINT ( 'NONE',  ( 83.90000000000000568, -33.22500000000000142, 102.5980762113533018 ) ) ;
#5479=CARTESIAN_POINT ( 'NONE',  ( -79.64356964374998427, -33.47812499938547859, -101.5914258081833879 ) ) ;
#5482=CARTESIAN_POINT ( 'NONE',  ( 80.90000000000000568, -31.59374999877097423, -102.5980762113533018 ) ) ;
#5485=VERTEX_POINT ( 'NONE', #3555 ) ;
#5486=CARTESIAN_POINT ( 'NONE',  ( 81.02178482187500208, -34.04062499938548569, -102.3871387122750889 ) ) ;
#5491=VERTEX_POINT ( 'NONE', #9512 ) ;
#5498=CARTESIAN_POINT ( 'NONE',  ( 79.39999999999999147, -32.47500000000000142, -99.99999999999998579 ) ) ;
#5499=CARTESIAN_POINT ( 'NONE',  ( -82.40000000000000568, -30.00000000000000355, 99.99999999999998579 ) ) ;
#5500=CARTESIAN_POINT ( 'NONE',  ( -79.64356964374999848, -32.27812499938548996, 99.99999999999998579 ) ) ;
#5506=CARTESIAN_POINT ( 'NONE',  ( -85.15643035625001289, -35.09062499938548285, 99.99999999999998579 ) ) ;
#5507=AXIS2_PLACEMENT_3D ( 'NONE', #11122, #6741, #6844 ) ;
#5518=AXIS2_PLACEMENT_3D ( 'NONE', #5499, #7330, #4208 ) ;
#5519=CARTESIAN_POINT ( 'NONE',  ( 83.90000000000000568, -32.26874999877097139, -97.40192378864668399 ) ) ;
#5520=CARTESIAN_POINT ( 'NONE',  ( 79.64356964374999848, -34.41562499938548569, 99.99999999999998579 ) ) ;
#5524=CARTESIAN_POINT ( 'NONE',  ( -82.39999999999999147, -34.64062499938548711, -96.81714838363319586 ) ) ;
#5525=CARTESIAN_POINT ( 'NONE',  ( 79.64356964375001269, -33.02812499938548285, 101.5914258081833879 ) ) ;
#5526=CARTESIAN_POINT ( 'NONE',  ( 81.02178482187500208, -33.25312499938548427, -102.3871387122750889 ) ) ;
#5528=CARTESIAN_POINT ( 'NONE',  ( -82.39999999999999147, -32.27812499938548285, 103.1828516163667899 ) ) ;
#5529=CARTESIAN_POINT ( 'NONE',  ( 83.77821517812500929, -31.86562499938548498, -102.3871387122750889 ) ) ;
#5530=VERTEX_POINT ( 'NONE', #6109 ) ;
#5535=CARTESIAN_POINT ( 'NONE',  ( -82.39999999999999147, -33.17812499938548854, 103.1828516163667899 ) ) ;
#5536=CARTESIAN_POINT ( 'NONE',  ( -81.02178482187500208, -31.64062499938548356, 97.61286128772489690 ) ) ;
#5539=FACE_OUTER_BOUND ( 'NONE', #11115, .T. ) ;
#5543=CARTESIAN_POINT ( 'NONE',  ( 82.40000000000001990, -32.53124999877097423, -103.0000000000000000 ) ) ;
#5547=CARTESIAN_POINT ( 'NONE',  ( 82.40000000000000568, -30.00000000000000355, -99.99999999999998579 ) ) ;
#5550=LINE ( 'NONE', #17172, #6198 ) ;
#5551=CARTESIAN_POINT ( 'NONE',  ( 82.40000000000001990, -34.55624999877097281, -97.00000000000000000 ) ) ;
#5552=DIRECTION ( 'NONE',  ( -0.000000000000000000, -1.000000000000000000, -0.000000000000000000 ) ) ;
#5553=CARTESIAN_POINT ( 'NONE',  ( 83.77821517812500929, -33.32812499938548711, -102.3871387122750889 ) ) ;
#5554=CARTESIAN_POINT ( 'NONE',  ( 82.39999999999999147, -32.98124999877096286, 96.99999999999998579 ) ) ;
#5556=CARTESIAN_POINT ( 'NONE',  ( 79.39999999999999147, -33.28124999877096712, 101.7320508075688821 ) ) ;
#5559=AXIS2_PLACEMENT_3D ( 'NONE', #9062, #8681, #10434 ) ;
#5563=CARTESIAN_POINT ( 'NONE',  ( 83.90000000000000568, -34.12500000000000000, 102.5980762113533018 ) ) ;
#5564=VERTEX_POINT ( 'NONE', #18707 ) ;
#5565=CARTESIAN_POINT ( 'NONE',  ( -81.02178482187500208, -33.59062499938548285, -97.61286128772489690 ) ) ;
#5571=CARTESIAN_POINT ( 'NONE',  ( -82.39999999999999147, -30.59062499938548640, -96.81714838363319586 ) ) ;
#5572=CARTESIAN_POINT ( 'NONE',  ( 79.39999999999999147, -34.72500000000000142, 99.99999999999998579 ) ) ;
#5576=CARTESIAN_POINT ( 'NONE',  ( -81.02178482187500208, -32.09062499938548285, -102.3871387122750889 ) ) ;
#5579=CARTESIAN_POINT ( 'NONE',  ( 83.90000000000000568, -32.26874999877097139, -97.40192378864668399 ) ) ;
#5581=ORIENTED_EDGE ( 'NONE', *, *, #18310, .T. ) ;
#5582=DIRECTION ( 'NONE',  ( 1.000000000000000000, -1.586032892321652285E-15, 0.000000000000000000 ) ) ;
#5585=PLANE ( 'NONE',  #17400 ) ;
#5588=VERTEX_POINT ( 'NONE', #3652 ) ;
#5590=CARTESIAN_POINT ( 'NONE',  ( -82.40000000000001990, -34.16250000000000853, -103.0000000000000000 ) ) ;
#5595=CARTESIAN_POINT ( 'NONE',  ( 82.39999999999999147, -32.36250000000000426, -96.53589838486223584 ) ) ;
#5596=EDGE_CURVE ( 'NONE', #8302, #8568, #9710, .T. ) ;
#5598=CARTESIAN_POINT ( 'NONE',  ( -79.64356964375001269, -31.79062499938548569, 98.40857419181659793 ) ) ;
#5603=EDGE_CURVE ( 'NONE', #14525, #15327, #14680, .T. ) ;
#5605=CARTESIAN_POINT ( 'NONE',  ( -81.02178482187500208, -34.79062499938548569, 97.61286128772489690 ) ) ;
#5606=CARTESIAN_POINT ( 'NONE',  ( -94.79999999999999716, -3.000000000000000000, -150.0000000000000000 ) ) ;
#5607=VERTEX_POINT ( 'NONE', #19156 ) ;
#5608=CARTESIAN_POINT ( 'NONE',  ( -81.02178482187500208, -31.34062499938548996, -97.61286128772489690 ) ) ;
#5610=CARTESIAN_POINT ( 'NONE',  ( 82.65333140691207348, -34.99995246259152992, 102.9892844631211943 ) ) ;
#5617=CARTESIAN_POINT ( 'NONE',  ( -79.39999999999999147, -33.82500000000000284, -99.99999999999998579 ) ) ;
#5618=CARTESIAN_POINT ( 'NONE',  ( 85.40000000000000568, -30.03750000000000497, 101.7320508075688679 ) ) ;
#5619=CARTESIAN_POINT ( 'NONE',  ( -82.40000000000001990, -34.55624999877097281, -103.0000000000000000 ) ) ;
#5622=CARTESIAN_POINT ( 'NONE',  ( -82.39999999999999147, -33.74062499938548854, -96.81714838363319586 ) ) ;
#5623=CARTESIAN_POINT ( 'NONE',  ( 85.15643035624999868, -33.70312499938548711, 98.40857419181659793 ) ) ;
#5624=CARTESIAN_POINT ( 'NONE',  ( 82.39999999999999147, -33.51562499938548001, -96.81714838363319586 ) ) ;
#5626=CARTESIAN_POINT ( 'NONE',  ( -82.39999999999999147, -33.62812499938548427, 103.1828516163667899 ) ) ;
#5627=CARTESIAN_POINT ( 'NONE',  ( 79.64356964375001269, -30.85312499938548569, -101.5914258081833879 ) ) ;
#5628=ORIENTED_EDGE ( 'NONE', *, *, #3556, .F. ) ;
#5629=CARTESIAN_POINT ( 'NONE',  ( 82.39999999999999147, -33.96562499938548285, 103.1828516163667899 ) ) ;
#5632=CARTESIAN_POINT ( 'NONE',  ( -85.15643035625001289, -32.39062499938548711, 99.99999999999998579 ) ) ;
#5633=CARTESIAN_POINT ( 'NONE',  ( -79.64356964375001269, -30.77812499938548285, 98.40857419181659793 ) ) ;
#5634=ORIENTED_EDGE ( 'NONE', *, *, #8204, .T. ) ;
#5637=CARTESIAN_POINT ( 'NONE',  ( 80.85389467647095785, -35.00000000000000000, -97.51091559654246055 ) ) ;
#5638=DIRECTION ( 'NONE',  ( -0.000000000000000000, -1.000000000000000000, -0.000000000000000000 ) ) ;
#5641=FACE_OUTER_BOUND ( 'NONE', #4086, .T. ) ;
#5643=CARTESIAN_POINT ( 'NONE',  ( 79.64356964374999848, -33.17812499938548854, 99.99999999999998579 ) ) ;
#5644=DIRECTION ( 'NONE',  ( 0.000000000000000000, -1.000000000000000000, 0.000000000000000000 ) ) ;
#5645=CARTESIAN_POINT ( 'NONE',  ( -83.20384757729337366, -32.55134618820330417, -97.00000000000000000 ) ) ;
#5646=CARTESIAN_POINT ( 'NONE',  ( 85.15643035625001289, -32.95312499938548711, -99.99999999999998579 ) ) ;
#5647=LINE ( 'NONE', #8277, #1494 ) ;
#5648=( BOUNDED_CURVE ( )  B_SPLINE_CURVE ( 2, ( #963, #5645, #8461, #7103, #17557, #4074, #17463, #1052, #11591 ),
 .UNSPECIFIED., .F., .F. ) 
 B_SPLINE_CURVE_WITH_KNOTS ( ( 3, 2, 2, 2, 3 ),
 ( 0.3958333333333334259, 0.4027777777777777901, 0.4166666666666666852, 0.4305555555555555802, 0.4374999999999999445 ),
 .UNSPECIFIED. ) 
 CURVE ( )  GEOMETRIC_REPRESENTATION_ITEM ( )  RATIONAL_B_SPLINE_CURVE ( ( 0.9330127018922192983, 0.9330127018922200755, 1.000000000000000000, 0.8660254037844387076, 1.000000000000000000, 0.8660254037844387076, 1.000000000000000000, 0.9330127018922198534, 0.9330127018922192983 ) ) 
 REPRESENTATION_ITEM ( '' )  );
#5649=VERTEX_POINT ( 'NONE', #17689 ) ;
#5650=CARTESIAN_POINT ( 'NONE',  ( 83.90000000000000568, -33.16874999877096286, 102.5980762113533018 ) ) ;
#5656=FACE_OUTER_BOUND ( 'NONE', #14229, .T. ) ;
#5658=CARTESIAN_POINT ( 'NONE',  ( -79.64356964374999848, -34.41562499938548569, -99.99999999999998579 ) ) ;
#5659=CARTESIAN_POINT ( 'NONE',  ( 82.40000000000001990, -33.26250000000000284, 103.0000000000000000 ) ) ;
#5661=FACE_OUTER_BOUND ( 'NONE', #15170, .T. ) ;
#5662=CARTESIAN_POINT ( 'NONE',  ( -79.39999999999999147, -35.11874999877096570, -99.99999999999998579 ) ) ;
#5663=CARTESIAN_POINT ( 'NONE',  ( -79.39999999999999147, -32.41874999877096997, -99.99999999999998579 ) ) ;
#5668=CARTESIAN_POINT ( 'NONE',  ( -83.77821517812500929, -32.46562499938548285, -102.3871387122750889 ) ) ;
#5671=CARTESIAN_POINT ( 'NONE',  ( 85.40000000000000568, -32.64374999877097139, -99.99999999999998579 ) ) ;
#5673=EDGE_LOOP ( 'NONE', ( #17275, #17497, #6927, #13 ) ) ;
#5678=ADVANCED_FACE ( 'NONE', ( #3214, #1752, #7519 ), #10551, .F. ) ;
#5685=CARTESIAN_POINT ( 'NONE',  ( 79.39999999999999147, -33.41250000000000142, -101.7320508075688537 ) ) ;
#5686=CARTESIAN_POINT ( 'NONE',  ( 80.80636817121802551, -31.99999999999999289, -102.4696265554868120 ) ) ;
#5687=CARTESIAN_POINT ( 'NONE',  ( -79.64356964374999848, -31.37812499938548427, 99.99999999999998579 ) ) ;
#5689=DIRECTION ( 'NONE',  ( 0.000000000000000000, 0.000000000000000000, -1.000000000000000000 ) ) ;
#5691=CARTESIAN_POINT ( 'NONE',  ( 96.99999999999994316, -29.80000000000000426, 150.0000000000000000 ) ) ;
#5694=CARTESIAN_POINT ( 'NONE',  ( -82.39999999999999147, -32.05312499938548854, -103.1828516163667899 ) ) ;
#5695=DIRECTION ( 'NONE',  ( 0.000000000000000000, 0.000000000000000000, -1.000000000000000000 ) ) ;
#5703=ORIENTED_EDGE ( 'NONE', *, *, #17732, .T. ) ;
#5706=CARTESIAN_POINT ( 'NONE',  ( -84.42750213138106119, -35.00000000000000711, -102.2200415044235768 ) ) ;
#5708=CARTESIAN_POINT ( 'NONE',  ( 82.39999999999999147, -34.30312499938548143, 103.1828516163667899 ) ) ;
#5714=CARTESIAN_POINT ( 'NONE',  ( 85.40000000000000568, -33.09374999877096712, -99.99999999999998579 ) ) ;
#5715=CARTESIAN_POINT ( 'NONE',  ( 82.39999999999999147, -32.50312499938548427, -96.81714838363319586 ) ) ;
#5717=CARTESIAN_POINT ( 'NONE',  ( -81.02178482187500208, -32.99062499938548854, 97.61286128772489690 ) ) ;
#5718=CARTESIAN_POINT ( 'NONE',  ( 82.39999999999999147, -31.37812499938548427, -103.1828516163667899 ) ) ;
#5721=CARTESIAN_POINT ( 'NONE',  ( 85.15643035624999868, -34.71562499938548285, 98.40857419181659793 ) ) ;
#5722=CARTESIAN_POINT ( 'NONE',  ( 82.40000000000000568, -33.71249999999998437, -96.99999999999998579 ) ) ;
#5725=CARTESIAN_POINT ( 'NONE',  ( -83.77821517812500929, -32.46562499938548285, 97.61286128772489690 ) ) ;
#5726=ORIENTED_EDGE ( 'NONE', *, *, #18216, .T. ) ;
#5729=CARTESIAN_POINT ( 'NONE',  ( 79.73531137350353504, -34.99999999999998579, -98.99456257074372445 ) ) ;
#5731=CARTESIAN_POINT ( 'NONE',  ( -82.40000000000000568, -34.61250000000001137, 97.00000000000000000 ) ) ;
#5735=CARTESIAN_POINT ( 'NONE',  ( 79.64356964374999848, -32.27812499938548996, 99.99999999999998579 ) ) ;
#5737=CARTESIAN_POINT ( 'NONE',  ( 85.15643035624999868, -33.36562499938548854, -101.5914258081833879 ) ) ;
#5738=CARTESIAN_POINT ( 'NONE',  ( -82.39999999999999147, -32.39062499938548001, -96.81714838363319586 ) ) ;
#5740=CARTESIAN_POINT ( 'NONE',  ( 79.39999999999999147, -33.73124999877096997, 101.7320508075688821 ) ) ;
#5742=CARTESIAN_POINT ( 'NONE',  ( 82.40000000000001990, -32.75624999877096855, 103.0000000000000000 ) ) ;
#5744=CARTESIAN_POINT ( 'NONE',  ( 83.92761994969310990, -32.00000000000000711, 102.3311504458557266 ) ) ;
#5746=CARTESIAN_POINT ( 'NONE',  ( -85.15643035624999868, -34.67812499938548143, -101.5914258081833879 ) ) ;
#5750=CARTESIAN_POINT ( 'NONE',  ( -85.15643035624999868, -30.66562499938548569, -98.40857419181659793 ) ) ;
#5751=CARTESIAN_POINT ( 'NONE',  ( -81.90908125315185373, -32.00000000000000000, -102.8381494550067146 ) ) ;
#5752=CARTESIAN_POINT ( 'NONE',  ( -85.40000000000000568, -31.33124999877096428, -101.7320508075688679 ) ) ;
#5756=CARTESIAN_POINT ( 'NONE',  ( -85.15643035625001289, -33.70312499938548711, -98.40857419181659793 ) ) ;
#5757=CARTESIAN_POINT ( 'NONE',  ( 80.90000000000000568, -32.55000000000000426, -102.5980762113533018 ) ) ;
#5759=CARTESIAN_POINT ( 'NONE',  ( 82.39999999999999147, -32.75624999877096855, -96.53589838486223584 ) ) ;
#5762=CARTESIAN_POINT ( 'NONE',  ( 83.77821517812500929, -34.11562499938548854, -102.3871387122750889 ) ) ;
#5774=FACE_OUTER_BOUND ( 'NONE', #4295, .T. ) ;
#5776=CARTESIAN_POINT ( 'NONE',  ( -83.77821517812500929, -32.87812499938548427, 102.3871387122750889 ) ) ;
#5778=FACE_OUTER_BOUND ( 'NONE', #6806, .T. ) ;
#5781=CARTESIAN_POINT ( 'NONE',  ( -83.77821517812500929, -34.56562499938548427, 102.3871387122750889 ) ) ;
#5783=VERTEX_POINT ( 'NONE', #595 ) ;
#5785=CARTESIAN_POINT ( 'NONE',  ( -85.15643035624999868, -35.16562499938547859, -98.40857419181659793 ) ) ;
#5792=ADVANCED_FACE ( 'NONE', ( #3411 ), #15625, .T. ) ;
#5795=EDGE_CURVE ( 'NONE', #12381, #14868, #11628, .T. ) ;
#5797=CARTESIAN_POINT ( 'NONE',  ( -85.39999999999999147, -34.97364041986484295, -101.0919042218176287 ) ) ;
#5799=EDGE_CURVE ( 'NONE', #5933, #17663, #13613, .T. ) ;
#5800=CYLINDRICAL_SURFACE ( 'NONE', #19120, 3.000000000000002665 ) ;
#5801=CARTESIAN_POINT ( 'NONE',  ( 83.90000000000000568, -30.37500000000000355, 97.40192378864668399 ) ) ;
#5802=CARTESIAN_POINT ( 'NONE',  ( 82.40000000000001990, -34.16250000000000853, -97.00000000000000000 ) ) ;
#5807=CARTESIAN_POINT ( 'NONE',  ( 85.15643035624999868, -34.67812499938548143, 101.5914258081833879 ) ) ;
#5808=CARTESIAN_POINT ( 'NONE',  ( 82.39999999999999147, -30.25312499938548783, -96.81714838363319586 ) ) ;
#5809=EDGE_CURVE ( 'NONE', #11864, #5485, #16801, .T. ) ;
#5811=CARTESIAN_POINT ( 'NONE',  ( 85.40000000000000568, -34.91250000000000142, -101.7320508075688821 ) ) ;
#5812=CARTESIAN_POINT ( 'NONE',  ( 79.64356964374999848, -33.96562499938548285, -99.99999999999998579 ) ) ;
#5815=CARTESIAN_POINT ( 'NONE',  ( 79.64356964375001269, -35.01562499938548711, 98.40857419181659793 ) ) ;
#5818=VECTOR ( 'NONE', #10453, 1000.000000000000000 ) ;
#5819=CARTESIAN_POINT ( 'NONE',  ( -85.15643035625001289, -32.84062499938548285, 99.99999999999998579 ) ) ;
#5821=CARTESIAN_POINT ( 'NONE',  ( -84.25709831968909214, -35.00000000000001421, 102.1174602701862000 ) ) ;
#5823=CARTESIAN_POINT ( 'NONE',  ( 79.59365286754818669, -35.00000000000000711, -99.92898555286036810 ) ) ;
#5827=CARTESIAN_POINT ( 'NONE',  ( -81.59615242270660929, -32.32634618820329564, 96.99999999999997158 ) ) ;
#5830=CARTESIAN_POINT ( 'NONE',  ( 85.15643035625001289, -32.95312499938548711, 99.99999999999998579 ) ) ;
#5831=FACE_OUTER_BOUND ( 'NONE', #12802, .T. ) ;
#5833=CARTESIAN_POINT ( 'NONE',  ( 82.39999999999999147, -34.41562499938547859, -96.81714838363319586 ) ) ;
#5834=CARTESIAN_POINT ( 'NONE',  ( -82.39999999999999147, -31.04062499938548569, -96.81714838363319586 ) ) ;
#5836=CARTESIAN_POINT ( 'NONE',  ( 79.39999999999999147, -33.76874999877097139, 99.99999999999998579 ) ) ;
#5840=CARTESIAN_POINT ( 'NONE',  ( -83.77821517812500929, -31.52812499938548996, 102.3871387122750889 ) ) ;
#5841=CARTESIAN_POINT ( 'NONE',  ( 80.24181665645362216, -31.99999999999999289, 102.0230471654357700 ) ) ;
#5843=CARTESIAN_POINT ( 'NONE',  ( -83.77821517812500929, -34.56562499938548427, -97.61286128772489690 ) ) ;
#5844=AXIS2_PLACEMENT_3D ( 'NONE', #3295, #7601, #17779 ) ;
#5848=CARTESIAN_POINT ( 'NONE',  ( -83.77821517812500929, -32.42812499938548854, -97.61286128772489690 ) ) ;
#5849=CARTESIAN_POINT ( 'NONE',  ( -80.60346964438549833, -31.99999999999999289, -102.3251727584376312 ) ) ;
#5850=CARTESIAN_POINT ( 'NONE',  ( -85.40000000000000568, -32.19374999877096855, -99.99999999999998579 ) ) ;
#5855=CARTESIAN_POINT ( 'NONE',  ( -85.40000000000000568, -33.54374999877096286, 99.99999999999998579 ) ) ;
#5858=CARTESIAN_POINT ( 'NONE',  ( 85.40000000000000568, -32.15624999877096712, -101.7320508075688679 ) ) ;
#5859=VECTOR ( 'NONE', #11257, 1000.000000000000000 ) ;
#5861=VERTEX_POINT ( 'NONE', #12682 ) ;
#5870=CARTESIAN_POINT ( 'NONE',  ( -82.85293433259495544, -32.00000000000000000, 97.19890519204300006 ) ) ;
#5873=CARTESIAN_POINT ( 'NONE',  ( -80.07894310789832559, -35.00000000000000711, 101.4973817956044684 ) ) ;
#5874=DIRECTION ( 'NONE',  ( 0.000000000000000000, 0.000000000000000000, 1.000000000000000000 ) ) ;
#5878=CARTESIAN_POINT ( 'NONE',  ( -85.15643035625001289, -34.30312499938548854, 99.99999999999998579 ) ) ;
#5887=CARTESIAN_POINT ( 'NONE',  ( -82.39999999999999147, -35.09062499938548285, -96.81714838363319586 ) ) ;
#5889=VECTOR ( 'NONE', #3397, 1000.000000000000000 ) ;
#5891=CARTESIAN_POINT ( 'NONE',  ( -82.40000000000001990, -32.75624999877096855, 97.00000000000000000 ) ) ;
#5898=ORIENTED_EDGE ( 'NONE', *, *, #12830, .T. ) ;
#5901=CARTESIAN_POINT ( 'NONE',  ( -79.39999999999999147, -31.55624999877096926, 101.7320508075688537 ) ) ;
#5902=CARTESIAN_POINT ( 'NONE',  ( 82.39999999999999147, -33.03750000000000142, 96.53589838486223584 ) ) ;
#5903=LINE ( 'NONE', #5994, #10857 ) ;
#5906=CARTESIAN_POINT ( 'NONE',  ( 82.39999999999999147, -34.97812499938547859, 96.81714838363319586 ) ) ;
#5907=EDGE_CURVE ( 'NONE', #422, #8584, #11400, .T. ) ;
#5908=CARTESIAN_POINT ( 'NONE',  ( 83.77821517812500929, -30.21562499938548285, -97.61286128772489690 ) ) ;
#5911=CARTESIAN_POINT ( 'NONE',  ( 85.39999999999999147, -34.97364041986484295, -98.90809577818235709 ) ) ;
#5912=CARTESIAN_POINT ( 'NONE',  ( 79.64356964375001269, -32.57812499938548001, -98.40857419181659793 ) ) ;
#5915=CARTESIAN_POINT ( 'NONE',  ( 81.59615242270662350, -33.91740381056766296, -103.0000000000000000 ) ) ;
#5917=CARTESIAN_POINT ( 'NONE',  ( -85.40000000000000568, -31.35000000000000142, 99.99999999999998579 ) ) ;
#5922=( BOUNDED_SURFACE ( )  B_SPLINE_SURFACE ( 1, 2, ( 
 ( #2315, #10920, #2134, #13944, #18645, #12776, #14230, #772, #4979, #5071, #15417, #2028, #3881, #584, #12482, #11310, #9844, #679, #18745, #2413, #14136, #9550, #8281, #5364, #17277, #14328, #12672, #3590, #967, #18450, #16978, #15616, #8091, #14044, #6630, #12579, #5268, #5162, #11108, #17076, #9656, #11213, #4174, #15998, #7292, #18841, #7198, #7107, #2601, #2700, #6922, #17368, #14515, #8562, #3980, #15902, #18935, #13063, #1246, #16197, #2804, #13147, #2898, #19028, #12965, #9945, #8756, #14615, #7010, #17467, #8658, #14708, #13247, #4367, #5650, #1346, #2508, #5556, #19219, #11595, #1149, #8465, #19122, #16094, #17760, #17563, #5464, #10135, #12870, #5740, #5836, #11689, #17658, #11505, #8852, #4078, #1056, #11407, #14808, #4270, #10327, #10231, #16286, #10039, #11788, #14421, #15194, #15103, #4761, #1434, #15010, #10704, #369, #5934, #3274, #7488, #7584, #12173, #13729, #13443, #16481, #2989, #3085, #16669, #17695, #10513, #8944, #7673, #1812, #9232, #9139, #7389, #77, #11881, #13350 ),
 ( #12273, #9046, #7776, #10798, #10611, #17945, #6319, #18236, #18141, #4853, #16578, #11977, #16761, #3377, #6030, #4661, #1628, #4557, #17849, #1718, #13534, #9328, #173, #6124, #4462, #10416, #12075, #14911, #13628, #16379, #1540, #272, #18051, #3178, #6225, #7869, #6807, #12367, #18334, #14207, #12753, #3568, #17152, #5343, #5140, #12459, #18622, #3760, #6704, #844, #11085, #6514, #5240, #18722, #557, #18523, #5046, #18426, #4953, #3667, #10988, #2293, #16956, #14021, #9527, #17055, #11283, #12648, #656, #17251, #3857, #12552, #15493, #15689, #13821, #15594, #2105, #8066, #9631, #15293, #6411, #6604, #2202, #10895, #16863, #7964, #8163, #14112, #11189, #9725, #749, #1907, #8257, #2005, #3469, #463, #9426, #15395, #13919, #5629, #11670, #10209, #7271, #8541, #17635, #18819, #15883, #4249, #14492, #18912, #6899, #17538, #19009, #1323, #17446, #8353, #10016, #9820, #11575, #5721, #8635, #2676, #8445, #11764, #2487, #3956, #15782, #5815, #1123, #13226, #15974, #19199, #12941, #4153, #10114 ) ),
 .UNSPECIFIED., .F., .F., .F. ) 
 B_SPLINE_SURFACE_WITH_KNOTS ( ( 2, 2 ),
 ( 3, 2, 2, 2, 2, 2, 2, 2, 2, 2, 2, 2, 2, 2, 2, 2, 2, 2, 2, 2, 2, 2, 2, 2, 2, 2, 2, 2, 2, 2, 2, 2, 2, 2, 2, 2, 2, 2, 2, 2, 2, 2, 2, 2, 2, 2, 2, 2, 2, 2, 2, 2, 2, 2, 2, 2, 2, 2, 2, 2, 2, 2, 2, 2, 2, 2, 2, 3 ),
 ( 0.000000000000000000, 1.000000000000000000 ),
 ( 0.000000000000000000, 0.01388888888888888812, 0.02777777777777777624, 0.04166666666666666435, 0.05555555555555555247, 0.06944444444444444753, 0.08333333333333332871, 0.09722222222222222376, 0.1111111111111111049, 0.1250000000000000000, 0.1388888888888888951, 0.1527777777777777901, 0.1666666666666666574, 0.1805555555555555525, 0.1944444444444444475, 0.2083333333333333426, 0.2222222222222222099, 0.2361111111111111049, 0.2500000000000000000, 0.2638888888888888951, 0.2777777777777777901, 0.2916666666666666852, 0.3055555555555555802, 0.3194444444444444198, 0.3333333333333333148, 0.3472222222222222099, 0.3611111111111111049, 0.3750000000000000000, 0.3888888888888888951, 0.4027777777777777901, 0.4166666666666666852, 0.4305555555555555802, 0.4444444444444444198, 0.4583333333333333148, 0.4722222222222222099, 0.4861111111111111049, 0.5000000000000000000, 0.5138888888888888395, 0.5277777777777777901, 0.5416666666666666297, 0.5555555555555555802, 0.5694444444444444198, 0.5833333333333333703, 0.5972222222222222099, 0.6111111111111111605, 0.6250000000000000000, 0.6388888888888888395, 0.6527777777777777901, 0.6666666666666666297, 0.6805555555555555802, 0.6944444444444444198, 0.7083333333333333703, 0.7222222222222222099, 0.7361111111111111605, 0.7500000000000000000, 0.7638888888888888395, 0.7777777777777777901, 0.7916666666666666297, 0.8055555555555555802, 0.8194444444444444198, 0.8333333333333333703, 0.8472222222222222099, 0.8611111111111111605, 0.8750000000000000000, 0.8888888888888888395, 0.9027777777777777901, 0.9166666666666666297, 0.9258785144422092550 ),
 .UNSPECIFIED. ) 
 GEOMETRIC_REPRESENTATION_ITEM ( )  RATIONAL_B_SPLINE_SURFACE ( (
 ( 1.000000000000000000, 0.8660254037844387076, 1.000000000000000000, 0.8660254037844387076, 1.000000000000000000, 0.8660254037844387076, 1.000000000000000000, 0.8660254037844387076, 1.000000000000000000, 0.8660254037844387076, 1.000000000000000000, 0.8660254037844387076, 1.000000000000000000, 0.8660254037844387076, 1.000000000000000000, 0.8660254037844387076, 1.000000000000000000, 0.8660254037844387076, 1.000000000000000000, 0.8660254037844387076, 1.000000000000000000, 0.8660254037844387076, 1.000000000000000000, 0.8660254037844387076, 1.000000000000000000, 0.8660254037844387076, 1.000000000000000000, 0.8660254037844387076, 1.000000000000000000, 0.8660254037844387076, 1.000000000000000000, 0.8660254037844387076, 1.000000000000000000, 0.8660254037844387076, 1.000000000000000000, 0.8660254037844387076, 1.000000000000000000, 0.8660254037844387076, 1.000000000000000000, 0.8660254037844387076, 1.000000000000000000, 0.8660254037844387076, 1.000000000000000000, 0.8660254037844387076, 1.000000000000000000, 0.8660254037844387076, 1.000000000000000000, 0.8660254037844387076, 1.000000000000000000, 0.8660254037844387076, 1.000000000000000000, 0.8660254037844387076, 1.000000000000000000, 0.8660254037844387076, 1.000000000000000000, 0.8660254037844387076, 1.000000000000000000, 0.8660254037844387076, 1.000000000000000000, 0.8660254037844387076, 1.000000000000000000, 0.8660254037844387076, 1.000000000000000000, 0.8660254037844387076, 1.000000000000000000, 0.8660254037844387076, 1.000000000000000000, 0.8660254037844387076, 1.000000000000000000, 0.8660254037844387076, 1.000000000000000000, 0.8660254037844387076, 1.000000000000000000, 0.8660254037844387076, 1.000000000000000000, 0.8660254037844387076, 1.000000000000000000, 0.8660254037844387076, 1.000000000000000000, 0.8660254037844387076, 1.000000000000000000, 0.8660254037844387076, 1.000000000000000000, 0.8660254037844387076, 1.000000000000000000, 0.8660254037844387076, 1.000000000000000000, 0.8660254037844387076, 1.000000000000000000, 0.8660254037844387076, 1.000000000000000000, 0.8660254037844387076, 1.000000000000000000, 0.8660254037844387076, 1.000000000000000000, 0.8660254037844387076, 1.000000000000000000, 0.8660254037844387076, 1.000000000000000000, 0.8660254037844387076, 1.000000000000000000, 0.8660254037844387076, 1.000000000000000000, 0.8660254037844387076, 1.000000000000000000, 0.8660254037844387076, 1.000000000000000000, 0.8660254037844387076, 1.000000000000000000, 0.8660254037844387076, 1.000000000000000000, 0.8660254037844387076, 1.000000000000000000, 0.8660254037844387076, 1.000000000000000000, 0.8660254037844387076, 1.000000000000000000, 0.8660254037844387076, 1.000000000000000000, 0.8660254037844387076, 1.000000000000000000, 0.8660254037844387076, 1.000000000000000000, 0.8660254037844387076, 1.000000000000000000, 0.8660254037844387076, 1.000000000000000000, 0.8660254037844387076, 1.000000000000000000, 0.8660254037844387076, 1.000000000000000000, 0.8660254037844387076, 1.000000000000000000, 0.9111409417988175496, 0.9401539645359766606),
 ( 1.000000000000000000, 0.8660254037844387076, 1.000000000000000000, 0.8660254037844387076, 1.000000000000000000, 0.8660254037844387076, 1.000000000000000000, 0.8660254037844387076, 1.000000000000000000, 0.8660254037844387076, 1.000000000000000000, 0.8660254037844387076, 1.000000000000000000, 0.8660254037844387076, 1.000000000000000000, 0.8660254037844387076, 1.000000000000000000, 0.8660254037844387076, 1.000000000000000000, 0.8660254037844387076, 1.000000000000000000, 0.8660254037844387076, 1.000000000000000000, 0.8660254037844387076, 1.000000000000000000, 0.8660254037844387076, 1.000000000000000000, 0.8660254037844387076, 1.000000000000000000, 0.8660254037844387076, 1.000000000000000000, 0.8660254037844387076, 1.000000000000000000, 0.8660254037844387076, 1.000000000000000000, 0.8660254037844387076, 1.000000000000000000, 0.8660254037844387076, 1.000000000000000000, 0.8660254037844387076, 1.000000000000000000, 0.8660254037844387076, 1.000000000000000000, 0.8660254037844387076, 1.000000000000000000, 0.8660254037844387076, 1.000000000000000000, 0.8660254037844387076, 1.000000000000000000, 0.8660254037844387076, 1.000000000000000000, 0.8660254037844387076, 1.000000000000000000, 0.8660254037844387076, 1.000000000000000000, 0.8660254037844387076, 1.000000000000000000, 0.8660254037844387076, 1.000000000000000000, 0.8660254037844387076, 1.000000000000000000, 0.8660254037844387076, 1.000000000000000000, 0.8660254037844387076, 1.000000000000000000, 0.8660254037844387076, 1.000000000000000000, 0.8660254037844387076, 1.000000000000000000, 0.8660254037844387076, 1.000000000000000000, 0.8660254037844387076, 1.000000000000000000, 0.8660254037844387076, 1.000000000000000000, 0.8660254037844387076, 1.000000000000000000, 0.8660254037844387076, 1.000000000000000000, 0.8660254037844387076, 1.000000000000000000, 0.8660254037844387076, 1.000000000000000000, 0.8660254037844387076, 1.000000000000000000, 0.8660254037844387076, 1.000000000000000000, 0.8660254037844387076, 1.000000000000000000, 0.8660254037844387076, 1.000000000000000000, 0.8660254037844387076, 1.000000000000000000, 0.8660254037844387076, 1.000000000000000000, 0.8660254037844387076, 1.000000000000000000, 0.8660254037844387076, 1.000000000000000000, 0.8660254037844387076, 1.000000000000000000, 0.8660254037844387076, 1.000000000000000000, 0.8660254037844387076, 1.000000000000000000, 0.8660254037844387076, 1.000000000000000000, 0.8660254037844387076, 1.000000000000000000, 0.8660254037844387076, 1.000000000000000000, 0.8660254037844387076, 1.000000000000000000, 0.8660254037844387076, 1.000000000000000000, 0.8660254037844387076, 1.000000000000000000, 0.8660254037844387076, 1.000000000000000000, 0.8660254037844387076, 1.000000000000000000, 0.8660254037844387076, 1.000000000000000000, 0.8660254037844387076, 1.000000000000000000, 0.8660254037844387076, 1.000000000000000000, 0.8660254037844387076, 1.000000000000000000, 0.8660254037844387076, 1.000000000000000000, 0.8660254037844387076, 1.000000000000000000, 0.9111409417988175496, 0.9401539645359766606) ) ) 
 REPRESENTATION_ITEM ( '' )  SURFACE ( )  );
#5927=CARTESIAN_POINT ( 'NONE',  ( 84.28136653320183314, -32.00000000000000711, 102.0145392219077394 ) ) ;
#5928=CARTESIAN_POINT ( 'NONE',  ( 85.15643035624999868, -32.09062499938548996, 101.5914258081833879 ) ) ;
#5929=CARTESIAN_POINT ( 'NONE',  ( 82.40000000000000568, -32.08124999877097139, 97.00000000000000000 ) ) ;
#5930=PLANE ( 'NONE',  #1212 ) ;
#5931=CARTESIAN_POINT ( 'NONE',  ( -82.39999999999999147, -32.84062499938548996, 103.1828516163667899 ) ) ;
#5932=CARTESIAN_POINT ( 'NONE',  ( -81.02178482187500208, -31.90312499938548996, -97.61286128772489690 ) ) ;
#5933=VERTEX_POINT ( 'NONE', #1258 ) ;
#5934=CARTESIAN_POINT ( 'NONE',  ( 79.39999999999999147, -34.63124999877096855, 101.7320508075688821 ) ) ;
#5937=CARTESIAN_POINT ( 'NONE',  ( -82.39999999999999147, -32.16562499938549280, 96.81714838363319586 ) ) ;
#5938=FACE_OUTER_BOUND ( 'NONE', #4970, .T. ) ;
#5940=CARTESIAN_POINT ( 'NONE',  ( -79.64356964375001269, -33.92812499938548854, -101.5914258081833879 ) ) ;
#5942=DIRECTION ( 'NONE',  ( 0.000000000000000000, 0.000000000000000000, 1.000000000000000000 ) ) ;
#5944=CARTESIAN_POINT ( 'NONE',  ( -83.77821517812500929, -33.47812499938548569, -102.3871387122750889 ) ) ;
#5946=CARTESIAN_POINT ( 'NONE',  ( -79.39999999999999147, -31.51874999877096784, -99.99999999999998579 ) ) ;
#5950=CARTESIAN_POINT ( 'NONE',  ( -83.77821517812500929, -34.26562499938548711, -102.3871387122750889 ) ) ;
#5951=CARTESIAN_POINT ( 'NONE',  ( 83.77821517812500929, -32.46562499938548285, 102.3871387122750889 ) ) ;
#5953=CARTESIAN_POINT ( 'NONE',  ( 82.40000000000000568, -30.00000000000000355, 99.99999999999998579 ) ) ;
#5954=CARTESIAN_POINT ( 'NONE',  ( 79.39999999999999147, -34.66874999877096997, -99.99999999999998579 ) ) ;
#5956=EDGE_LOOP ( 'NONE', ( #9662, #13188, #16962, #8487 ) ) ;
#5957=CARTESIAN_POINT ( 'NONE',  ( 83.77821517812500929, -34.56562499938548427, -102.3871387122750889 ) ) ;
#5962=ADVANCED_FACE ( 'NONE', ( #18849 ), #7204, .T. ) ;
#5963=EDGE_LOOP ( 'NONE', ( #19204, #3666, #18653, #11049, #6520, #5395, #9978, #8117, #17109, #8816, #2180, #2063, #16723, #1722, #11580, #4319, #5273 ) ) ;
#5968=ORIENTED_EDGE ( 'NONE', *, *, #6579, .F. ) ;
#5969=CARTESIAN_POINT ( 'NONE',  ( 82.40000000000000568, -32.30624999877097281, -97.00000000000000000 ) ) ;
#5970=CARTESIAN_POINT ( 'NONE',  ( -94.79999999999999716, -29.80000000000000426, 150.0000000000000000 ) ) ;
#5971=CARTESIAN_POINT ( 'NONE',  ( -79.64356964374999848, -33.62812499938548427, 99.99999999999998579 ) ) ;
#5976=CARTESIAN_POINT ( 'NONE',  ( -81.59615242270665192, -33.28259618943233278, 97.00000000000000000 ) ) ;
#5977=CARTESIAN_POINT ( 'NONE',  ( 94.79999999999991189, -3.000000000000000000, 150.0000000000000000 ) ) ;
#5978=CARTESIAN_POINT ( 'NONE',  ( -85.40000000000000568, -34.50000000000000000, -99.99999999999998579 ) ) ;
#5980=CARTESIAN_POINT ( 'NONE',  ( -85.15643035624999868, -34.15312499938548285, -98.40857419181659793 ) ) ;
#5981=CARTESIAN_POINT ( 'NONE',  ( -83.90000000000000568, -33.52499999999999858, 102.5980762113533018 ) ) ;
#5982=DIRECTION ( 'NONE',  ( 0.000000000000000000, -1.000000000000000000, 0.000000000000000000 ) ) ;
#5989=ORIENTED_EDGE ( 'NONE', *, *, #892, .F. ) ;
#5992=CARTESIAN_POINT ( 'NONE',  ( -82.39999999999999147, -31.18124999877096926, 103.4641016151377499 ) ) ;
#5993=CARTESIAN_POINT ( 'NONE',  ( 79.39999999999999147, -32.51250000000000284, 98.26794919243113213 ) ) ;
#5994=CARTESIAN_POINT ( 'NONE',  ( 69.99999999999998579, -34.99999999999999289, 150.0000000000000000 ) ) ;
#5997=CARTESIAN_POINT ( 'NONE',  ( 83.20384757729335945, -33.00134618820329990, -102.9999999999999858 ) ) ;
#6000=CARTESIAN_POINT ( 'NONE',  ( 85.15643035624999868, -31.97812499938548925, -98.40857419181659793 ) ) ;
#6001=ORIENTED_EDGE ( 'NONE', *, *, #2788, .F. ) ;
#6003=CARTESIAN_POINT ( 'NONE',  ( 83.77821517812500929, -33.81562499938548427, -97.61286128772489690 ) ) ;
#6007=CARTESIAN_POINT ( 'NONE',  ( -82.39999999999999147, -31.46250000000000568, 96.53589838486223584 ) ) ;
#6012=ADVANCED_FACE ( 'NONE', ( #11416 ), #2610, .F. ) ;
#6013=B_SPLINE_CURVE_WITH_KNOTS ( 'NONE', 3,
 ( #10868, #13888, #13795, #6384, #6097, #9109, #10485, #16642, #3445, #15073, #3244, #1693, #16550, #12045, #12147, #13600, #16839, #6292 ),
 .UNSPECIFIED., .F., .F.,
 ( 4, 2, 2, 2, 2, 2, 2, 2, 4 ),
 ( 0.000000000000000000, 0.0007089252359966436746, 0.001417850471993287349, 0.002126775707989931024, 0.002835700943986574699, 0.003544626179983218373, 0.004253551415979862048, 0.004962476651976506156, 0.005671401887973149397 ),
 .UNSPECIFIED. ) ;
#6014=EDGE_CURVE ( 'NONE', #7316, #2256, #14336, .T. ) ;
#6019=LINE ( 'NONE', #7573, #1801 ) ;
#6022=CARTESIAN_POINT ( 'NONE',  ( 83.77821517812500929, -32.87812499938548427, 97.61286128772489690 ) ) ;
#6023=EDGE_CURVE ( 'NONE', #12074, #18433, #5275, .T. ) ;
#6025=CARTESIAN_POINT ( 'NONE',  ( -82.39999999999999147, -32.36250000000000426, -102.9999999999999858 ) ) ;
#6026=CARTESIAN_POINT ( 'NONE',  ( -79.64356964374998427, -32.69062499938548427, 98.40857419181659793 ) ) ;
#6029=ORIENTED_EDGE ( 'NONE', *, *, #5324, .F. ) ;
#6030=CARTESIAN_POINT ( 'NONE',  ( 83.77821517812500929, -30.77812499938548640, 102.3871387122750889 ) ) ;
#6031=LINE ( 'NONE', #174, #13336 ) ;
#6032=CARTESIAN_POINT ( 'NONE',  ( -94.79999999999999716, 0.000000000000000000, 150.0000000000000000 ) ) ;
#6034=CARTESIAN_POINT ( 'NONE',  ( -81.02178482187500208, -32.35312499938548569, 102.3871387122750889 ) ) ;
#6036=CARTESIAN_POINT ( 'NONE',  ( -84.70388354820684640, -35.00002705695768412, -101.9214814096701076 ) ) ;
#6037=ORIENTED_EDGE ( 'NONE', *, *, #3662, .F. ) ;
#6038=CARTESIAN_POINT ( 'NONE',  ( -79.39999999999999147, -31.61250000000000071, -98.26794919243113213 ) ) ;
#6042=CARTESIAN_POINT ( 'NONE',  ( -85.15643035624999868, -32.99062499938548854, -101.5914258081833879 ) ) ;
#6043=EDGE_CURVE ( 'NONE', #4397, #17663, #12973, .T. ) ;
#6049=CARTESIAN_POINT ( 'NONE',  ( 82.39999999999999147, -33.17812499938548854, 96.81714838363319586 ) ) ;
#6052=CARTESIAN_POINT ( 'NONE',  ( 79.39999999999999147, -33.35624999877097707, -101.7320508075688537 ) ) ;
#6054=ORIENTED_EDGE ( 'NONE', *, *, #9967, .T. ) ;
#6057=EDGE_CURVE ( 'NONE', #6753, #18433, #13151, .T. ) ;
#6062=EDGE_LOOP ( 'NONE', ( #17590, #15416, #11161, #11195, #4194, #6758, #3991, #6547, #9540, #11265, #14050, #13820, #11343, #17198, #14327, #490, #13043 ) ) ;
#6065=CARTESIAN_POINT ( 'NONE',  ( -83.90000000000000568, -33.52499999999999858, -97.40192378864668399 ) ) ;
#6066=EDGE_LOOP ( 'NONE', ( #17040, #2060, #18457, #8243 ) ) ;
#6069=CARTESIAN_POINT ( 'NONE',  ( -79.64356964375001269, -34.04062499938549280, 98.40857419181659793 ) ) ;
#6075=CARTESIAN_POINT ( 'NONE',  ( 81.59615242270662350, -34.63259618943234130, -96.99999999999997158 ) ) ;
#6076=CARTESIAN_POINT ( 'NONE',  ( -82.39999999999999147, -33.48750000000000426, 103.0000000000000000 ) ) ;
#6077=CARTESIAN_POINT ( 'NONE',  ( -80.03686793005711309, -35.00000000000002842, -101.6462804658012118 ) ) ;
#6081=CARTESIAN_POINT ( 'NONE',  ( -79.64356964375001269, -33.02812499938548285, -101.5914258081833879 ) ) ;
#6084=CARTESIAN_POINT ( 'NONE',  ( -85.40000000000000568, -32.68124999877097281, 98.26794919243111792 ) ) ;
#6086=CARTESIAN_POINT ( 'NONE',  ( 82.40000000000001990, -33.26250000000000284, -97.00000000000000000 ) ) ;
#6092=CARTESIAN_POINT ( 'NONE',  ( -85.40000000000000568, -32.64374999877097139, 99.99999999999998579 ) ) ;
#6093=CARTESIAN_POINT ( 'NONE',  ( 83.90000000000000568, -31.72500000000000142, 97.40192378864668399 ) ) ;
#6097=CARTESIAN_POINT ( 'NONE',  ( 83.30522522562139898, -31.99999999999999289, -97.33297554272277807 ) ) ;
#6099=CARTESIAN_POINT ( 'NONE',  ( 82.39999999999999147, -31.37812499938548427, -103.1828516163667899 ) ) ;
#6100=ORIENTED_EDGE ( 'NONE', *, *, #528, .F. ) ;
#6102=CARTESIAN_POINT ( 'NONE',  ( 82.39999999999999147, -33.17812499938548854, -103.1828516163667899 ) ) ;
#6104=FACE_OUTER_BOUND ( 'NONE', #2486, .T. ) ;
#6105=CARTESIAN_POINT ( 'NONE',  ( -82.40000000000000568, -34.78124999877096712, 102.9999999999999858 ) ) ;
#6107=CARTESIAN_POINT ( 'NONE',  ( -79.39999999999999147, -31.12500000000000355, 99.99999999999998579 ) ) ;
#6109=CARTESIAN_POINT ( 'NONE',  ( 79.68596062386927770, -32.00000000000000000, 98.72172371342817598 ) ) ;
#6112=CARTESIAN_POINT ( 'NONE',  ( 79.64356964375001269, -30.77812499938548285, 101.5914258081833879 ) ) ;
#6116=CARTESIAN_POINT ( 'NONE',  ( -81.59615242270662350, -32.56740381056766864, 103.0000000000000000 ) ) ;
#6117=CARTESIAN_POINT ( 'NONE',  ( 83.77821517812500929, -30.51562499938548711, 97.61286128772489690 ) ) ;
#6118=CARTESIAN_POINT ( 'NONE',  ( -85.40000000000000568, -32.66250000000000142, 101.7320508075688821 ) ) ;
#6120=CARTESIAN_POINT ( 'NONE',  ( 81.02178482187500208, -35.05312499938548854, -102.3871387122750889 ) ) ;
#6121=CARTESIAN_POINT ( 'NONE',  ( -85.15643035624999868, -31.19062499938548783, -101.5914258081833879 ) ) ;
#6123=ORIENTED_EDGE ( 'NONE', *, *, #528, .T. ) ;
#6124=CARTESIAN_POINT ( 'NONE',  ( 85.15643035624999868, -31.11562499938548854, 98.40857419181659793 ) ) ;
#6125=DIRECTION ( 'NONE',  ( -1.586032892321652088E-15, -1.000000000000000000, 0.000000000000000000 ) ) ;
#6128=CARTESIAN_POINT ( 'NONE',  ( -83.77821517812500929, -31.97812499938548925, 102.3871387122750889 ) ) ;
#6131=CARTESIAN_POINT ( 'NONE',  ( -82.39999999999999147, -32.13749999999999574, -96.53589838486223584 ) ) ;
#6135=CARTESIAN_POINT ( 'NONE',  ( -83.90000000000000568, -34.81874999877096855, -97.40192378864668399 ) ) ;
#6136=CARTESIAN_POINT ( 'NONE',  ( -82.39999999999999147, -32.39062499938548001, -96.81714838363319586 ) ) ;
#6141=CARTESIAN_POINT ( 'NONE',  ( -81.02178482187500208, -33.89062499938548711, -102.3871387122750889 ) ) ;
#6142=CARTESIAN_POINT ( 'NONE',  ( 82.39999999999999147, -32.95312499938548711, 103.1828516163667899 ) ) ;
#6145=CARTESIAN_POINT ( 'NONE',  ( 85.40000000000000568, -35.36739044046696279, -98.90809476984486537 ) ) ;
#6147=EDGE_CURVE ( 'NONE', #13275, #13349, #4903, .T. ) ;
#6148=ORIENTED_EDGE ( 'NONE', *, *, #18134, .F. ) ;
#6157=ORIENTED_EDGE ( 'NONE', *, *, #4155, .F. ) ;
#6158=ORIENTED_EDGE ( 'NONE', *, *, #14769, .F. ) ;
#6162=CARTESIAN_POINT ( 'NONE',  ( -83.90000000000000568, -33.97500000000000853, -97.40192378864668399 ) ) ;
#6167=CARTESIAN_POINT ( 'NONE',  ( -81.02178482187500208, -33.55312499938548854, 97.61286128772489690 ) ) ;
#6170=VECTOR ( 'NONE', #6125, 1000.000000000000000 ) ;
#6173=DIRECTION ( 'NONE',  ( 0.000000000000000000, -0.000000000000000000, -1.000000000000000000 ) ) ;
#6174=CARTESIAN_POINT ( 'NONE',  ( -80.32125193361316917, -35.00000000000001421, -102.0234471769925193 ) ) ;
#6177=VECTOR ( 'NONE', #16045, 1000.000000000000000 ) ;
#6178=CARTESIAN_POINT ( 'NONE',  ( -83.77821517812500929, -34.11562499938548854, -97.61286128772489690 ) ) ;
#6181=CARTESIAN_POINT ( 'NONE',  ( 94.79999999999995453, -35.00000000000000000, -150.0000000000000000 ) ) ;
#6182=LINE ( 'NONE', #7536, #3039 ) ;
#6184=DIRECTION ( 'NONE',  ( 1.000000000000000000, 0.000000000000000000, 0.000000000000000000 ) ) ;
#6185=AXIS2_PLACEMENT_3D ( 'NONE', #8542, #14399, #9726 ) ;
#6189=CARTESIAN_POINT ( 'NONE',  ( 82.40000000000000568, -34.55624999877097281, 102.9999999999999858 ) ) ;
#6191=CARTESIAN_POINT ( 'NONE',  ( -82.39999999999999147, -31.63124999877097210, 103.4641016151377499 ) ) ;
#6192=CARTESIAN_POINT ( 'NONE',  ( 82.39999999999999147, -31.68750000000000355, 96.53589838486223584 ) ) ;
#6194=EDGE_CURVE ( 'NONE', #2988, #17308, #10333, .T. ) ;
#6195=CARTESIAN_POINT ( 'NONE',  ( 82.40000000000001990, -32.30624999877097281, 103.0000000000000000 ) ) ;
#6197=CARTESIAN_POINT ( 'NONE',  ( 79.64356964374998427, -33.14062499938548711, -98.40857419181659793 ) ) ;
#6198=VECTOR ( 'NONE', #9742, 1000.000000000000000 ) ;
#6199=CARTESIAN_POINT ( 'NONE',  ( -79.68596062386970402, -32.00000000000002132, -98.72172371342720965 ) ) ;
#6201=CARTESIAN_POINT ( 'NONE',  ( 79.64356964374999848, -34.86562499938548143, -99.99999999999998579 ) ) ;
#6205=CARTESIAN_POINT ( 'NONE',  ( 83.77821517812500929, -32.76562499938548711, -102.3871387122750889 ) ) ;
#6209=CARTESIAN_POINT ( 'NONE',  ( -82.39999999999999147, -34.75312499938549138, 96.81714838363319586 ) ) ;
#6214=CARTESIAN_POINT ( 'NONE',  ( 85.15643035624999868, -31.07812499938548356, 101.5914258081833879 ) ) ;
#6216=CARTESIAN_POINT ( 'NONE',  ( -83.90000000000000568, -33.22500000000000142, -102.5980762113533018 ) ) ;
#6219=CARTESIAN_POINT ( 'NONE',  ( 85.15643035625001289, -33.85312499938549280, 99.99999999999998579 ) ) ;
#6222=CARTESIAN_POINT ( 'NONE',  ( -79.64356964374998427, -32.24062499938548854, 98.40857419181659793 ) ) ;
#6223=CARTESIAN_POINT ( 'NONE',  ( -83.77821517812500929, -34.67812499938548854, -97.61286128772489690 ) ) ;
#6225=CARTESIAN_POINT ( 'NONE',  ( 83.77821517812500929, -31.52812499938548996, 97.61286128772489690 ) ) ;
#6226=FACE_OUTER_BOUND ( 'NONE', #15808, .T. ) ;
#6228=CARTESIAN_POINT ( 'NONE',  ( -79.64356964375001269, -32.76562499938548711, 101.5914258081833879 ) ) ;
#6229=FACE_OUTER_BOUND ( 'NONE', #18073, .T. ) ;
#6231=CARTESIAN_POINT ( 'NONE',  ( -82.39999999999999147, -31.01249999999999929, -103.4641016151377499 ) ) ;
#6232=CARTESIAN_POINT ( 'NONE',  ( 84.69814068649969840, -35.00052333152936512, -98.07164593887567605 ) ) ;
#6233=CARTESIAN_POINT ( 'NONE',  ( 79.39999999999999147, -33.76874999877097139, 99.99999999999998579 ) ) ;
#6234=CARTESIAN_POINT ( 'NONE',  ( -85.15643035624999868, -34.26562499938548711, -98.40857419181659793 ) ) ;
#6240=CARTESIAN_POINT ( 'NONE',  ( 83.90000000000000568, -32.17500000000000426, 97.40192378864668399 ) ) ;
#6241=CARTESIAN_POINT ( 'NONE',  ( 79.64356964374998427, -34.37812499938548427, 101.5914258081833879 ) ) ;
#6242=PLANE ( 'NONE',  #11177 ) ;
#6244=CARTESIAN_POINT ( 'NONE',  ( 80.90000000000000568, -35.19374999877096855, -102.5980762113533018 ) ) ;
#6247=EDGE_CURVE ( 'NONE', #12925, #10773, #1321, .T. ) ;
#6255=ORIENTED_EDGE ( 'NONE', *, *, #7076, .T. ) ;
#6258=CARTESIAN_POINT ( 'NONE',  ( -85.40000000000000568, -34.05000000000000426, -99.99999999999998579 ) ) ;
#6259=ORIENTED_EDGE ( 'NONE', *, *, #15450, .T. ) ;
#6260=ADVANCED_FACE ( 'NONE', ( #19196 ), #8771, .F. ) ;
#6261=DIRECTION ( 'NONE',  ( 1.000000000000000000, 0.000000000000000000, -0.000000000000000000 ) ) ;
#6263=EDGE_CURVE ( 'NONE', #19033, #10520, #13693, .T. ) ;
#6264=CARTESIAN_POINT ( 'NONE',  ( -69.99999999999998579, -32.00000000000000000, 150.0000000000000000 ) ) ;
#6274=ORIENTED_EDGE ( 'NONE', *, *, #17842, .T. ) ;
#6275=CARTESIAN_POINT ( 'NONE',  ( -81.02178482187500208, -32.09062499938548285, -102.3871387122750889 ) ) ;
#6277=( BOUNDED_CURVE ( )  B_SPLINE_CURVE ( 2, ( #6692, #12635, #18318, #14295, #5617, #2660, #4235, #11752, #11562 ),
 .UNSPECIFIED., .F., .F. ) 
 B_SPLINE_CURVE_WITH_KNOTS ( ( 3, 2, 2, 2, 3 ),
 ( 0.6875000000000000000, 0.6944444444444444198, 0.7083333333333333703, 0.7222222222222222099, 0.7291666666666668517 ),
 .UNSPECIFIED. ) 
 CURVE ( )  GEOMETRIC_REPRESENTATION_ITEM ( )  RATIONAL_B_SPLINE_CURVE ( ( 0.9330127018922194093, 0.9330127018922194093, 1.000000000000000000, 0.8660254037844387076, 1.000000000000000000, 0.8660254037844387076, 1.000000000000000000, 0.9330127018922177440, 0.9330127018922194093 ) ) 
 REPRESENTATION_ITEM ( '' )  );
#6280=CARTESIAN_POINT ( 'NONE',  ( -83.90000000000000568, -32.71874999877096712, 97.40192378864668399 ) ) ;
#6282=DIRECTION ( 'NONE',  ( 0.000000000000000000, -0.000000000000000000, -1.000000000000000000 ) ) ;
#6285=CARTESIAN_POINT ( 'NONE',  ( -84.29633955546275104, -32.00000000000001421, 102.0295751981970511 ) ) ;
#6286=CARTESIAN_POINT ( 'NONE',  ( 82.39999999999999147, -31.01249999999999929, -96.53589838486223584 ) ) ;
#6287=CARTESIAN_POINT ( 'NONE',  ( -80.90000000000000568, -31.89374999877096784, 97.40192378864668399 ) ) ;
#6288=CARTESIAN_POINT ( 'NONE',  ( 80.90000000000000568, -32.40000000000000568, 102.5980762113533018 ) ) ;
#6289=CARTESIAN_POINT ( 'NONE',  ( 83.20384757729335945, -33.63615380933863008, 102.9999999999999716 ) ) ;
#6291=CARTESIAN_POINT ( 'NONE',  ( 85.15643035625001289, -33.44062499938548427, -98.40857419181659793 ) ) ;
#6292=CARTESIAN_POINT ( 'NONE',  ( 79.58826230851033756, -31.99999999999998579, -98.95399275611669054 ) ) ;
#6293=CARTESIAN_POINT ( 'NONE',  ( 81.02178482187500208, -32.69062499938548427, -102.3871387122750889 ) ) ;
#6297=CARTESIAN_POINT ( 'NONE',  ( -85.40000000000000568, -34.50000000000000000, 99.99999999999998579 ) ) ;
#6298=CYLINDRICAL_SURFACE ( 'NONE', #17256, 3.000000000000002665 ) ;
#6300=EDGE_CURVE ( 'NONE', #9376, #2579, #18148, .T. ) ;
#6302=CARTESIAN_POINT ( 'NONE',  ( -83.90000000000000568, -30.52500000000000213, 97.40192378864668399 ) ) ;
#6308=CARTESIAN_POINT ( 'NONE',  ( 84.67508262029679145, -31.99999999999999289, -101.5663513044664938 ) ) ;
#6311=CARTESIAN_POINT ( 'NONE',  ( 79.64356964375001269, -34.94062499938549138, 101.5914258081833879 ) ) ;
#6313=CARTESIAN_POINT ( 'NONE',  ( 82.39999999999999147, -32.61562499938548854, -96.81714838363319586 ) ) ;
#6315=CARTESIAN_POINT ( 'NONE',  ( -85.15643035625001289, -33.85312499938549280, 99.99999999999998579 ) ) ;
#6316=CARTESIAN_POINT ( 'NONE',  ( -79.64356964375001269, -34.11562499938548854, -98.40857419181659793 ) ) ;
#6317=PRODUCT_DEFINITION_CONTEXT ( 'detailed design', #14194, 'design' ) ;
#6319=CARTESIAN_POINT ( 'NONE',  ( 79.64356964374999848, -30.47812499938548569, 99.99999999999998579 ) ) ;
#6324=CARTESIAN_POINT ( 'NONE',  ( -79.64356964374999848, -34.52812499938548285, 99.99999999999998579 ) ) ;
#6325=CARTESIAN_POINT ( 'NONE',  ( -84.44763168836720979, -32.00000000000001421, -98.15470523285542015 ) ) ;
#6326=ORIENTED_EDGE ( 'NONE', *, *, #8155, .T. ) ;
#6327=CARTESIAN_POINT ( 'NONE',  ( -80.90000000000000568, -31.20000000000000284, -97.40192378864668399 ) ) ;
#6329=CARTESIAN_POINT ( 'NONE',  ( 85.40000000000000568, -34.85624999877096997, -101.7320508075688821 ) ) ;
#6330=DIRECTION ( 'NONE',  ( 0.000000000000000000, 1.000000000000000000, 0.000000000000000000 ) ) ;
#6336=CARTESIAN_POINT ( 'NONE',  ( 82.39999999999999147, -32.36250000000000426, 102.9999999999999858 ) ) ;
#6337=CARTESIAN_POINT ( 'NONE',  ( 81.02178482187500208, -33.14062499938548711, 97.61286128772489690 ) ) ;
#6340=CARTESIAN_POINT ( 'NONE',  ( 82.39999999999999147, -32.81250000000000000, -97.00000000000000000 ) ) ;
#6341=CARTESIAN_POINT ( 'NONE',  ( 80.90000000000000568, -33.39374999877097139, -102.5980762113533018 ) ) ;
#6351=CARTESIAN_POINT ( 'NONE',  ( -83.20384757729337366, -32.15759618943233278, -97.00000000000000000 ) ) ;
#6352=ORIENTED_EDGE ( 'NONE', *, *, #17037, .F. ) ;
#6355=CARTESIAN_POINT ( 'NONE',  ( -85.40000000000000568, -32.68124999877097281, -101.7320508075688679 ) ) ;
#6361=CARTESIAN_POINT ( 'NONE',  ( 79.39999999999999147, -34.76250000000000284, -101.7320508075688537 ) ) ;
#6362=CARTESIAN_POINT ( 'NONE',  ( -79.39999999999999147, -33.33749999999999858, 98.26794919243110371 ) ) ;
#6367=CARTESIAN_POINT ( 'NONE',  ( -81.02178482187500208, -33.89062499938548711, -102.3871387122750889 ) ) ;
#6368=CARTESIAN_POINT ( 'NONE',  ( -82.40000000000001990, -32.75624999877096855, -103.0000000000000000 ) ) ;
#6371=CARTESIAN_POINT ( 'NONE',  ( 82.40000000000000568, -30.00000000000000355, -99.99999999999998579 ) ) ;
#6372=CARTESIAN_POINT ( 'NONE',  ( 69.99999999999998579, -31.99999999999998579, -150.0000000000000000 ) ) ;
#6374=DIRECTION ( 'NONE',  ( 0.000000000000000000, 0.000000000000000000, -1.000000000000000000 ) ) ;
#6375=CARTESIAN_POINT ( 'NONE',  ( -82.40000000000001990, -32.13750000000000284, 103.0000000000000000 ) ) ;
#6378=CARTESIAN_POINT ( 'NONE',  ( 79.39999999999999147, -31.08750000000000213, -98.26794919243110371 ) ) ;
#6379=ADVANCED_FACE ( 'NONE', ( #5774 ), #10272, .F. ) ;
#6380=CARTESIAN_POINT ( 'NONE',  ( -85.40000000000000568, -34.40624999877096712, 101.7320508075688679 ) ) ;
#6381=CARTESIAN_POINT ( 'NONE',  ( -85.40000000000000568, -32.23124999877096997, -101.7320508075688821 ) ) ;
#6383=CARTESIAN_POINT ( 'NONE',  ( 81.02178482187500208, -33.10312499938548569, -97.61286128772489690 ) ) ;
#6384=CARTESIAN_POINT ( 'NONE',  ( 83.52022063337599889, -31.99999999999998579, -97.42682425339255303 ) ) ;
#6385=CARTESIAN_POINT ( 'NONE',  ( 85.15643035624999868, -34.67812499938548143, -98.40857419181659793 ) ) ;
#6386=ORIENTED_EDGE ( 'NONE', *, *, #16158, .F. ) ;
#6389=CARTESIAN_POINT ( 'NONE',  ( -82.39999999999999147, -34.38750000000000284, 103.4641016151377499 ) ) ;
#6396=CARTESIAN_POINT ( 'NONE',  ( -80.90000000000000568, -31.65000000000000568, 102.5980762113533018 ) ) ;
#6404=CARTESIAN_POINT ( 'NONE',  ( -79.64356964374998427, -32.24062499938548854, -101.5914258081833879 ) ) ;
#6405=CARTESIAN_POINT ( 'NONE',  ( 83.77821517812500929, -34.67812499938548854, 97.61286128772489690 ) ) ;
#6406=CARTESIAN_POINT ( 'NONE',  ( 85.15643035624999868, -31.11562499938548854, -101.5914258081833879 ) ) ;
#6408=CARTESIAN_POINT ( 'NONE',  ( -82.39999999999999147, -34.19062499938548427, 103.1828516163667899 ) ) ;
#6409=CARTESIAN_POINT ( 'NONE',  ( -79.64356964375001269, -33.66562499938549280, -98.40857419181659793 ) ) ;
#6410=EDGE_LOOP ( 'NONE', ( #10331, #14644, #14692, #18934 ) ) ;
#6411=CARTESIAN_POINT ( 'NONE',  ( 81.02178482187500208, -33.25312499938548427, 97.61286128772489690 ) ) ;
#6414=CARTESIAN_POINT ( 'NONE',  ( -82.39999999999999147, -33.96562499938548285, 96.81714838363319586 ) ) ;
#6418=CARTESIAN_POINT ( 'NONE',  ( -85.40000000000000568, -30.48749999999999716, -101.7320508075688679 ) ) ;
#6419=CARTESIAN_POINT ( 'NONE',  ( 82.39999999999999147, -34.83749999999999858, -103.4641016151377499 ) ) ;
#6420=CARTESIAN_POINT ( 'NONE',  ( 80.90000000000000568, -33.84374999877096712, 97.40192378864668399 ) ) ;
#6421=CARTESIAN_POINT ( 'NONE',  ( -96.99999999999998579, -5.200000000000000178, -150.0000000000000000 ) ) ;
#6426=ADVANCED_FACE ( 'NONE', ( #15602 ), #16872, .F. ) ;
#6429=CARTESIAN_POINT ( 'NONE',  ( 82.40000000000000568, -34.61250000000001137, -97.00000000000000000 ) ) ;
#6430=CARTESIAN_POINT ( 'NONE',  ( -83.90000000000000568, -33.61874999877097281, -102.5980762113533018 ) ) ;
#6431=CYLINDRICAL_SURFACE ( 'NONE', #16178, 5.199999999999996625 ) ;
#6432=VECTOR ( 'NONE', #163, 1000.000000000000000 ) ;
#6434=CARTESIAN_POINT ( 'NONE',  ( 79.64356964375001269, -32.31562499938548427, -101.5914258081833879 ) ) ;
#6435=CARTESIAN_POINT ( 'NONE',  ( 79.39999999999999147, -34.76250000000000284, 98.26794919243113213 ) ) ;
#6444=ORIENTED_EDGE ( 'NONE', *, *, #6194, .F. ) ;
#6448=CARTESIAN_POINT ( 'NONE',  ( -85.40000000000000568, -33.60000000000000142, -99.99999999999998579 ) ) ;
#6451=CARTESIAN_POINT ( 'NONE',  ( -79.39999999999999147, -34.66874999877096997, -99.99999999999998579 ) ) ;
#6457=DIRECTION ( 'NONE',  ( 0.000000000000000000, -0.000000000000000000, -1.000000000000000000 ) ) ;
#6459=ORIENTED_EDGE ( 'NONE', *, *, #7602, .F. ) ;
#6463=CARTESIAN_POINT ( 'NONE',  ( -79.39999999999999147, -33.37500000000000000, -99.99999999999998579 ) ) ;
#6467=ORIENTED_EDGE ( 'NONE', *, *, #9613, .F. ) ;
#6472=CARTESIAN_POINT ( 'NONE',  ( 81.59615242270662350, -33.22634618820330843, -97.00000000000000000 ) ) ;
#6473=CARTESIAN_POINT ( 'NONE',  ( 85.15643035625001289, -35.09062499938548285, -99.99999999999998579 ) ) ;
#6476=CARTESIAN_POINT ( 'NONE',  ( -79.39999999999999147, -33.35624999877097707, 101.7320508075688537 ) ) ;
#6477=CARTESIAN_POINT ( 'NONE',  ( -82.40000000000000568, -32.30624999877097281, -102.9999999999999858 ) ) ;
#6479=CARTESIAN_POINT ( 'NONE',  ( 79.64356964374998427, -34.04062499938549280, -98.40857419181659793 ) ) ;
#6480=AXIS2_PLACEMENT_3D ( 'NONE', #16628, #2854, #10571 ) ;
#6482=CARTESIAN_POINT ( 'NONE',  ( -81.02178482187500208, -33.89062499938548711, 97.61286128772489690 ) ) ;
#6483=CARTESIAN_POINT ( 'NONE',  ( 82.39999999999999147, -33.17812499938548854, -103.1828516163667899 ) ) ;
#6486=CARTESIAN_POINT ( 'NONE',  ( -85.40000000000000568, -33.60000000000000142, 99.99999999999998579 ) ) ;
#6487=AXIS2_PLACEMENT_3D ( 'NONE', #2891, #12167, #8847 ) ;
#6494=CARTESIAN_POINT ( 'NONE',  ( -83.90000000000000568, -33.22500000000000142, 97.40192378864668399 ) ) ;
#6496=CARTESIAN_POINT ( 'NONE',  ( -84.70388354820684640, -35.00002705695768412, 98.07851859032987818 ) ) ;
#6497=AXIS2_PLACEMENT_3D ( 'NONE', #3718, #7922, #8015 ) ;
#6499=CARTESIAN_POINT ( 'NONE',  ( 81.02178482187500208, -32.99062499938548854, 102.3871387122750889 ) ) ;
#6501=AXIS2_PLACEMENT_3D ( 'NONE', #10295, #14387, #13118 ) ;
#6502=EDGE_CURVE ( 'NONE', #11363, #9425, #18731, .T. ) ;
#6503=CARTESIAN_POINT ( 'NONE',  ( 79.58826230851033756, -31.99999999999998579, -98.95399275611669054 ) ) ;
#6506=CARTESIAN_POINT ( 'NONE',  ( -85.15643035625001289, -32.46562499938548996, -98.40857419181659793 ) ) ;
#6507=CARTESIAN_POINT ( 'NONE',  ( 79.64356964374999848, -34.52812499938548285, 99.99999999999998579 ) ) ;
#6508=CARTESIAN_POINT ( 'NONE',  ( 85.15643035624999868, -31.56562499938548427, -101.5914258081833879 ) ) ;
#6511=CARTESIAN_POINT ( 'NONE',  ( -82.39999999999999147, -34.64062499938548711, 103.1828516163667899 ) ) ;
#6512=CARTESIAN_POINT ( 'NONE',  ( -82.39999999999999147, -33.51562499938548001, -103.1828516163667899 ) ) ;
#6513=ORIENTED_EDGE ( 'NONE', *, *, #11389, .T. ) ;
#6514=CARTESIAN_POINT ( 'NONE',  ( 82.39999999999999147, -32.16562499938549280, 103.1828516163667899 ) ) ;
#6516=AXIS2_PLACEMENT_3D ( 'NONE', #10366, #11548, #14757 ) ;
#6517=DIRECTION ( 'NONE',  ( -1.000000000000000000, 1.156482317317870344E-15, 0.000000000000000000 ) ) ;
#6518=CARTESIAN_POINT ( 'NONE',  ( -82.39999999999999147, -34.41562499938547859, 96.81714838363319586 ) ) ;
#6520=ORIENTED_EDGE ( 'NONE', *, *, #8170, .T. ) ;
#6521=CARTESIAN_POINT ( 'NONE',  ( -79.39999999999999147, -32.92500000000000426, -99.99999999999998579 ) ) ;
#6524=CARTESIAN_POINT ( 'NONE',  ( -85.15643035624999868, -35.16562499938547859, -98.40857419181659793 ) ) ;
#6528=CARTESIAN_POINT ( 'NONE',  ( -82.40000000000000568, -30.00000000000000355, 99.99999999999998579 ) ) ;
#6531=CARTESIAN_POINT ( 'NONE',  ( 82.40000000000001990, -34.16250000000000853, 103.0000000000000000 ) ) ;
#6533=CARTESIAN_POINT ( 'NONE',  ( 82.39999999999999147, -31.71562499938548640, -96.81714838363319586 ) ) ;
#6540=CARTESIAN_POINT ( 'NONE',  ( -85.40000000000000568, -34.95000000000000284, 99.99999999999998579 ) ) ;
#6541=EDGE_LOOP ( 'NONE', ( #3759, #5628, #1847, #4935 ) ) ;
#6543=VERTEX_POINT ( 'NONE', #12467 ) ;
#6544=CARTESIAN_POINT ( 'NONE',  ( -85.15643035625001289, -30.59062499938548285, -99.99999999999998579 ) ) ;
#6545=DIRECTION ( 'NONE',  ( -0.000000000000000000, 0.000000000000000000, -1.000000000000000000 ) ) ;
#6546=CARTESIAN_POINT ( 'NONE',  ( -94.79999999999999716, -5.200000000000000178, 150.0000000000000000 ) ) ;
#6547=ORIENTED_EDGE ( 'NONE', *, *, #13345, .T. ) ;
#6549=CARTESIAN_POINT ( 'NONE',  ( -85.40000000000000568, -33.05624999877096570, -98.26794919243111792 ) ) ;
#6552=( BOUNDED_CURVE ( )  B_SPLINE_CURVE ( 2, ( #3432, #7923, #4617, #13873, #14968, #16537, #1682, #13497, #6086 ),
 .UNSPECIFIED., .F., .F. ) 
 B_SPLINE_CURVE_WITH_KNOTS ( ( 3, 2, 2, 2, 3 ),
 ( 0.5625000000000000000, 0.5694444444444444198, 0.5833333333333333703, 0.5972222222222222099, 0.6041666666666666297 ),
 .UNSPECIFIED. ) 
 CURVE ( )  GEOMETRIC_REPRESENTATION_ITEM ( )  RATIONAL_B_SPLINE_CURVE ( ( 0.9330127018922194093, 0.9330127018922194093, 1.000000000000000000, 0.8660254037844387076, 1.000000000000000000, 0.8660254037844387076, 1.000000000000000000, 0.9330127018922198534, 0.9330127018922192983 ) ) 
 REPRESENTATION_ITEM ( '' )  );
#6555=CARTESIAN_POINT ( 'NONE',  ( 82.39999999999999147, -34.33124999877097139, -103.0000000000000000 ) ) ;
#6559=CARTESIAN_POINT ( 'NONE',  ( -83.77821517812500929, -34.56562499938548427, -97.61286128772489690 ) ) ;
#6560=CARTESIAN_POINT ( 'NONE',  ( -79.39999999999999147, -32.90624999877096712, -98.26794919243113213 ) ) ;
#6561=ORIENTED_EDGE ( 'NONE', *, *, #9238, .T. ) ;
#6570=CARTESIAN_POINT ( 'NONE',  ( 85.15643035624999868, -34.67812499938548143, -98.40857419181659793 ) ) ;
#6572=CARTESIAN_POINT ( 'NONE',  ( -85.15643035624999868, -30.29062499938548925, 98.40857419181659793 ) ) ;
#6574=CARTESIAN_POINT ( 'NONE',  ( 85.40000000000000568, -32.28750000000000142, -98.26794919243111792 ) ) ;
#6576=CARTESIAN_POINT ( 'NONE',  ( 85.15643035625001289, -34.26562499938548711, -101.5914258081833879 ) ) ;
#6578=CARTESIAN_POINT ( 'NONE',  ( -85.15643035625001289, -33.74062499938548854, 99.99999999999998579 ) ) ;
#6579=EDGE_CURVE ( 'NONE', #540, #2299, #17624, .T. ) ;
#6581=CARTESIAN_POINT ( 'NONE',  ( 79.64356964375001269, -33.55312499938548854, -101.5914258081833879 ) ) ;
#6583=CARTESIAN_POINT ( 'NONE',  ( 82.40000000000000568, -33.03750000000000142, 96.99999999999998579 ) ) ;
#6584=CARTESIAN_POINT ( 'NONE',  ( -83.90000000000000568, -33.67500000000000426, 97.40192378864668399 ) ) ;
#6585=CARTESIAN_POINT ( 'NONE',  ( 85.40000000000000568, -33.50624999877096855, -101.7320508075688821 ) ) ;
#6589=CARTESIAN_POINT ( 'NONE',  ( -79.39999999999999147, -32.51250000000000284, 101.7320508075688537 ) ) ;
#6594=CARTESIAN_POINT ( 'NONE',  ( 82.39999999999999147, -31.37812499938548427, 96.81714838363319586 ) ) ;
#6595=CARTESIAN_POINT ( 'NONE',  ( 84.93334430221544551, -31.99999999999998579, -101.1009827666102581 ) ) ;
#6597=CARTESIAN_POINT ( 'NONE',  ( -85.15643035625001289, -32.54062499938548569, -101.5914258081833879 ) ) ;
#6598=CARTESIAN_POINT ( 'NONE',  ( 83.77821517812500929, -33.36562499938548854, 102.3871387122750889 ) ) ;
#6599=CARTESIAN_POINT ( 'NONE',  ( 81.02178482187500208, -32.20312499938548711, -97.61286128772489690 ) ) ;
#6601=CARTESIAN_POINT ( 'NONE',  ( -81.02178482187500208, -34.90312499938548285, 97.61286128772489690 ) ) ;
#6602=CARTESIAN_POINT ( 'NONE',  ( -82.39999999999999147, -33.06562499938548427, -103.1828516163667899 ) ) ;
#6604=CARTESIAN_POINT ( 'NONE',  ( 82.39999999999999147, -33.29062499938549280, 96.81714838363319586 ) ) ;
#6606=CARTESIAN_POINT ( 'NONE',  ( -79.64356964374999848, -30.81562499938548427, 99.99999999999998579 ) ) ;
#6607=CARTESIAN_POINT ( 'NONE',  ( -82.39999999999999147, -34.86562499938548854, 96.81714838363319586 ) ) ;
#6611=CARTESIAN_POINT ( 'NONE',  ( -85.40000000000000568, -34.08749999999999858, -101.7320508075688679 ) ) ;
#6613=CARTESIAN_POINT ( 'NONE',  ( 79.39999999999999147, -32.92500000000000426, -99.99999999999998579 ) ) ;
#6614=CARTESIAN_POINT ( 'NONE',  ( 83.60689295392862164, -35.00000000000000000, -97.24646917567282856 ) ) ;
#6619=ORIENTED_EDGE ( 'NONE', *, *, #16104, .T. ) ;
#6621=CARTESIAN_POINT ( 'NONE',  ( 83.90000000000000568, -34.42500000000000426, -102.5980762113533018 ) ) ;
#6622=CARTESIAN_POINT ( 'NONE',  ( -83.20384757729335945, -33.45134618820330985, -96.99999999999998579 ) ) ;
#6623=DIRECTION ( 'NONE',  ( -1.000000000000000000, 0.000000000000000000, 0.000000000000000000 ) ) ;
#6624=CARTESIAN_POINT ( 'NONE',  ( -82.40000000000000568, -34.55624999877097281, 97.00000000000000000 ) ) ;
#6625=CARTESIAN_POINT ( 'NONE',  ( 79.64356964374999848, -30.47812499938548569, -99.99999999999998579 ) ) ;
#6626=CARTESIAN_POINT ( 'NONE',  ( 81.59615242270665192, -34.81740381056767575, 97.00000000000000000 ) ) ;
#6627=AXIS2_PLACEMENT_3D ( 'NONE', #10047, #12784, #1063 ) ;
#6629=ORIENTED_EDGE ( 'NONE', *, *, #12126, .F. ) ;
#6630=CARTESIAN_POINT ( 'NONE',  ( 83.90000000000000568, -31.66874999877096997, 97.40192378864668399 ) ) ;
#6638=VERTEX_POINT ( 'NONE', #10024 ) ;
#6639=CARTESIAN_POINT ( 'NONE',  ( -81.02178482187500208, -31.64062499938548356, -102.3871387122750889 ) ) ;
#6641=CARTESIAN_POINT ( 'NONE',  ( -83.90000000000000568, -32.17500000000000426, -97.40192378864668399 ) ) ;
#6643=CARTESIAN_POINT ( 'NONE',  ( 85.15643035625001289, -32.50312499938548427, 99.99999999999998579 ) ) ;
#6644=CARTESIAN_POINT ( 'NONE',  ( -85.40000000000000568, -34.44374999877096855, -99.99999999999998579 ) ) ;
#6646=CARTESIAN_POINT ( 'NONE',  ( 82.39999999999999147, -34.38750000000000284, 96.53589838486223584 ) ) ;
#6651=FACE_OUTER_BOUND ( 'NONE', #2111, .T. ) ;
#6652=CARTESIAN_POINT ( 'NONE',  ( 79.39999999999999147, -34.21874999877096712, -99.99999999999998579 ) ) ;
#6654=CARTESIAN_POINT ( 'NONE',  ( 85.40000000000000568, -30.39374999877097139, -99.99999999999998579 ) ) ;
#6657=CARTESIAN_POINT ( 'NONE',  ( 79.64356964374998427, -33.55312499938548854, -101.5914258081833879 ) ) ;
#6658=CARTESIAN_POINT ( 'NONE',  ( -85.15643035625001289, -35.09062499938548285, -99.99999999999998579 ) ) ;
#6665=ORIENTED_EDGE ( 'NONE', *, *, #3294, .T. ) ;
#6671=CARTESIAN_POINT ( 'NONE',  ( 85.40000000000000568, -30.41249999999999787, -101.7320508075688679 ) ) ;
#6672=EDGE_CURVE ( 'NONE', #18169, #13093, #4268, .T. ) ;
#6673=CARTESIAN_POINT ( 'NONE',  ( -79.64356964374999848, -34.98839802032724577, -99.56403331587389971 ) ) ;
#6674=B_SPLINE_CURVE_WITH_KNOTS ( 'NONE', 3,
 ( #4232, #2764, #10382, #7450, #15065, #13409, #2954, #11941, #18826, #5448, #14870, #11386, #4331, #8720, #14673, #39 ),
 .UNSPECIFIED., .F., .F.,
 ( 4, 2, 2, 2, 2, 2, 2, 4 ),
 ( 0.000000000000000000, 0.0005391024520904326520, 0.001078204904180865304, 0.002156409808361677265, 0.002695512260452082812, 0.003234614712542487492, 0.003773717164632892172, 0.004312819616723297285 ),
 .UNSPECIFIED. ) ;
#6675=CARTESIAN_POINT ( 'NONE',  ( -82.39999999999999147, -34.33124999877097139, 103.4641016151377499 ) ) ;
#6679=DIRECTION ( 'NONE',  ( 0.000000000000000000, 0.000000000000000000, 1.000000000000000000 ) ) ;
#6680=CARTESIAN_POINT ( 'NONE',  ( -82.39999999999999147, -33.85312499938547859, 96.81714838363319586 ) ) ;
#6684=CARTESIAN_POINT ( 'NONE',  ( -85.40000000000000568, -34.05000000000000426, 99.99999999999998579 ) ) ;
#6686=CARTESIAN_POINT ( 'NONE',  ( 83.20384757729335945, -33.69240381056766154, 102.9999999999999858 ) ) ;
#6689=CARTESIAN_POINT ( 'NONE',  ( -79.39999999999999147, -32.92500000000000426, 99.99999999999998579 ) ) ;
#6692=CARTESIAN_POINT ( 'NONE',  ( -82.40000000000000568, -33.71249999999998437, -102.9999999999999858 ) ) ;
#6693=CARTESIAN_POINT ( 'NONE',  ( 83.77821517812500929, -32.01562499938548001, 102.3871387122750889 ) ) ;
#6694=CARTESIAN_POINT ( 'NONE',  ( 84.82992844608112648, -31.99999999999999289, -98.68659295968670619 ) ) ;
#6695=( BOUNDED_CURVE ( )  B_SPLINE_CURVE ( 2, ( #1638, #16873, #7878, #6329, #16585, #12085, #10619, #4670, #9147 ),
 .UNSPECIFIED., .F., .F. ) 
 B_SPLINE_CURVE_WITH_KNOTS ( ( 3, 2, 2, 2, 3 ),
 ( 0.8125000000000001110, 0.8194444444444444198, 0.8333333333333333703, 0.8472222222222222099, 0.8530683953269213582 ),
 .UNSPECIFIED. ) 
 CURVE ( )  GEOMETRIC_REPRESENTATION_ITEM ( )  RATIONAL_B_SPLINE_CURVE ( ( 0.9330127018922194093, 0.9330127018922204085, 1.000000000000000000, 0.8660254037844387076, 1.000000000000000000, 0.8660254037844387076, 1.000000000000000000, 0.9436068149601996025, 0.9346881722405915305 ) ) 
 REPRESENTATION_ITEM ( '' )  );
#6698=CARTESIAN_POINT ( 'NONE',  ( 81.02178482187500208, -31.34062499938548996, 97.61286128772489690 ) ) ;
#6699=CARTESIAN_POINT ( 'NONE',  ( 79.64356964375001269, -32.31562499938548427, -101.5914258081833879 ) ) ;
#6701=CARTESIAN_POINT ( 'NONE',  ( -79.64356964374998427, -34.49062499938548854, 98.40857419181659793 ) ) ;
#6702=CARTESIAN_POINT ( 'NONE',  ( -85.15643035625001289, -31.49062499938548498, -99.99999999999998579 ) ) ;
#6703=EDGE_LOOP ( 'NONE', ( #7340, #16297, #6274, #7420 ) ) ;
#6704=CARTESIAN_POINT ( 'NONE',  ( 85.15643035625001289, -32.05312499938548854, 99.99999999999998579 ) ) ;
#6706=CARTESIAN_POINT ( 'NONE',  ( -85.15643035625001289, -30.59062499938548285, 99.99999999999998579 ) ) ;
#6707=CARTESIAN_POINT ( 'NONE',  ( -81.02178482187500208, -34.90312499938548285, 97.61286128772489690 ) ) ;
#6710=CARTESIAN_POINT ( 'NONE',  ( -80.90000000000000568, -32.40000000000000568, -102.5980762113533018 ) ) ;
#6718=CARTESIAN_POINT ( 'NONE',  ( 82.39999999999999147, -34.75312499938548427, 103.1828516163667899 ) ) ;
#6719=CARTESIAN_POINT ( 'NONE',  ( 85.15643035625001289, -31.15312499938548996, 99.99999999999998579 ) ) ;
#6722=CARTESIAN_POINT ( 'NONE',  ( 83.77821517812500929, -31.97812499938548925, -102.3871387122750889 ) ) ;
#6731=EDGE_CURVE ( 'NONE', #7323, #10655, #17641, .T. ) ;
#6733=DIRECTION ( 'NONE',  ( -0.000000000000000000, -1.000000000000000000, -0.000000000000000000 ) ) ;
#6736=CARTESIAN_POINT ( 'NONE',  ( -85.15643035624999868, -32.42812499938548854, -101.5914258081833879 ) ) ;
#6739=CARTESIAN_POINT ( 'NONE',  ( 83.77821517812500929, -33.77812499938548285, 97.61286128772489690 ) ) ;
#6740=CARTESIAN_POINT ( 'NONE',  ( -82.39999999999999147, -34.55624999877096570, -103.4641016151377499 ) ) ;
#6741=DIRECTION ( 'NONE',  ( 0.000000000000000000, 0.000000000000000000, 1.000000000000000000 ) ) ;
#6742=CARTESIAN_POINT ( 'NONE',  ( -80.03686793005704203, -35.00000000000000000, 98.35371953419887348 ) ) ;
#6747=B_SPLINE_CURVE_WITH_KNOTS ( 'NONE', 3,
 ( #7626, #17799, #13291, #16332, #11833, #10653, #13580, #11927, #6174, #6077, #2941, #16527, #14957, #16620, #4410, #3128, #10367, #7529 ),
 .UNSPECIFIED., .F., .F.,
 ( 4, 2, 2, 2, 2, 2, 2, 2, 4 ),
 ( 0.000000000000000000, 0.0007106627595358627324, 0.001421325519071725465, 0.002131988278607587980, 0.002842651038143450930, 0.003553313797679313879, 0.004263976557215175961, 0.004974639316751038910, 0.005685302076286901860 ),
 .UNSPECIFIED. ) ;
#6753=VERTEX_POINT ( 'NONE', #12446 ) ;
#6754=CARTESIAN_POINT ( 'NONE',  ( 79.64356964374998427, -33.47812499938547859, -98.40857419181659793 ) ) ;
#6757=DIRECTION ( 'NONE',  ( 0.000000000000000000, -1.000000000000000000, 0.000000000000000000 ) ) ;
#6758=ORIENTED_EDGE ( 'NONE', *, *, #4863, .T. ) ;
#6768=CARTESIAN_POINT ( 'NONE',  ( 79.39999999999999147, -33.86250000000000426, -101.7320508075688537 ) ) ;
#6771=CARTESIAN_POINT ( 'NONE',  ( -82.39999999999999147, -33.88124999877096855, 103.4641016151377499 ) ) ;
#6773=CARTESIAN_POINT ( 'NONE',  ( -82.39999999999999147, -33.20624999877097849, 97.00000000000000000 ) ) ;
#6774=CARTESIAN_POINT ( 'NONE',  ( 80.90000000000000568, -33.24374999877097281, 102.5980762113533018 ) ) ;
#6775=CARTESIAN_POINT ( 'NONE',  ( 82.40000000000001990, -33.88124999877096855, 97.00000000000000000 ) ) ;
#6776=DIRECTION ( 'NONE',  ( 0.000000000000000000, -1.000000000000000000, 0.000000000000000000 ) ) ;
#6777=CARTESIAN_POINT ( 'NONE',  ( -83.77821517812500929, -32.76562499938548711, 102.3871387122750889 ) ) ;
#6778=CYLINDRICAL_SURFACE ( 'NONE', #10522, 3.000000000000002665 ) ;
#6785=DIRECTION ( 'NONE',  ( -1.000000000000000000, 0.000000000000000000, 0.000000000000000000 ) ) ;
#6790=ORIENTED_EDGE ( 'NONE', *, *, #11964, .F. ) ;
#6795=CARTESIAN_POINT ( 'NONE',  ( 83.77821517812500929, -32.76562499938548711, 97.61286128772489690 ) ) ;
#6800=CARTESIAN_POINT ( 'NONE',  ( -79.64356964374998427, -34.11562499938548854, -98.40857419181659793 ) ) ;
#6801=CARTESIAN_POINT ( 'NONE',  ( 85.15643035624999868, -31.52812499938547930, 101.5914258081833879 ) ) ;
#6803=CARTESIAN_POINT ( 'NONE',  ( 85.15643035625001289, -34.30312499938548854, -99.99999999999998579 ) ) ;
#6805=CARTESIAN_POINT ( 'NONE',  ( -81.02178482187500208, -34.49062499938548854, 102.3871387122750889 ) ) ;
#6806=EDGE_LOOP ( 'NONE', ( #6942, #13539, #7564, #7804 ) ) ;
#6807=CARTESIAN_POINT ( 'NONE',  ( 85.15643035625001289, -31.60312499938548569, 99.99999999999998579 ) ) ;
#6808=VECTOR ( 'NONE', #7057, 1000.000000000000000 ) ;
#6810=CARTESIAN_POINT ( 'NONE',  ( -79.64356964375001269, -30.85312499938548569, 101.5914258081833879 ) ) ;
#6811=CARTESIAN_POINT ( 'NONE',  ( -79.64356964375001269, -31.67812499938548143, 98.40857419181659793 ) ) ;
#6812=CARTESIAN_POINT ( 'NONE',  ( -94.79999999999999716, -32.00000000000000000, 150.0000000000000000 ) ) ;
#6814=CARTESIAN_POINT ( 'NONE',  ( -85.40000000000000568, -34.50000000000000000, -99.99999999999998579 ) ) ;
#6818=CARTESIAN_POINT ( 'NONE',  ( -82.40000000000000568, -30.00000000000000355, 99.99999999999998579 ) ) ;
#6819=CARTESIAN_POINT ( 'NONE',  ( -83.20384757729338787, -34.59240381056766722, 97.00000000000000000 ) ) ;
#6820=VECTOR ( 'NONE', #7016, 1000.000000000000000 ) ;
#6821=CARTESIAN_POINT ( 'NONE',  ( -82.85024983566745505, -35.00000000000000711, 97.02690897175904183 ) ) ;
#6823=CARTESIAN_POINT ( 'NONE',  ( 81.02178482187500208, -34.94062499938548427, 97.61286128772489690 ) ) ;
#6824=CARTESIAN_POINT ( 'NONE',  ( 83.77821517812500929, -31.07812499938548711, 97.61286128772489690 ) ) ;
#6825=DIRECTION ( 'NONE',  ( 1.000000000000000000, 0.000000000000000000, 0.000000000000000000 ) ) ;
#6826=EDGE_CURVE ( 'NONE', #5168, #14858, #6277, .T. ) ;
#6827=CARTESIAN_POINT ( 'NONE',  ( -83.90000000000000568, -32.77499999999999858, -102.5980762113533018 ) ) ;
#6828=CARTESIAN_POINT ( 'NONE',  ( 79.64356964375001269, -31.79062499938548569, -98.40857419181659793 ) ) ;
#6839=CARTESIAN_POINT ( 'NONE',  ( -79.64356964375001269, -31.67812499938548143, -101.5914258081833879 ) ) ;
#6841=EDGE_LOOP ( 'NONE', ( #3699, #13865, #14193, #2144 ) ) ;
#6842=CARTESIAN_POINT ( 'NONE',  ( 79.64356964374998427, -34.49062499938548854, 101.5914258081833879 ) ) ;
#6843=CARTESIAN_POINT ( 'NONE',  ( -85.15643035624999868, -31.64062499938548356, -101.5914258081833879 ) ) ;
#6844=DIRECTION ( 'NONE',  ( 1.000000000000000000, 0.000000000000000000, -0.000000000000000000 ) ) ;
#6847=CARTESIAN_POINT ( 'NONE',  ( -81.02178482187500208, -33.59062499938548285, -97.61286128772489690 ) ) ;
#6853=CARTESIAN_POINT ( 'NONE',  ( 79.64356964374998427, -32.65312499938548285, -101.5914258081833879 ) ) ;
#6857=B_SPLINE_CURVE_WITH_KNOTS ( 'NONE', 3,
 ( #9044, #13725, #366, #15007, #15100, #2893, #1431, #10510, #3271, #9227, #1809, #9135, #268, #18048, #8941, #4458 ),
 .UNSPECIFIED., .F., .F.,
 ( 4, 2, 2, 2, 2, 2, 2, 4 ),
 ( 0.000000000000000000, 0.0005391024520904310257, 0.001078204904180862051, 0.002156409808361698516, 0.002695512260452095389, 0.003234614712542491395, 0.003773717164632888268, 0.004312819616723284274 ),
 .UNSPECIFIED. ) ;
#6858=CARTESIAN_POINT ( 'NONE',  ( -82.39999999999999147, -33.65624999877097423, 97.00000000000000000 ) ) ;
#6860=FACE_OUTER_BOUND ( 'NONE', #10242, .T. ) ;
#6864=EDGE_CURVE ( 'NONE', #9562, #2447, #3895, .T. ) ;
#6865=VERTEX_POINT ( 'NONE', #14675 ) ;
#6866=CARTESIAN_POINT ( 'NONE',  ( 79.39999999999999147, -32.92500000000000426, -99.99999999999998579 ) ) ;
#6867=FACE_OUTER_BOUND ( 'NONE', #6541, .T. ) ;
#6868=CARTESIAN_POINT ( 'NONE',  ( -79.64356964374999848, -30.47812499938548569, 99.99999999999998579 ) ) ;
#6873=CARTESIAN_POINT ( 'NONE',  ( 94.79999999999995453, -35.00000000000000000, 150.0000000000000000 ) ) ;
#6874=CARTESIAN_POINT ( 'NONE',  ( -84.51154815724953551, -35.14114861271051637, 98.22820072003833047 ) ) ;
#6875=LINE ( 'NONE', #12728, #5859 ) ;
#6879=CYLINDRICAL_SURFACE ( 'NONE', #4907, 3.000000000000002665 ) ;
#6886=CARTESIAN_POINT ( 'NONE',  ( -84.12112955302457351, -35.00000000000000000, -102.4658001909609908 ) ) ;
#6887=CARTESIAN_POINT ( 'NONE',  ( 85.15643035624999868, -32.35312499938549280, 98.40857419181659793 ) ) ;
#6891=CARTESIAN_POINT ( 'NONE',  ( -82.39999999999999147, -34.19062499938548427, -96.81714838363319586 ) ) ;
#6892=CARTESIAN_POINT ( 'NONE',  ( 81.02178482187500208, -32.24062499938548854, 97.61286128772489690 ) ) ;
#6893=CARTESIAN_POINT ( 'NONE',  ( 82.39999999999999147, -33.29062499938549280, -103.1828516163667899 ) ) ;
#6896=CARTESIAN_POINT ( 'NONE',  ( -85.15643035625001289, -32.87812499938548427, 98.40857419181659793 ) ) ;
#6898=VERTEX_POINT ( 'NONE', #17332 ) ;
#6899=CARTESIAN_POINT ( 'NONE',  ( 83.77821517812500929, -34.37812499938548427, 102.3871387122750889 ) ) ;
#6903=CARTESIAN_POINT ( 'NONE',  ( -83.77821517812500929, -31.56562499938548427, 97.61286128772489690 ) ) ;
#6904=CARTESIAN_POINT ( 'NONE',  ( -81.02178482187500208, -31.34062499938548996, 102.3871387122750889 ) ) ;
#6905=CARTESIAN_POINT ( 'NONE',  ( -82.40000000000000568, -30.00000000000000355, 96.99999999999998579 ) ) ;
#6907=CARTESIAN_POINT ( 'NONE',  ( -85.40000000000000568, -33.18750000000000000, -101.7320508075688679 ) ) ;
#6915=CARTESIAN_POINT ( 'NONE',  ( -81.59615242270660929, -32.32634618820329564, -102.9999999999999858 ) ) ;
#6919=CARTESIAN_POINT ( 'NONE',  ( 82.39999999999999147, -33.96562499938548285, -96.81714838363319586 ) ) ;
#6921=ORIENTED_EDGE ( 'NONE', *, *, #18321, .T. ) ;
#6922=CARTESIAN_POINT ( 'NONE',  ( 83.90000000000000568, -32.26874999877097139, 102.5980762113533018 ) ) ;
#6927=ORIENTED_EDGE ( 'NONE', *, *, #3978, .T. ) ;
#6928=CARTESIAN_POINT ( 'NONE',  ( -82.39999999999999147, -32.72812499938548569, -96.81714838363319586 ) ) ;
#6929=CARTESIAN_POINT ( 'NONE',  ( 79.39999999999999147, -32.41874999877096997, 99.99999999999998579 ) ) ;
#6931=CARTESIAN_POINT ( 'NONE',  ( 82.39999999999999147, -32.61562499938548854, 103.1828516163667899 ) ) ;
#6932=CARTESIAN_POINT ( 'NONE',  ( -83.77821517812500929, -31.07812499938548711, -97.61286128772489690 ) ) ;
#6933=CARTESIAN_POINT ( 'NONE',  ( 79.39999999999999147, -33.33749999999999858, 101.7320508075688821 ) ) ;
#6937=CARTESIAN_POINT ( 'NONE',  ( -85.15643035625001289, -33.25312499938548427, -98.40857419181659793 ) ) ;
#6938=VECTOR ( 'NONE', #8521, 1000.000000000000000 ) ;
#6940=CARTESIAN_POINT ( 'NONE',  ( 80.90000000000000568, -30.99374999877096926, -97.40192378864668399 ) ) ;
#6942=ORIENTED_EDGE ( 'NONE', *, *, #1842, .F. ) ;
#6943=CARTESIAN_POINT ( 'NONE',  ( 79.64356964374999848, -33.96562499938548285, -99.99999999999998579 ) ) ;
#6945=CARTESIAN_POINT ( 'NONE',  ( -82.40000000000001990, -32.53124999877097423, -97.00000000000000000 ) ) ;
#6947=EDGE_CURVE ( 'NONE', #17768, #11098, #294, .T. ) ;
#6950=VERTEX_POINT ( 'NONE', #11466 ) ;
#6954=EDGE_LOOP ( 'NONE', ( #2366, #6561, #8406, #13956 ) ) ;
#6955=CARTESIAN_POINT ( 'NONE',  ( 94.79999999999995453, -35.00000000000000000, 150.0000000000000000 ) ) ;
#6956=CARTESIAN_POINT ( 'NONE',  ( 82.39999999999999147, -32.58750000000000568, -103.4641016151377499 ) ) ;
#6958=CARTESIAN_POINT ( 'NONE',  ( -85.15643035624999868, -32.09062499938548996, 98.40857419181659793 ) ) ;
#6960=CARTESIAN_POINT ( 'NONE',  ( 99.99999999999994316, -21.80000000000003268, -142.6499999999999773 ) ) ;
#6965=VECTOR ( 'NONE', #11126, 1000.000000000000000 ) ;
#6969=CARTESIAN_POINT ( 'NONE',  ( 85.40000000000000568, -34.93124999877096570, 101.7320508075688821 ) ) ;
#6970=CARTESIAN_POINT ( 'NONE',  ( -82.40000000000001990, -33.93750000000000711, 103.0000000000000000 ) ) ;
#6973=ADVANCED_FACE ( 'NONE', ( #8621 ), #5800, .F. ) ;
#6976=CARTESIAN_POINT ( 'NONE',  ( -79.39999999999999147, -30.58124999877096784, 98.26794919243110371 ) ) ;
#6977=CARTESIAN_POINT ( 'NONE',  ( 85.15643035624999868, -34.22812499938547859, 101.5914258081833879 ) ) ;
#6978=CYLINDRICAL_SURFACE ( 'NONE', #6501, 3.000000000000002665 ) ;
#6979=DIRECTION ( 'NONE',  ( -0.000000000000000000, -1.000000000000000000, -0.000000000000000000 ) ) ;
#6981=CARTESIAN_POINT ( 'NONE',  ( -83.77821517812500929, -34.82812499938548711, -102.3871387122750889 ) ) ;
#6982=CARTESIAN_POINT ( 'NONE',  ( 79.64356964374999848, -32.16562499938548569, 99.99999999999998579 ) ) ;
#6984=CARTESIAN_POINT ( 'NONE',  ( 85.15643035624999868, -33.36562499938548854, -101.5914258081833879 ) ) ;
#6986=CARTESIAN_POINT ( 'NONE',  ( -83.77821517812500929, -32.91562499938547859, 97.61286128772489690 ) ) ;
#6987=CARTESIAN_POINT ( 'NONE',  ( 82.39999999999999147, -30.25312499938548783, -96.81714838363319586 ) ) ;
#6988=ADVANCED_FACE ( 'NONE', ( #3941 ), #18885, .F. ) ;
#6990=DIRECTION ( 'NONE',  ( -0.000000000000000000, -1.000000000000000000, -0.000000000000000000 ) ) ;
#6993=CARTESIAN_POINT ( 'NONE',  ( -85.15643035624999868, -33.70312499938548711, 101.5914258081833879 ) ) ;
#6994=CARTESIAN_POINT ( 'NONE',  ( -81.02178482187500208, -30.44062499938548783, 102.3871387122750889 ) ) ;
#6998=EDGE_CURVE ( 'NONE', #7789, #3915, #5177, .T. ) ;
#7001=DIRECTION ( 'NONE',  ( 0.000000000000000000, 0.000000000000000000, -1.000000000000000000 ) ) ;
#7007=CARTESIAN_POINT ( 'NONE',  ( 79.64356964375001269, -32.76562499938548711, -101.5914258081833879 ) ) ;
#7008=CARTESIAN_POINT ( 'NONE',  ( -83.90000000000000568, -33.16874999877096286, 97.40192378864668399 ) ) ;
#7010=CARTESIAN_POINT ( 'NONE',  ( 80.90000000000000568, -32.94374999877096855, 97.40192378864668399 ) ) ;
#7015=CARTESIAN_POINT ( 'NONE',  ( 85.40000000000000568, -34.46249999999999858, 98.26794919243111792 ) ) ;
#7016=DIRECTION ( 'NONE',  ( -1.586032892321652088E-15, -1.000000000000000000, 0.000000000000000000 ) ) ;
#7018=CARTESIAN_POINT ( 'NONE',  ( -85.15643035624999868, -35.05312499938548143, -98.40857419181659793 ) ) ;
#7020=VERTEX_POINT ( 'NONE', #6264 ) ;
#7021=CARTESIAN_POINT ( 'NONE',  ( 85.15643035625001289, -33.36562499938548854, 98.40857419181659793 ) ) ;
#7023=CARTESIAN_POINT ( 'NONE',  ( -81.02178482187500208, -31.00312499938548783, -97.61286128772489690 ) ) ;
#7024=CARTESIAN_POINT ( 'NONE',  ( 80.90000000000000568, -33.75000000000000000, 102.5980762113533018 ) ) ;
#7028=CARTESIAN_POINT ( 'NONE',  ( -82.39999999999999147, -33.17812499938548854, -96.81714838363319586 ) ) ;
#7029=VECTOR ( 'NONE', #282, 1000.000000000000000 ) ;
#7031=CARTESIAN_POINT ( 'NONE',  ( 85.40000000000000568, -31.78124999877096712, -98.26794919243111792 ) ) ;
#7041=VECTOR ( 'NONE', #8531, 1000.000000000000000 ) ;
#7042=CARTESIAN_POINT ( 'NONE',  ( -85.40000000000000568, -32.19374999877096855, 99.99999999999998579 ) ) ;
#7043=ORIENTED_EDGE ( 'NONE', *, *, #12020, .T. ) ;
#7044=CARTESIAN_POINT ( 'NONE',  ( 85.40000000000000568, -32.28750000000000142, -98.26794919243111792 ) ) ;
#7045=CARTESIAN_POINT ( 'NONE',  ( 84.12306224665901766, -31.99999999999999289, -102.1915028381726529 ) ) ;
#7046=CARTESIAN_POINT ( 'NONE',  ( -81.02178482187500208, -32.65312499938548996, 97.61286128772489690 ) ) ;
#7048=CARTESIAN_POINT ( 'NONE',  ( -82.40000000000000568, -34.10624999877096997, 96.99999999999998579 ) ) ;
#7051=CARTESIAN_POINT ( 'NONE',  ( 85.40000000000000568, -34.03124999877096712, 101.7320508075688821 ) ) ;
#7053=DIRECTION ( 'NONE',  ( 0.000000000000000000, 0.000000000000000000, 1.000000000000000000 ) ) ;
#7054=CARTESIAN_POINT ( 'NONE',  ( 94.79999999999991189, -3.000000000000000000, 150.0000000000000000 ) ) ;
#7056=CARTESIAN_POINT ( 'NONE',  ( -85.15643035624999868, -30.62812499938548427, -101.5914258081833879 ) ) ;
#7057=DIRECTION ( 'NONE',  ( -0.000000000000000000, -1.000000000000000000, -0.000000000000000000 ) ) ;
#7063=ORIENTED_EDGE ( 'NONE', *, *, #13529, .T. ) ;
#7066=CARTESIAN_POINT ( 'NONE',  ( -82.85024983566745505, -35.00000000000000711, -102.9730910282409440 ) ) ;
#7068=CARTESIAN_POINT ( 'NONE',  ( 85.15643035625001289, -33.74062499938548854, 99.99999999999998579 ) ) ;
#7070=FACE_OUTER_BOUND ( 'NONE', #4688, .T. ) ;
#7072=CARTESIAN_POINT ( 'NONE',  ( -79.64356964374998427, -33.66562499938548569, -98.40857419181659793 ) ) ;
#7076=EDGE_CURVE ( 'NONE', #10346, #10326, #1854, .T. ) ;
#7077=CARTESIAN_POINT ( 'NONE',  ( 85.15643035624999868, -34.71562499938548285, -101.5914258081833879 ) ) ;
#7079=CARTESIAN_POINT ( 'NONE',  ( -85.15643035625001289, -33.32812499938548711, 98.40857419181659793 ) ) ;
#7080=CARTESIAN_POINT ( 'NONE',  ( 83.77821517812500929, -32.01562499938548001, -97.61286128772489690 ) ) ;
#7085=CARTESIAN_POINT ( 'NONE',  ( -81.02178482187500208, -34.34062499938548285, 97.61286128772489690 ) ) ;
#7086=CARTESIAN_POINT ( 'NONE',  ( -85.15643035625001289, -31.49062499938548498, 99.99999999999998579 ) ) ;
#7092=CARTESIAN_POINT ( 'NONE',  ( 81.48596794228853923, -34.99999999999999289, -97.18639806692210925 ) ) ;
#7096=CARTESIAN_POINT ( 'NONE',  ( -83.95700771753406855, -35.00000000000000711, 97.42750194505822492 ) ) ;
#7099=CARTESIAN_POINT ( 'NONE',  ( -83.20384757729333103, -33.18615380933863435, -103.0000000000000000 ) ) ;
#7102=VECTOR ( 'NONE', #9191, 1000.000000000000000 ) ;
#7103=CARTESIAN_POINT ( 'NONE',  ( -85.40000000000000568, -32.60624999877096997, -98.26794919243111792 ) ) ;
#7104=CARTESIAN_POINT ( 'NONE',  ( 85.15643035624999868, -33.44062499938548427, -98.40857419181659793 ) ) ;
#7107=CARTESIAN_POINT ( 'NONE',  ( 85.40000000000000568, -32.15624999877096712, 98.26794919243111792 ) ) ;
#7113=CARTESIAN_POINT ( 'NONE',  ( -84.25709831968909214, -35.00000000000001421, -97.88253972981382844 ) ) ;
#7114=ORIENTED_EDGE ( 'NONE', *, *, #12808, .T. ) ;
#7115=CARTESIAN_POINT ( 'NONE',  ( -81.02178482187500208, -33.44062499938548427, -102.3871387122750889 ) ) ;
#7116=CARTESIAN_POINT ( 'NONE',  ( 81.59615242270660929, -32.32634618820329564, 102.9999999999999858 ) ) ;
#7117=EDGE_LOOP ( 'NONE', ( #5060, #157, #5898, #9953 ) ) ;
#7118=CARTESIAN_POINT ( 'NONE',  ( -82.40000000000000568, -30.00000000000000355, -99.99999999999998579 ) ) ;
#7120=CARTESIAN_POINT ( 'NONE',  ( -81.02178482187500208, -30.40312499938548640, -102.3871387122750889 ) ) ;
#7121=CARTESIAN_POINT ( 'NONE',  ( -79.39999999999999147, -30.58124999877096784, -101.7320508075688821 ) ) ;
#7122=CARTESIAN_POINT ( 'NONE',  ( -81.48596794228825502, -35.00000000000001421, 97.18639806692218031 ) ) ;
#7125=AXIS2_PLACEMENT_3D ( 'NONE', #9203, #15168, #4729 ) ;
#7126=CARTESIAN_POINT ( 'NONE',  ( -81.02178482187500208, -32.69062499938548427, -97.61286128772489690 ) ) ;
#7127=CARTESIAN_POINT ( 'NONE',  ( -79.39999999999999147, -34.25624999877096855, -98.26794919243113213 ) ) ;
#7128=CARTESIAN_POINT ( 'NONE',  ( 83.90000000000000568, -31.81874999877096855, -97.40192378864668399 ) ) ;
#7130=ORIENTED_EDGE ( 'NONE', *, *, #15919, .T. ) ;
#7131=CARTESIAN_POINT ( 'NONE',  ( 85.15643035625001289, -34.22812499938548569, -98.40857419181659793 ) ) ;
#7135=CARTESIAN_POINT ( 'NONE',  ( -96.99999999999998579, 0.000000000000000000, 150.0000000000000000 ) ) ;
#7141=CIRCLE ( 'NONE', #3702, 5.199999999999996625 ) ;
#7143=EDGE_LOOP ( 'NONE', ( #2243, #16176, #2352, #12996 ) ) ;
#7144=CARTESIAN_POINT ( 'NONE',  ( 81.59615242270660929, -32.32634618820329564, -96.99999999999997158 ) ) ;
#7145=CARTESIAN_POINT ( 'NONE',  ( 85.40000000000000568, -33.18750000000000000, -98.26794919243111792 ) ) ;
#7146=LINE ( 'NONE', #19067, #1751 ) ;
#7147=CARTESIAN_POINT ( 'NONE',  ( -79.64356964375001269, -30.96562499938548640, 101.5914258081833879 ) ) ;
#7153=DIRECTION ( 'NONE',  ( 1.000000000000000000, 0.000000000000000000, -0.000000000000000000 ) ) ;
#7154=CARTESIAN_POINT ( 'NONE',  ( -83.20384757729338787, -34.59240381056766722, -102.9999999999999858 ) ) ;
#7156=( NAMED_UNIT ( * ) PLANE_ANGLE_UNIT ( ) SI_UNIT ( $, .RADIAN. ) );
#7157=CARTESIAN_POINT ( 'NONE',  ( -85.15643035625001289, -30.59062499938548285, -99.99999999999998579 ) ) ;
#7162=CARTESIAN_POINT ( 'NONE',  ( 79.39999999999999147, -32.47500000000000142, 99.99999999999998579 ) ) ;
#7166=CARTESIAN_POINT ( 'NONE',  ( -79.39999999999999147, -30.65624999877096712, 101.7320508075688537 ) ) ;
#7167=CARTESIAN_POINT ( 'NONE',  ( 82.39999999999999147, -30.56250000000000355, 103.4641016151377499 ) ) ;
#7172=CARTESIAN_POINT ( 'NONE',  ( -79.64356964374999848, -34.07812499938548711, -99.99999999999998579 ) ) ;
#7173=CARTESIAN_POINT ( 'NONE',  ( 83.77821517812500929, -34.71562499938548285, 102.3871387122750889 ) ) ;
#7174=CARTESIAN_POINT ( 'NONE',  ( 82.39999999999999147, -32.05312499938548854, -96.81714838363319586 ) ) ;
#7176=CARTESIAN_POINT ( 'NONE',  ( -82.39999999999999147, -33.40312499938548285, 96.81714838363319586 ) ) ;
#7182=CARTESIAN_POINT ( 'NONE',  ( -79.64356964375001269, -33.02812499938548285, 98.40857419181659793 ) ) ;
#7183=ORIENTED_EDGE ( 'NONE', *, *, #6023, .T. ) ;
#7187=CARTESIAN_POINT ( 'NONE',  ( 85.40000000000000568, -33.60000000000000142, -99.99999999999998579 ) ) ;
#7192=CARTESIAN_POINT ( 'NONE',  ( 79.64356964375001269, -33.66562499938549280, 98.40857419181659793 ) ) ;
#7195=CARTESIAN_POINT ( 'NONE',  ( 82.39999999999999147, -33.51562499938548001, -96.81714838363319586 ) ) ;
#7196=CARTESIAN_POINT ( 'NONE',  ( -82.39999999999999147, -30.36562499938549209, -103.1828516163667899 ) ) ;
#7198=CARTESIAN_POINT ( 'NONE',  ( 83.90000000000000568, -32.11874999877097281, 97.40192378864668399 ) ) ;
#7203=CARTESIAN_POINT ( 'NONE',  ( -85.15643035624999868, -33.70312499938548711, -98.40857419181659793 ) ) ;
#7204=PLANE ( 'NONE',  #3180 ) ;
#7206=ORIENTED_EDGE ( 'NONE', *, *, #19047, .F. ) ;
#7208=CARTESIAN_POINT ( 'NONE',  ( -82.39999999999999147, -31.49062499938548854, -96.81714838363319586 ) ) ;
#7210=CARTESIAN_POINT ( 'NONE',  ( -85.40000000000000568, -31.78124999877096712, -101.7320508075688679 ) ) ;
#7214=CARTESIAN_POINT ( 'NONE',  ( -82.39999999999999147, -32.05312499938548854, -103.1828516163667899 ) ) ;
#7216=CARTESIAN_POINT ( 'NONE',  ( -79.39999999999999147, -34.18124999877097281, -101.7320508075688963 ) ) ;
#7217=CARTESIAN_POINT ( 'NONE',  ( 79.39999999999999147, -31.96874999877096712, -99.99999999999998579 ) ) ;
#7219=EDGE_CURVE ( 'NONE', #5564, #17054, #3859, .T. ) ;
#7220=ORIENTED_EDGE ( 'NONE', *, *, #1234, .T. ) ;
#7221=CARTESIAN_POINT ( 'NONE',  ( 85.15643035625001289, -34.15312499938548285, -101.5914258081833879 ) ) ;
#7224=EDGE_CURVE ( 'NONE', #5172, #5491, #19041, .T. ) ;
#7229=CARTESIAN_POINT ( 'NONE',  ( -80.52691934816502339, -34.99999999999999289, -97.94626448418668474 ) ) ;
#7233=DIRECTION ( 'NONE',  ( -0.000000000000000000, -0.000000000000000000, -1.000000000000000000 ) ) ;
#7234=CARTESIAN_POINT ( 'NONE',  ( 82.15584532983331201, -31.99999999999999289, -102.8696726379688329 ) ) ;
#7236=( BOUNDED_CURVE ( )  B_SPLINE_CURVE ( 2, ( #10194, #11368, #16157, #2768, #8724, #14677, #13215, #19186, #5802 ),
 .UNSPECIFIED., .F., .F. ) 
 B_SPLINE_CURVE_WITH_KNOTS ( ( 3, 2, 2, 2, 3 ),
 ( 0.7291666666666668517, 0.7361111111111111605, 0.7500000000000000000, 0.7638888888888888395, 0.7708333333333332593 ),
 .UNSPECIFIED. ) 
 CURVE ( )  GEOMETRIC_REPRESENTATION_ITEM ( )  RATIONAL_B_SPLINE_CURVE ( ( 0.9330127018922194093, 0.9330127018922209636, 1.000000000000000000, 0.8660254037844387076, 1.000000000000000000, 0.8660254037844387076, 1.000000000000000000, 0.9330127018922198534, 0.9330127018922192983 ) ) 
 REPRESENTATION_ITEM ( '' )  );
#7237=CARTESIAN_POINT ( 'NONE',  ( -83.77821517812500929, -31.07812499938548711, 102.3871387122750889 ) ) ;
#7241=FACE_OUTER_BOUND ( 'NONE', #7439, .T. ) ;
#7242=CARTESIAN_POINT ( 'NONE',  ( 85.00132729414795563, -34.99999999999999289, 98.78874432549832818 ) ) ;
#7244=ORIENTED_EDGE ( 'NONE', *, *, #8793, .T. ) ;
#7245=CARTESIAN_POINT ( 'NONE',  ( -79.64356964375001269, -30.77812499938548285, -101.5914258081833879 ) ) ;
#7247=VECTOR ( 'NONE', #13607, 1000.000000000000000 ) ;
#7252=EDGE_CURVE ( 'NONE', #11363, #3019, #9961, .T. ) ;
#7258=CARTESIAN_POINT ( 'NONE',  ( 82.40000000000000568, -32.30624999877097281, -97.00000000000000000 ) ) ;
#7259=CARTESIAN_POINT ( 'NONE',  ( 80.90000000000000568, -30.15000000000000213, 102.5980762113533018 ) ) ;
#7260=PLANE ( 'NONE',  #14916 ) ;
#7265=CARTESIAN_POINT ( 'NONE',  ( 79.64356964375001269, -34.00312499938549138, 98.40857419181659793 ) ) ;
#7266=CARTESIAN_POINT ( 'NONE',  ( 81.02178482187500208, -32.54062499938548569, -97.61286128772489690 ) ) ;
#7271=CARTESIAN_POINT ( 'NONE',  ( 79.64356964374999848, -34.07812499938548711, 99.99999999999998579 ) ) ;
#7275=CARTESIAN_POINT ( 'NONE',  ( -81.02178482187500208, -33.59062499938548285, 102.3871387122750889 ) ) ;
#7277=CARTESIAN_POINT ( 'NONE',  ( -83.65502553130849606, -35.00000000000002842, 102.4885329066896702 ) ) ;
#7280=( BOUNDED_CURVE ( )  B_SPLINE_CURVE ( 2, ( #9002, #17805, #5981, #8807, #7535, #2945, #14962, #8898, #14764 ),
 .UNSPECIFIED., .F., .F. ) 
 B_SPLINE_CURVE_WITH_KNOTS ( ( 3, 2, 2, 2, 3 ),
 ( 0.6458333333333332593, 0.6527777777777777901, 0.6666666666666666297, 0.6805555555555555802, 0.6875000000000000000 ),
 .UNSPECIFIED. ) 
 CURVE ( )  GEOMETRIC_REPRESENTATION_ITEM ( )  RATIONAL_B_SPLINE_CURVE ( ( 0.9330127018922192983, 0.9330127018922187432, 1.000000000000000000, 0.8660254037844387076, 1.000000000000000000, 0.8660254037844387076, 1.000000000000000000, 0.9330127018922194093, 0.9330127018922194093 ) ) 
 REPRESENTATION_ITEM ( '' )  );
#7282=CARTESIAN_POINT ( 'NONE',  ( 82.40000000000001990, -34.16250000000000853, -97.00000000000000000 ) ) ;
#7283=CARTESIAN_POINT ( 'NONE',  ( -80.08630547029558500, -32.02340763552836478, 102.1282894555903198 ) ) ;
#7286=CARTESIAN_POINT ( 'NONE',  ( 83.77821517812500929, -33.77812499938548285, 97.61286128772489690 ) ) ;
#7289=CARTESIAN_POINT ( 'NONE',  ( 85.15643035625001289, -33.40312499938548285, -99.99999999999998579 ) ) ;
#7290=CARTESIAN_POINT ( 'NONE',  ( -82.39999999999999147, -32.16562499938549280, -103.1828516163667899 ) ) ;
#7291=EDGE_LOOP ( 'NONE', ( #3448, #7494, #8733, #10380 ) ) ;
#7292=CARTESIAN_POINT ( 'NONE',  ( 80.90000000000000568, -32.04374999877096997, 97.40192378864668399 ) ) ;
#7294=CARTESIAN_POINT ( 'NONE',  ( 85.40000000000000568, -34.48124999877096997, 101.7320508075688821 ) ) ;
#7295=CARTESIAN_POINT ( 'NONE',  ( 80.80006050682045782, -31.99999999999997868, 102.4537706361795131 ) ) ;
#7297=CARTESIAN_POINT ( 'NONE',  ( -81.02178482187500208, -34.49062499938548854, -97.61286128772489690 ) ) ;
#7301=CARTESIAN_POINT ( 'NONE',  ( -79.64356964374999848, -34.52812499938548285, -99.99999999999998579 ) ) ;
#7303=CARTESIAN_POINT ( 'NONE',  ( -79.39999999999999147, -30.61874999877096926, -99.99999999999998579 ) ) ;
#7307=CARTESIAN_POINT ( 'NONE',  ( -85.40000000000000568, -33.50624999877096855, 101.7320508075688821 ) ) ;
#7310=( BOUNDED_CURVE ( )  B_SPLINE_CURVE ( 2, ( #10049, #16007, #6135, #15111, #3189, #17957, #3093, #13829, #4771 ),
 .UNSPECIFIED., .F., .F. ) 
 B_SPLINE_CURVE_WITH_KNOTS ( ( 3, 2, 2, 2, 3 ),
 ( 0.8125000000000001110, 0.8194444444444444198, 0.8333333333333333703, 0.8472222222222222099, 0.8530683953269213582 ),
 .UNSPECIFIED. ) 
 CURVE ( )  GEOMETRIC_REPRESENTATION_ITEM ( )  RATIONAL_B_SPLINE_CURVE ( ( 0.9330127018922194093, 0.9330127018922204085, 1.000000000000000000, 0.8660254037844387076, 1.000000000000000000, 0.8660254037844387076, 1.000000000000000000, 0.9436068149601996025, 0.9346881722405915305 ) ) 
 REPRESENTATION_ITEM ( '' )  );
#7311=CARTESIAN_POINT ( 'NONE',  ( -82.40000000000001990, -33.93750000000000711, -97.00000000000000000 ) ) ;
#7312=CARTESIAN_POINT ( 'NONE',  ( 79.39999999999999147, -31.06874999877096855, -99.99999999999998579 ) ) ;
#7315=EDGE_CURVE ( 'NONE', #15349, #16451, #9397, .T. ) ;
#7316=VERTEX_POINT ( 'NONE', #8477 ) ;
#7317=CARTESIAN_POINT ( 'NONE',  ( 85.15643035625001289, -34.67812499938548143, -98.40857419181659793 ) ) ;
#7322=ORIENTED_EDGE ( 'NONE', *, *, #7470, .T. ) ;
#7323=VERTEX_POINT ( 'NONE', #17576 ) ;
#7324=CARTESIAN_POINT ( 'NONE',  ( -83.52022063339109081, -31.99999999999999289, 97.42682425340038321 ) ) ;
#7329=CARTESIAN_POINT ( 'NONE',  ( 84.70388354820681798, -35.00002705695767702, 101.9214814096700934 ) ) ;
#7330=DIRECTION ( 'NONE',  ( -0.000000000000000000, -1.000000000000000000, -0.000000000000000000 ) ) ;
#7332=CARTESIAN_POINT ( 'NONE',  ( -83.77821517812500929, -33.77812499938548285, 102.3871387122750889 ) ) ;
#7340=ORIENTED_EDGE ( 'NONE', *, *, #15097, .F. ) ;
#7341=CARTESIAN_POINT ( 'NONE',  ( 0.000000000000000000, 0.000000000000000000, 0.000000000000000000 ) ) ;
#7342=CARTESIAN_POINT ( 'NONE',  ( -81.02178482187500208, -34.90312499938548285, -102.3871387122750889 ) ) ;
#7346=CARTESIAN_POINT ( 'NONE',  ( -83.20384757729335945, -32.73615380933863150, 96.99999999999998579 ) ) ;
#7352=ORIENTED_EDGE ( 'NONE', *, *, #11128, .T. ) ;
#7355=CARTESIAN_POINT ( 'NONE',  ( -80.90000000000000568, -30.99374999877096926, 97.40192378864668399 ) ) ;
#7356=CARTESIAN_POINT ( 'NONE',  ( 83.77821517812500929, -34.56562499938548427, 97.61286128772489690 ) ) ;
#7357=CYLINDRICAL_SURFACE ( 'NONE', #9621, 3.000000000000002665 ) ;
#7359=AXIS2_PLACEMENT_3D ( 'NONE', #12469, #12377, #666 ) ;
#7361=CARTESIAN_POINT ( 'NONE',  ( 79.64356964374999848, -34.41562499938548569, 99.99999999999998579 ) ) ;
#7362=CARTESIAN_POINT ( 'NONE',  ( 85.15643035624999868, -31.07812499938548356, -98.40857419181659793 ) ) ;
#7364=DIRECTION ( 'NONE',  ( 0.000000000000000000, -1.000000000000000000, 0.000000000000000000 ) ) ;
#7365=CARTESIAN_POINT ( 'NONE',  ( 79.64356964375001269, -32.12812499938548427, -98.40857419181659793 ) ) ;
#7368=LINE ( 'NONE', #7467, #7247 ) ;
#7372=CARTESIAN_POINT ( 'NONE',  ( -83.77821517812500929, -33.21562499938548285, 102.3871387122750889 ) ) ;
#7374=CARTESIAN_POINT ( 'NONE',  ( -82.39999999999999147, -32.81250000000000000, 97.00000000000000000 ) ) ;
#7382=CARTESIAN_POINT ( 'NONE',  ( 79.64356964375001269, -31.86562499938548143, 98.40857419181659793 ) ) ;
#7383=LINE ( 'NONE', #13343, #11150 ) ;
#7387=CARTESIAN_POINT ( 'NONE',  ( -83.77821517812500929, -31.22812499938548569, -102.3871387122750889 ) ) ;
#7389=CARTESIAN_POINT ( 'NONE',  ( 85.40000000000000568, -35.30624999877096570, 98.26794919243111792 ) ) ;
#7392=CARTESIAN_POINT ( 'NONE',  ( -83.77821517812500929, -31.67812499938548498, 97.61286128772489690 ) ) ;
#7393=CARTESIAN_POINT ( 'NONE',  ( 79.39999999999999147, -33.73124999877096997, -98.26794919243110371 ) ) ;
#7395=CARTESIAN_POINT ( 'NONE',  ( -83.77821517812500929, -35.01562499938548711, -97.61286128772489690 ) ) ;
#7398=CARTESIAN_POINT ( 'NONE',  ( -83.77821517812500929, -33.02812499938548285, -102.3871387122750889 ) ) ;
#7401=CARTESIAN_POINT ( 'NONE',  ( -82.39999999999999147, -30.73124999877096641, -96.53589838486223584 ) ) ;
#7405=CARTESIAN_POINT ( 'NONE',  ( -82.39999999999999147, -34.07812499938548711, -96.81714838363319586 ) ) ;
#7406=CARTESIAN_POINT ( 'NONE',  ( 81.02178482187500208, -34.49062499938548854, 97.61286128772489690 ) ) ;
#7409=CARTESIAN_POINT ( 'NONE',  ( 79.39999999999999147, -34.70624999877097139, -101.7320508075688537 ) ) ;
#7413=CARTESIAN_POINT ( 'NONE',  ( 79.64356964374999848, -34.41562499938548569, -99.99999999999998579 ) ) ;
#7419=ORIENTED_EDGE ( 'NONE', *, *, #2537, .T. ) ;
#7420=ORIENTED_EDGE ( 'NONE', *, *, #13639, .T. ) ;
#7424=ORIENTED_EDGE ( 'NONE', *, *, #7927, .F. ) ;
#7425=CARTESIAN_POINT ( 'NONE',  ( -80.80861089413673426, -34.99999999999999289, 102.2789443502789055 ) ) ;
#7427=AXIS2_PLACEMENT_3D ( 'NONE', #10084, #7053, #7153 ) ;
#7428=EDGE_CURVE ( 'NONE', #4491, #7737, #17397, .T. ) ;
#7429=CIRCLE ( 'NONE', #8052, 2.199999999999993516 ) ;
#7430=CARTESIAN_POINT ( 'NONE',  ( -82.39999999999999147, -34.41562499938547859, 96.81714838363319586 ) ) ;
#7432=( BOUNDED_CURVE ( )  B_SPLINE_CURVE ( 2, ( #5969, #7144, #4497, #4206, #8984, #13189, #11724, #10452, #13094 ),
 .UNSPECIFIED., .F., .F. ) 
 B_SPLINE_CURVE_WITH_KNOTS ( ( 3, 2, 2, 2, 3 ),
 ( 0.3541666666666666297, 0.3611111111111111049, 0.3750000000000000000, 0.3888888888888888951, 0.3958333333333334259 ),
 .UNSPECIFIED. ) 
 CURVE ( )  GEOMETRIC_REPRESENTATION_ITEM ( )  RATIONAL_B_SPLINE_CURVE ( ( 0.9330127018922194093, 0.9330127018922190762, 1.000000000000000000, 0.8660254037844387076, 1.000000000000000000, 0.8660254037844387076, 1.000000000000000000, 0.9330127018922185211, 0.9330127018922192983 ) ) 
 REPRESENTATION_ITEM ( '' )  );
#7436=CARTESIAN_POINT ( 'NONE',  ( 79.60045861139946055, -35.00000000000000711, 100.3117415790902953 ) ) ;
#7437=CARTESIAN_POINT ( 'NONE',  ( -82.40000000000000568, -30.00000000000000355, 96.99999999999998579 ) ) ;
#7439=EDGE_LOOP ( 'NONE', ( #11843, #4230, #4124, #391 ) ) ;
#7440=CARTESIAN_POINT ( 'NONE',  ( -79.64356964375001269, -33.55312499938548854, -98.40857419181659793 ) ) ;
#7448=ORIENTED_EDGE ( 'NONE', *, *, #19056, .T. ) ;
#7450=CARTESIAN_POINT ( 'NONE',  ( -84.85729912020876498, -32.00000000000000000, 101.2614033343865856 ) ) ;
#7453=CARTESIAN_POINT ( 'NONE',  ( -82.39999999999999147, -31.40624999877097068, 96.53589838486223584 ) ) ;
#7454=CARTESIAN_POINT ( 'NONE',  ( 79.39999999999999147, -31.12500000000000355, 99.99999999999998579 ) ) ;
#7458=CARTESIAN_POINT ( 'NONE',  ( 79.64356964375001269, -34.45312499938548711, 98.40857419181659793 ) ) ;
#7459=CARTESIAN_POINT ( 'NONE',  ( 85.15643035625001289, -31.49062499938548498, -99.99999999999998579 ) ) ;
#7460=VERTEX_POINT ( 'NONE', #18694 ) ;
#7462=DIRECTION ( 'NONE',  ( 0.000000000000000000, 0.000000000000000000, 1.000000000000000000 ) ) ;
#7463=CARTESIAN_POINT ( 'NONE',  ( 85.15643035625001289, -34.19062499938548427, -99.99999999999998579 ) ) ;
#7464=( BOUNDED_CURVE ( )  B_SPLINE_CURVE ( 2, ( #19031, #13067, #2606, #7015, #17280, #3985, #13251, #12968, #10043 ),
 .UNSPECIFIED., .F., .F. ) 
 B_SPLINE_CURVE_WITH_KNOTS ( ( 3, 2, 2, 2, 3 ),
 ( 0.8125000000000000000, 0.8194444444444444198, 0.8333333333333333703, 0.8472222222222222099, 0.8541666666666665186 ),
 .UNSPECIFIED. ) 
 CURVE ( )  GEOMETRIC_REPRESENTATION_ITEM ( )  RATIONAL_B_SPLINE_CURVE ( ( 0.9330127018922194093, 0.9330127018922194093, 1.000000000000000000, 0.8660254037844387076, 1.000000000000000000, 0.8660254037844387076, 1.000000000000000000, 0.9330127018922209636, 0.9330127018922194093 ) ) 
 REPRESENTATION_ITEM ( '' )  );
#7465=EDGE_CURVE ( 'NONE', #7832, #609, #438, .T. ) ;
#7467=CARTESIAN_POINT ( 'NONE',  ( -82.40000000000000568, -30.00000000000000355, 103.0000000000000000 ) ) ;
#7468=CARTESIAN_POINT ( 'NONE',  ( 82.40000000000000568, -33.93750000000000711, -102.9999999999999858 ) ) ;
#7470=EDGE_CURVE ( 'NONE', #9248, #1356, #18398, .T. ) ;
#7471=CARTESIAN_POINT ( 'NONE',  ( -83.25523545990762386, -35.19352049914630953, 96.73097394877602540 ) ) ;
#7479=CARTESIAN_POINT ( 'NONE',  ( -81.59615242270663771, -32.51115380933863008, 103.0000000000000000 ) ) ;
#7482=CARTESIAN_POINT ( 'NONE',  ( 81.02178482187500208, -31.45312499938549067, 97.61286128772489690 ) ) ;
#7483=DIRECTION ( 'NONE',  ( -0.000000000000000000, -1.000000000000000000, -0.000000000000000000 ) ) ;
#7485=CARTESIAN_POINT ( 'NONE',  ( -79.64356964374998427, -32.31562499938548427, 101.5914258081833879 ) ) ;
#7486=CARTESIAN_POINT ( 'NONE',  ( -79.64356964375001269, -30.51562499938548711, -98.40857419181659793 ) ) ;
#7487=ORIENTED_EDGE ( 'NONE', *, *, #19050, .T. ) ;
#7488=CARTESIAN_POINT ( 'NONE',  ( 79.39999999999999147, -34.70624999877097139, 98.26794919243113213 ) ) ;
#7492=CARTESIAN_POINT ( 'NONE',  ( -79.64356964375001269, -30.96562499938548640, 101.5914258081833879 ) ) ;
#7493=CARTESIAN_POINT ( 'NONE',  ( 84.28136653320183314, -32.00000000000000711, 102.0145392219077394 ) ) ;
#7494=ORIENTED_EDGE ( 'NONE', *, *, #10846, .F. ) ;
#7496=CARTESIAN_POINT ( 'NONE',  ( -79.39999999999999147, -30.18750000000000355, -101.7320508075688821 ) ) ;
#7499=CARTESIAN_POINT ( 'NONE',  ( -82.39999999999999147, -32.61562499938548854, -103.1828516163667899 ) ) ;
#7504=CARTESIAN_POINT ( 'NONE',  ( 85.15643035625001289, -33.74062499938548854, 99.99999999999998579 ) ) ;
#7505=LINE ( 'NONE', #13265, #16468 ) ;
#7506=CARTESIAN_POINT ( 'NONE',  ( 99.99999999999997158, -5.200000000000008171, 150.0000000000000000 ) ) ;
#7507=CARTESIAN_POINT ( 'NONE',  ( 82.39999999999999147, -35.23124999877096997, -103.4641016151377499 ) ) ;
#7514=ORIENTED_EDGE ( 'NONE', *, *, #8745, .T. ) ;
#7518=( BOUNDED_CURVE ( )  B_SPLINE_CURVE ( 2, ( #9155, #15118, #13649, #7307, #5855, #13264, #11809, #13745, #18156 ),
 .UNSPECIFIED., .F., .F. ) 
 B_SPLINE_CURVE_WITH_KNOTS ( ( 3, 2, 2, 2, 3 ),
 ( 0.5625000000000000000, 0.5694444444444444198, 0.5833333333333333703, 0.5972222222222222099, 0.6041666666666666297 ),
 .UNSPECIFIED. ) 
 CURVE ( )  GEOMETRIC_REPRESENTATION_ITEM ( )  RATIONAL_B_SPLINE_CURVE ( ( 0.9330127018922194093, 0.9330127018922194093, 1.000000000000000000, 0.8660254037844387076, 1.000000000000000000, 0.8660254037844387076, 1.000000000000000000, 0.9330127018922198534, 0.9330127018922192983 ) ) 
 REPRESENTATION_ITEM ( '' )  );
#7519=FACE_BOUND ( 'NONE', #4692, .T. ) ;
#7522=DIRECTION ( 'NONE',  ( -1.000000000000000000, -0.000000000000000000, -0.000000000000000000 ) ) ;
#7524=CARTESIAN_POINT ( 'NONE',  ( -79.64356964374999848, -33.17812499938548854, 99.99999999999998579 ) ) ;
#7528=CARTESIAN_POINT ( 'NONE',  ( -99.99999999999998579, -35.00000000000000000, 150.0000000000000000 ) ) ;
#7529=CARTESIAN_POINT ( 'NONE',  ( -79.77811200999879304, -35.00000000000000000, -99.14934632385212865 ) ) ;
#7532=VERTEX_POINT ( 'NONE', #13195 ) ;
#7534=CARTESIAN_POINT ( 'NONE',  ( -79.64356964374999848, -32.61562499938548854, -99.99999999999998579 ) ) ;
#7535=CARTESIAN_POINT ( 'NONE',  ( -85.40000000000000568, -33.60000000000000142, 99.99999999999998579 ) ) ;
#7536=CARTESIAN_POINT ( 'NONE',  ( 99.99999999999994316, -29.80000000000000782, 150.0000000000000000 ) ) ;
#7543=DIRECTION ( 'NONE',  ( 0.000000000000000000, 0.000000000000000000, 1.000000000000000000 ) ) ;
#7545=CARTESIAN_POINT ( 'NONE',  ( -85.40000000000000568, -33.09374999877096712, 99.99999999999998579 ) ) ;
#7546=CARTESIAN_POINT ( 'NONE',  ( 83.90000000000000568, -32.17500000000000426, 97.40192378864668399 ) ) ;
#7547=CARTESIAN_POINT ( 'NONE',  ( -82.39076102795762324, -32.00000000000001421, -97.13047754280714230 ) ) ;
#7550=LINE ( 'NONE', #18210, #19307 ) ;
#7552=AXIS2_PLACEMENT_3D ( 'NONE', #1849, #6545, #14148 ) ;
#7554=CARTESIAN_POINT ( 'NONE',  ( 79.64356964374999848, -30.81562499938548427, -99.99999999999998579 ) ) ;
#7555=ORIENTED_EDGE ( 'NONE', *, *, #16104, .F. ) ;
#7557=FACE_OUTER_BOUND ( 'NONE', #11603, .T. ) ;
#7558=CARTESIAN_POINT ( 'NONE',  ( 81.02178482187500208, -34.34062499938548285, -97.61286128772489690 ) ) ;
#7560=CARTESIAN_POINT ( 'NONE',  ( 82.40000000000000568, -30.00000000000000355, -99.99999999999998579 ) ) ;
#7563=CARTESIAN_POINT ( 'NONE',  ( -83.90000000000000568, -30.82500000000000284, 102.5980762113533018 ) ) ;
#7564=ORIENTED_EDGE ( 'NONE', *, *, #17408, .T. ) ;
#7565=CARTESIAN_POINT ( 'NONE',  ( -84.97511176747894979, -34.99999999999999289, 98.48300226794593470 ) ) ;
#7567=CIRCLE ( 'NONE', #11932, 5.199999999999996625 ) ;
#7569=CARTESIAN_POINT ( 'NONE',  ( 81.02178482187500208, -30.44062499938548783, 97.61286128772489690 ) ) ;
#7572=CARTESIAN_POINT ( 'NONE',  ( -85.40000000000000568, -33.18750000000000000, -101.7320508075688821 ) ) ;
#7573=CARTESIAN_POINT ( 'NONE',  ( 96.99999999999997158, -5.200000000000003730, 150.0000000000000000 ) ) ;
#7575=CARTESIAN_POINT ( 'NONE',  ( 79.64356964375001269, -30.32812499938548711, 101.5914258081833879 ) ) ;
#7577=FACE_OUTER_BOUND ( 'NONE', #17998, .T. ) ;
#7580=DIRECTION ( 'NONE',  ( 0.000000000000000000, 1.000000000000000000, 0.000000000000000000 ) ) ;
#7581=CARTESIAN_POINT ( 'NONE',  ( -85.15643035624999868, -31.64062499938548356, -101.5914258081833879 ) ) ;
#7584=CARTESIAN_POINT ( 'NONE',  ( 80.90000000000000568, -34.74374999877097281, 97.40192378864668399 ) ) ;
#7585=CARTESIAN_POINT ( 'NONE',  ( 83.20384757729337366, -34.35134618820330843, 97.00000000000000000 ) ) ;
#7587=CARTESIAN_POINT ( 'NONE',  ( -85.15643035624999868, -31.19062499938548783, 98.40857419181659793 ) ) ;
#7588=CARTESIAN_POINT ( 'NONE',  ( -84.97511176747885031, -35.00000000000002132, -101.5169977320541790 ) ) ;
#7589=ORIENTED_EDGE ( 'NONE', *, *, #11638, .F. ) ;
#7590=CARTESIAN_POINT ( 'NONE',  ( -79.39999999999999147, -32.02500000000000568, -99.99999999999998579 ) ) ;
#7591=CARTESIAN_POINT ( 'NONE',  ( 82.40000000000001990, -32.53124999877097423, 97.00000000000000000 ) ) ;
#7593=CARTESIAN_POINT ( 'NONE',  ( -81.02178482187500208, -32.80312499938548854, -97.61286128772489690 ) ) ;
#7594=CARTESIAN_POINT ( 'NONE',  ( -84.28136653320150629, -32.00000000000001421, -102.0145392219080378 ) ) ;
#7599=CARTESIAN_POINT ( 'NONE',  ( 85.15643035625001289, -34.19062499938548427, 99.99999999999998579 ) ) ;
#7601=DIRECTION ( 'NONE',  ( -0.000000000000000000, -1.000000000000000000, -0.000000000000000000 ) ) ;
#7602=EDGE_CURVE ( 'NONE', #14237, #7460, #4028, .T. ) ;
#7603=CARTESIAN_POINT ( 'NONE',  ( 85.40000000000000568, -35.34374999877096712, -99.99999999999998579 ) ) ;
#7614=FACE_OUTER_BOUND ( 'NONE', #11669, .T. ) ;
#7616=CARTESIAN_POINT ( 'NONE',  ( 82.40000000000000568, -33.03750000000000142, 96.99999999999998579 ) ) ;
#7620=CARTESIAN_POINT ( 'NONE',  ( -81.02178482187500208, -34.00312499938548427, 97.61286128772489690 ) ) ;
#7625=FACE_BOUND ( 'NONE', #986, .T. ) ;
#7626=CARTESIAN_POINT ( 'NONE',  ( -82.65333140691201663, -34.99995246259153703, -102.9892844631211943 ) ) ;
#7629=CARTESIAN_POINT ( 'NONE',  ( -79.64356964375001269, -34.45312499938548711, -98.40857419181659793 ) ) ;
#7633=CARTESIAN_POINT ( 'NONE',  ( -85.40000000000000568, -32.60624999877096997, 101.7320508075688821 ) ) ;
#7634=CARTESIAN_POINT ( 'NONE',  ( -82.40000000000001990, -34.61250000000001137, -103.0000000000000000 ) ) ;
#7638=CARTESIAN_POINT ( 'NONE',  ( -85.40000000000000568, -34.95000000000000284, -99.99999999999998579 ) ) ;
#7640=CARTESIAN_POINT ( 'NONE',  ( -79.39999999999999147, -32.45624999877097139, 101.7320508075688537 ) ) ;
#7641=CARTESIAN_POINT ( 'NONE',  ( 85.40000000000000568, -30.93750000000000355, 101.7320508075688679 ) ) ;
#7645=AXIS2_PLACEMENT_3D ( 'NONE', #311, #1944, #6261 ) ;
#7646=CARTESIAN_POINT ( 'NONE',  ( 81.02178482187500208, -32.99062499938548854, -97.61286128772489690 ) ) ;
#7649=DIRECTION ( 'NONE',  ( 0.000000000000000000, -0.000000000000000000, 1.000000000000000000 ) ) ;
#7650=CARTESIAN_POINT ( 'NONE',  ( 83.77821517812500929, -33.36562499938548854, -97.61286128772489690 ) ) ;
#7651=CARTESIAN_POINT ( 'NONE',  ( 82.40000000000000568, -30.00000000000000355, 99.99999999999998579 ) ) ;
#7654=CARTESIAN_POINT ( 'NONE',  ( -79.64356964374999848, -34.86562499938548143, 99.99999999999998579 ) ) ;
#7655=ORIENTED_EDGE ( 'NONE', *, *, #3251, .T. ) ;
#7658=CARTESIAN_POINT ( 'NONE',  ( -79.39999999999999147, -34.31250000000000000, 101.7320508075688537 ) ) ;
#7659=CARTESIAN_POINT ( 'NONE',  ( 85.15643035624999868, -30.55312499938548854, 98.40857419181659793 ) ) ;
#7666=CARTESIAN_POINT ( 'NONE',  ( 81.02178482187500208, -30.29062499938548569, 102.3871387122750889 ) ) ;
#7669=CARTESIAN_POINT ( 'NONE',  ( 83.77821517812500929, -35.12812499938548427, -102.3871387122750889 ) ) ;
#7670=CARTESIAN_POINT ( 'NONE',  ( -85.15643035624999868, -34.34062499938548285, -101.5914258081833879 ) ) ;
#7673=CARTESIAN_POINT ( 'NONE',  ( 79.39999999999999147, -35.15624999877096712, 98.26794919243113213 ) ) ;
#7678=CARTESIAN_POINT ( 'NONE',  ( -79.64356964375001269, -32.31562499938548427, 101.5914258081833879 ) ) ;
#7681=CARTESIAN_POINT ( 'NONE',  ( -79.39999999999999147, -31.53750000000000497, -101.7320508075688821 ) ) ;
#7685=CARTESIAN_POINT ( 'NONE',  ( -83.77821517812500929, -34.22812499938549280, -97.61286128772489690 ) ) ;
#7690=ORIENTED_EDGE ( 'NONE', *, *, #15093, .T. ) ;
#7692=DIRECTION ( 'NONE',  ( 0.000000000000000000, 0.000000000000000000, -1.000000000000000000 ) ) ;
#7693=CARTESIAN_POINT ( 'NONE',  ( 82.39999999999999147, -33.40312499938548285, 103.1828516163667899 ) ) ;
#7694=DIRECTION ( 'NONE',  ( -0.000000000000000000, 0.000000000000000000, -1.000000000000000000 ) ) ;
#7697=CARTESIAN_POINT ( 'NONE',  ( 85.40000000000000568, -33.09374999877096712, -99.99999999999998579 ) ) ;
#7700=ORIENTED_EDGE ( 'NONE', *, *, #11127, .T. ) ;
#7706=CARTESIAN_POINT ( 'NONE',  ( -85.39999999999999147, -34.97364041986484295, 98.90809577818235709 ) ) ;
#7708=EDGE_LOOP ( 'NONE', ( #1962, #8290, #10439, #7690 ) ) ;
#7709=CARTESIAN_POINT ( 'NONE',  ( -85.15643035624999868, -30.17812499938548498, -101.5914258081833879 ) ) ;
#7711=ORIENTED_EDGE ( 'NONE', *, *, #8055, .T. ) ;
#7715=CARTESIAN_POINT ( 'NONE',  ( -82.39999999999999147, -34.86562499938548854, 96.81714838363319586 ) ) ;
#7722=CARTESIAN_POINT ( 'NONE',  ( 79.39999999999999147, -34.68750000000000000, -98.26794919243110371 ) ) ;
#7724=DIRECTION ( 'NONE',  ( -0.000000000000000000, -1.000000000000000000, -0.000000000000000000 ) ) ;
#7728=CARTESIAN_POINT ( 'NONE',  ( -83.77821517812500929, -33.36562499938548854, -102.3871387122750889 ) ) ;
#7733=CARTESIAN_POINT ( 'NONE',  ( -82.40000000000000568, -30.00000000000000355, 99.99999999999998579 ) ) ;
#7734=VECTOR ( 'NONE', #14557, 1000.000000000000000 ) ;
#7736=ORIENTED_EDGE ( 'NONE', *, *, #4040, .T. ) ;
#7737=VERTEX_POINT ( 'NONE', #8800 ) ;
#7738=CARTESIAN_POINT ( 'NONE',  ( 81.59615242270662350, -34.76115380933863719, 96.99999999999995737 ) ) ;
#7740=CARTESIAN_POINT ( 'NONE',  ( 79.39999999999999147, -30.63750000000000284, -98.26794919243110371 ) ) ;
#7741=CARTESIAN_POINT ( 'NONE',  ( -85.40000000000000568, -33.13124999877096855, 98.26794919243111792 ) ) ;
#7743=CARTESIAN_POINT ( 'NONE',  ( 85.40000000000000568, -32.70000000000000284, 99.99999999999998579 ) ) ;
#7745=CARTESIAN_POINT ( 'NONE',  ( -81.01744233620665625, -32.00000000000001421, -97.41649131116872695 ) ) ;
#7747=CARTESIAN_POINT ( 'NONE',  ( 79.64356964374998427, -33.66562499938548569, -101.5914258081833879 ) ) ;
#7748=FACE_OUTER_BOUND ( 'NONE', #14206, .T. ) ;
#7750=AXIS2_PLACEMENT_3D ( 'NONE', #10343, #17967, #8870 ) ;
#7751=CARTESIAN_POINT ( 'NONE',  ( 79.64356964375001269, -32.57812499938548001, -98.40857419181659793 ) ) ;
#7754=CARTESIAN_POINT ( 'NONE',  ( 83.77821517812500929, -33.21562499938548285, -102.3871387122750889 ) ) ;
#7755=CARTESIAN_POINT ( 'NONE',  ( 79.64356964374999848, -33.51562499938548711, -99.99999999999998579 ) ) ;
#7759=CARTESIAN_POINT ( 'NONE',  ( -83.90000000000000568, -30.37500000000000355, 102.5980762113533018 ) ) ;
#7765=CARTESIAN_POINT ( 'NONE',  ( 79.64356964374999848, -30.81562499938548427, 99.99999999999998579 ) ) ;
#7769=CARTESIAN_POINT ( 'NONE',  ( 85.15643035624999868, -33.89062499938548711, 101.5914258081833879 ) ) ;
#7770=CARTESIAN_POINT ( 'NONE',  ( 85.15643035625001289, -30.70312499938548711, -99.99999999999998579 ) ) ;
#7772=CARTESIAN_POINT ( 'NONE',  ( 85.15643035625001289, -35.20312499938548711, -99.99999999999998579 ) ) ;
#7773=CARTESIAN_POINT ( 'NONE',  ( -83.77821517812500929, -33.02812499938548285, -102.3871387122750889 ) ) ;
#7776=CARTESIAN_POINT ( 'NONE',  ( 83.77821517812500929, -30.32812499938548711, 102.3871387122750889 ) ) ;
#7779=CARTESIAN_POINT ( 'NONE',  ( -82.39999999999999147, -30.59062499938548640, 103.1828516163667899 ) ) ;
#7781=ORIENTED_EDGE ( 'NONE', *, *, #17556, .T. ) ;
#7782=CARTESIAN_POINT ( 'NONE',  ( -83.90000000000000568, -30.37500000000000355, -97.40192378864668399 ) ) ;
#7783=CARTESIAN_POINT ( 'NONE',  ( 84.01447415327271528, -35.02670941564510088, -97.25687757881057394 ) ) ;
#7784=CARTESIAN_POINT ( 'NONE',  ( 79.39999999999999147, -33.80624999877097281, 98.26794919243113213 ) ) ;
#7785=CARTESIAN_POINT ( 'NONE',  ( -79.64356964375001269, -35.01562499938548711, -98.40857419181659793 ) ) ;
#7789=VERTEX_POINT ( 'NONE', #16616 ) ;
#7791=CARTESIAN_POINT ( 'NONE',  ( 79.39999999999999147, -32.90624999877096712, -101.7320508075688537 ) ) ;
#7792=CARTESIAN_POINT ( 'NONE',  ( 82.39999999999999147, -32.50312499938548427, 103.1828516163667899 ) ) ;
#7794=CARTESIAN_POINT ( 'NONE',  ( -82.40000000000000568, -30.00000000000000355, -96.99999999999998579 ) ) ;
#7795=CARTESIAN_POINT ( 'NONE',  ( 82.39999999999999147, -33.88124999877096855, -103.4641016151377499 ) ) ;
#7797=ORIENTED_EDGE ( 'NONE', *, *, #315, .T. ) ;
#7804=ORIENTED_EDGE ( 'NONE', *, *, #2775, .T. ) ;
#7805=ORIENTED_EDGE ( 'NONE', *, *, #6147, .F. ) ;
#7807=CARTESIAN_POINT ( 'NONE',  ( -81.59615242270665192, -33.67634618820330417, -103.0000000000000000 ) ) ;
#7810=CARTESIAN_POINT ( 'NONE',  ( 85.15643035624999868, -32.02817623523065294, 98.94122380911255732 ) ) ;
#7811=CARTESIAN_POINT ( 'NONE',  ( -79.39999999999999147, -34.18124999877097281, -101.7320508075688821 ) ) ;
#7819=FACE_OUTER_BOUND ( 'NONE', #18870, .T. ) ;
#7821=ADVANCED_FACE ( 'NONE', ( #1477 ), #1761, .T. ) ;
#7824=CARTESIAN_POINT ( 'NONE',  ( -83.77821517812500929, -33.81562499938548427, -102.3871387122750889 ) ) ;
#7826=ORIENTED_EDGE ( 'NONE', *, *, #18220, .T. ) ;
#7832=VERTEX_POINT ( 'NONE', #13483 ) ;
#7836=CARTESIAN_POINT ( 'NONE',  ( 79.64356964374999848, -34.86562499938548143, -99.99999999999998579 ) ) ;
#7837=CARTESIAN_POINT ( 'NONE',  ( -85.40000000000000568, -33.58124999877097139, 98.26794919243111792 ) ) ;
#7838=CARTESIAN_POINT ( 'NONE',  ( -83.09162395290293546, -32.00000000000001421, -97.24830349208643554 ) ) ;
#7840=CARTESIAN_POINT ( 'NONE',  ( 82.39999999999999147, -33.74062499938548854, -103.1828516163667899 ) ) ;
#7841=CARTESIAN_POINT ( 'NONE',  ( 82.40000000000001990, -33.88124999877096855, -103.0000000000000000 ) ) ;
#7842=CARTESIAN_POINT ( 'NONE',  ( 79.64356964375001269, -34.45312499938548711, -101.5914258081833879 ) ) ;
#7845=ADVANCED_FACE ( 'NONE', ( #6651 ), #12596, .F. ) ;
#7846=CARTESIAN_POINT ( 'NONE',  ( -84.01447415327271528, -35.02670941564510088, 97.25687757881057394 ) ) ;
#7851=CARTESIAN_POINT ( 'NONE',  ( -83.90000000000000568, -32.32500000000000284, 97.40192378864668399 ) ) ;
#7857=CARTESIAN_POINT ( 'NONE',  ( 79.64356964375001269, -30.40312499938548285, 98.40857419181659793 ) ) ;
#7858=VECTOR ( 'NONE', #17186, 1000.000000000000000 ) ;
#7862=CARTESIAN_POINT ( 'NONE',  ( 84.12306224665906029, -32.00000000000000000, 97.80849716182737552 ) ) ;
#7863=CARTESIAN_POINT ( 'NONE',  ( 82.39999999999999147, -34.19062499938548427, 96.81714838363319586 ) ) ;
#7864=CARTESIAN_POINT ( 'NONE',  ( 79.64356964374999848, -30.92812499938548498, -99.99999999999998579 ) ) ;
#7866=CARTESIAN_POINT ( 'NONE',  ( -79.64356964374999848, -34.98839802032725288, 100.4359666841262282 ) ) ;
#7867=CARTESIAN_POINT ( 'NONE',  ( -81.02178482187500208, -34.15312499938548285, -97.61286128772489690 ) ) ;
#7869=CARTESIAN_POINT ( 'NONE',  ( 85.15643035624999868, -31.56562499938548427, 98.40857419181659793 ) ) ;
#7872=AXIS2_PLACEMENT_3D ( 'NONE', #8924, #4642, #10591 ) ;
#7873=CARTESIAN_POINT ( 'NONE',  ( -85.15643035625001289, -35.20312499938548711, 99.99999999999998579 ) ) ;
#7876=CARTESIAN_POINT ( 'NONE',  ( -79.39999999999999147, -30.71250000000000568, -98.26794919243113213 ) ) ;
#7877=CARTESIAN_POINT ( 'NONE',  ( 80.90000000000000568, -34.64999999999999858, -97.40192378864668399 ) ) ;
#7878=CARTESIAN_POINT ( 'NONE',  ( 83.90000000000000568, -34.81874999877096855, -102.5980762113533018 ) ) ;
#7879=CARTESIAN_POINT ( 'NONE',  ( -81.02178482187500208, -34.90312499938548285, -102.3871387122750889 ) ) ;
#7885=CARTESIAN_POINT ( 'NONE',  ( 85.40000000000000568, -34.50000000000000000, -99.99999999999998579 ) ) ;
#7887=CARTESIAN_POINT ( 'NONE',  ( 85.40000000000000568, -34.40624999877096712, -101.7320508075688821 ) ) ;
#7890=CARTESIAN_POINT ( 'NONE',  ( 79.64356964374999848, -32.27812499938548996, -99.99999999999998579 ) ) ;
#7892=ORIENTED_EDGE ( 'NONE', *, *, #64, .T. ) ;
#7902=CARTESIAN_POINT ( 'NONE',  ( -82.40000000000000568, -33.93750000000000711, -97.00000000000000000 ) ) ;
#7904=CARTESIAN_POINT ( 'NONE',  ( 82.39999999999999147, -32.16562499938548569, 103.1828516163667899 ) ) ;
#7905=CARTESIAN_POINT ( 'NONE',  ( -83.90000000000000568, -34.06874999877096855, -102.5980762113533018 ) ) ;
#7908=( BOUNDED_CURVE ( )  B_SPLINE_CURVE ( 2, ( #3739, #9609, #18505, #9407, #827, #15667, #9311, #6686, #12630 ),
 .UNSPECIFIED., .F., .F. ) 
 B_SPLINE_CURVE_WITH_KNOTS ( ( 3, 2, 2, 2, 3 ),
 ( 0.6458333333333332593, 0.6527777777777777901, 0.6666666666666666297, 0.6805555555555555802, 0.6875000000000000000 ),
 .UNSPECIFIED. ) 
 CURVE ( )  GEOMETRIC_REPRESENTATION_ITEM ( )  RATIONAL_B_SPLINE_CURVE ( ( 0.9330127018922192983, 0.9330127018922187432, 1.000000000000000000, 0.8660254037844387076, 1.000000000000000000, 0.8660254037844387076, 1.000000000000000000, 0.9330127018922194093, 0.9330127018922194093 ) ) 
 REPRESENTATION_ITEM ( '' )  );
#7911=EDGE_CURVE ( 'NONE', #14497, #14237, #18278, .T. ) ;
#7916=ORIENTED_EDGE ( 'NONE', *, *, #11964, .T. ) ;
#7918=CARTESIAN_POINT ( 'NONE',  ( -81.02178482187500208, -34.79062499938548569, -102.3871387122750889 ) ) ;
#7919=LINE ( 'NONE', #13868, #3360 ) ;
#7920=ORIENTED_EDGE ( 'NONE', *, *, #413, .F. ) ;
#7922=DIRECTION ( 'NONE',  ( -0.000000000000000000, -1.000000000000000000, -0.000000000000000000 ) ) ;
#7923=CARTESIAN_POINT ( 'NONE',  ( 83.20384757729335945, -33.05759618943233136, -102.9999999999999858 ) ) ;
#7927=EDGE_CURVE ( 'NONE', #14213, #14240, #17845, .T. ) ;
#7930=CARTESIAN_POINT ( 'NONE',  ( 83.90000000000000568, -31.27500000000000568, -102.5980762113533018 ) ) ;
#7931=LINE ( 'NONE', #12812, #13292 ) ;
#7933=CARTESIAN_POINT ( 'NONE',  ( -79.39999999999999147, -34.25624999877096855, 101.7320508075688537 ) ) ;
#7934=DIRECTION ( 'NONE',  ( -0.000000000000000000, -0.000000000000000000, -1.000000000000000000 ) ) ;
#7936=CARTESIAN_POINT ( 'NONE',  ( 85.15643035625001289, -32.99062499938548854, -98.40857419181659793 ) ) ;
#7937=CARTESIAN_POINT ( 'NONE',  ( -82.40000000000001990, -34.16250000000000853, 97.00000000000000000 ) ) ;
#7938=CARTESIAN_POINT ( 'NONE',  ( -82.39999999999999147, -33.40312499938548285, 96.81714838363319586 ) ) ;
#7940=CARTESIAN_POINT ( 'NONE',  ( 82.39999999999999147, -33.85312499938547859, -96.81714838363319586 ) ) ;
#7941=ORIENTED_EDGE ( 'NONE', *, *, #2702, .F. ) ;
#7943=DIRECTION ( 'NONE',  ( 1.000000000000000000, 0.000000000000000000, -0.000000000000000000 ) ) ;
#7948=CARTESIAN_POINT ( 'NONE',  ( -85.40000000000000568, -32.73750000000000426, 98.26794919243111792 ) ) ;
#7949=EDGE_LOOP ( 'NONE', ( #1957, #3162, #13902, #4376, #8444, #13666, #2943, #10642, #1306, #12008, #5989, #5968, #1440, #4791, #4819, #8021, #13357 ) ) ;
#7953=CARTESIAN_POINT ( 'NONE',  ( 79.64356964375001269, -32.20312499938548001, 98.40857419181659793 ) ) ;
#7954=CARTESIAN_POINT ( 'NONE',  ( 84.53225329756206463, -31.99999999999999289, -98.24409948398914594 ) ) ;
#7956=CARTESIAN_POINT ( 'NONE',  ( -85.15643035625001289, -32.05312499938548854, -99.99999999999998579 ) ) ;
#7957=CARTESIAN_POINT ( 'NONE',  ( 79.64356964375001269, -34.04062499938549280, 101.5914258081833879 ) ) ;
#7958=CARTESIAN_POINT ( 'NONE',  ( 85.15643035625001289, -32.50312499938548427, -99.99999999999998579 ) ) ;
#7961=CARTESIAN_POINT ( 'NONE',  ( -81.02178482187500208, -33.10312499938548569, 97.61286128772489690 ) ) ;
#7962=CARTESIAN_POINT ( 'NONE',  ( -82.39999999999999147, -34.64062499938548711, -96.81714838363319586 ) ) ;
#7963=ORIENTED_EDGE ( 'NONE', *, *, #15183, .T. ) ;
#7964=CARTESIAN_POINT ( 'NONE',  ( 85.15643035624999868, -33.44062499938548427, 101.5914258081833879 ) ) ;
#7967=CARTESIAN_POINT ( 'NONE',  ( -82.39999999999999147, -31.15312499938548640, 96.81714838363319586 ) ) ;
#7968=CARTESIAN_POINT ( 'NONE',  ( -85.15643035624999868, -34.26562499938548711, 101.5914258081833879 ) ) ;
#7969=ORIENTED_EDGE ( 'NONE', *, *, #5907, .F. ) ;
#7970=CARTESIAN_POINT ( 'NONE',  ( -82.39999999999999147, -33.03750000000000142, -96.53589838486223584 ) ) ;
#7971=( BOUNDED_CURVE ( )  B_SPLINE_CURVE ( 2, ( #9447, #481, #10916, #12291, #5262, #18446, #4874, #2022, #6624 ),
 .UNSPECIFIED., .F., .F. ) 
 B_SPLINE_CURVE_WITH_KNOTS ( ( 3, 2, 2, 2, 3 ),
 ( 0.7291666666666666297, 0.7361111111111111605, 0.7500000000000000000, 0.7638888888888888395, 0.7708333333333331483 ),
 .UNSPECIFIED. ) 
 CURVE ( )  GEOMETRIC_REPRESENTATION_ITEM ( )  RATIONAL_B_SPLINE_CURVE ( ( 0.9330127018922192983, 0.9330127018922187432, 1.000000000000000000, 0.8660254037844387076, 1.000000000000000000, 0.8660254037844387076, 1.000000000000000000, 0.9330127018922209636, 0.9330127018922194093 ) ) 
 REPRESENTATION_ITEM ( '' )  );
#7979=CYLINDRICAL_SURFACE ( 'NONE', #9929, 3.000000000000002665 ) ;
#7981=CARTESIAN_POINT ( 'NONE',  ( -85.40000000000000568, -33.54374999877096286, -99.99999999999998579 ) ) ;
#7982=DIRECTION ( 'NONE',  ( -0.000000000000000000, -0.000000000000000000, -1.000000000000000000 ) ) ;
#7985=CARTESIAN_POINT ( 'NONE',  ( 84.69813954184694182, -35.39427337414329600, -98.07164457472185859 ) ) ;
#7995=ORIENTED_EDGE ( 'NONE', *, *, #18683, .T. ) ;
#7996=CARTESIAN_POINT ( 'NONE',  ( -85.15643035625001289, -31.49062499938548498, -99.99999999999998579 ) ) ;
#7998=DIRECTION ( 'NONE',  ( 0.000000000000000000, -1.000000000000000000, 0.000000000000000000 ) ) ;
#8000=CARTESIAN_POINT ( 'NONE',  ( 83.77821517812500929, -32.12812499938548427, 102.3871387122750889 ) ) ;
#8002=CARTESIAN_POINT ( 'NONE',  ( -80.90000000000000568, -34.29374999877096997, -97.40192378864668399 ) ) ;
#8003=CARTESIAN_POINT ( 'NONE',  ( -82.17437583783126342, -34.99999999999998579, 97.01974242045221786 ) ) ;
#8006=CARTESIAN_POINT ( 'NONE',  ( 84.06832524826556607, -34.99999999999999289, -102.2567273996575210 ) ) ;
#8010=ORIENTED_EDGE ( 'NONE', *, *, #9607, .F. ) ;
#8011=DIRECTION ( 'NONE',  ( 1.000000000000000000, 3.548298019043479384E-15, 0.000000000000000000 ) ) ;
#8015=DIRECTION ( 'NONE',  ( 0.000000000000000000, 0.000000000000000000, -1.000000000000000000 ) ) ;
#8020=ORIENTED_EDGE ( 'NONE', *, *, #13997, .F. ) ;
#8021=ORIENTED_EDGE ( 'NONE', *, *, #11281, .F. ) ;
#8024=CARTESIAN_POINT ( 'NONE',  ( 85.40000000000000568, -30.03750000000000497, -98.26794919243111792 ) ) ;
#8027=CARTESIAN_POINT ( 'NONE',  ( -79.39999999999999147, -35.08124999877097139, 98.26794919243110371 ) ) ;
#8029=CARTESIAN_POINT ( 'NONE',  ( -83.20384757729335945, -32.28615380933863577, -103.0000000000000000 ) ) ;
#8031=CARTESIAN_POINT ( 'NONE',  ( 83.77821517812500929, -33.47812499938548569, -97.61286128772489690 ) ) ;
#8033=CARTESIAN_POINT ( 'NONE',  ( -81.02178482187500208, -34.04062499938548569, 102.3871387122750889 ) ) ;
#8035=CARTESIAN_POINT ( 'NONE',  ( 79.64356964375001269, -33.47812499938547859, -98.40857419181659793 ) ) ;
#8038=CARTESIAN_POINT ( 'NONE',  ( -79.39999999999999147, -34.23750000000000426, 98.26794919243110371 ) ) ;
#8044=CARTESIAN_POINT ( 'NONE',  ( -82.39999999999999147, -32.13749999999999574, 103.4641016151377499 ) ) ;
#8046=ORIENTED_EDGE ( 'NONE', *, *, #11635, .T. ) ;
#8049=CARTESIAN_POINT ( 'NONE',  ( 80.07894310789828296, -34.99999999999997868, 98.50261820439547478 ) ) ;
#8050=CARTESIAN_POINT ( 'NONE',  ( 85.15643035624999868, -33.32812499938548001, 101.5914258081833879 ) ) ;
#8052=AXIS2_PLACEMENT_3D ( 'NONE', #15359, #7934, #5018 ) ;
#8054=( BOUNDED_CURVE ( )  B_SPLINE_CURVE ( 2, ( #5590, #16228, #8594, #14945, #1466, #8881, #16319, #1570, #1280 ),
 .UNSPECIFIED., .F., .F. ) 
 B_SPLINE_CURVE_WITH_KNOTS ( ( 3, 2, 2, 2, 3 ),
 ( 0.7708333333333332593, 0.7777777777777777901, 0.7916666666666666297, 0.8055555555555555802, 0.8125000000000000000 ),
 .UNSPECIFIED. ) 
 CURVE ( )  GEOMETRIC_REPRESENTATION_ITEM ( )  RATIONAL_B_SPLINE_CURVE ( ( 0.9330127018922192983, 0.9330127018922187432, 1.000000000000000000, 0.8660254037844387076, 1.000000000000000000, 0.8660254037844387076, 1.000000000000000000, 0.9330127018922194093, 0.9330127018922194093 ) ) 
 REPRESENTATION_ITEM ( '' )  );
#8055=EDGE_CURVE ( 'NONE', #15743, #15327, #15510, .T. ) ;
#8057=CARTESIAN_POINT ( 'NONE',  ( 81.45486068924893175, -32.00000000000000000, 97.24663084804296886 ) ) ;
#8058=CARTESIAN_POINT ( 'NONE',  ( 85.15643035624999868, -33.32812499938548001, 101.5914258081833879 ) ) ;
#8059=ADVANCED_FACE ( 'NONE', ( #10432 ), #18065, .F. ) ;
#8060=CARTESIAN_POINT ( 'NONE',  ( 81.02178482187500208, -31.90312499938548996, -102.3871387122750889 ) ) ;
#8062=CARTESIAN_POINT ( 'NONE',  ( -79.64356964374998427, -34.11562499938548854, 101.5914258081833879 ) ) ;
#8063=CARTESIAN_POINT ( 'NONE',  ( -79.64356964375001269, -34.04062499938549280, -101.5914258081833879 ) ) ;
#8065=ORIENTED_EDGE ( 'NONE', *, *, #5185, .T. ) ;
#8066=CARTESIAN_POINT ( 'NONE',  ( 79.64356964375001269, -33.14062499938548711, 101.5914258081833879 ) ) ;
#8069=CARTESIAN_POINT ( 'NONE',  ( -79.64356964374999848, -31.71562499938548285, 99.99999999999998579 ) ) ;
#8070=CARTESIAN_POINT ( 'NONE',  ( -83.77821517812500929, -33.77812499938548285, 102.3871387122750889 ) ) ;
#8071=CYLINDRICAL_SURFACE ( 'NONE', #14292, 3.000000000000002665 ) ;
#8072=ORIENTED_EDGE ( 'NONE', *, *, #15488, .T. ) ;
#8073=CARTESIAN_POINT ( 'NONE',  ( -82.39999999999999147, -33.93750000000000000, -96.53589838486223584 ) ) ;
#8074=CARTESIAN_POINT ( 'NONE',  ( 81.59615242270662350, -32.83259618943233704, -96.99999999999998579 ) ) ;
#8075=CARTESIAN_POINT ( 'NONE',  ( 82.85024983566745505, -34.99999999999999289, -97.02690897175904183 ) ) ;
#8077=DIRECTION ( 'NONE',  ( 0.000000000000000000, 0.000000000000000000, 1.000000000000000000 ) ) ;
#8082=FACE_OUTER_BOUND ( 'NONE', #15843, .T. ) ;
#8083=CARTESIAN_POINT ( 'NONE',  ( 82.40000000000001990, -32.13750000000000284, 97.00000000000000000 ) ) ;
#8084=CARTESIAN_POINT ( 'NONE',  ( 81.02178482187500208, -34.79062499938548569, 102.3871387122750889 ) ) ;
#8088=CARTESIAN_POINT ( 'NONE',  ( 82.39999999999999147, -30.59062499938548640, -103.1828516163667899 ) ) ;
#8090=ORIENTED_EDGE ( 'NONE', *, *, #1401, .F. ) ;
#8091=CARTESIAN_POINT ( 'NONE',  ( 80.90000000000000568, -31.59374999877097423, 97.40192378864668399 ) ) ;
#8093=EDGE_CURVE ( 'NONE', #800, #2879, #7518, .T. ) ;
#8095=( BOUNDED_CURVE ( )  B_SPLINE_CURVE ( 2, ( #18736, #5356, #18635, #18925, #11494, #4069, #1138, #5258, #11204 ),
 .UNSPECIFIED., .F., .F. ) 
 B_SPLINE_CURVE_WITH_KNOTS ( ( 3, 2, 2, 2, 3 ),
 ( 0.8125000000000001110, 0.8194444444444444198, 0.8333333333333333703, 0.8472222222222222099, 0.8530683953269213582 ),
 .UNSPECIFIED. ) 
 CURVE ( )  GEOMETRIC_REPRESENTATION_ITEM ( )  RATIONAL_B_SPLINE_CURVE ( ( 0.9330127018922194093, 0.9330127018922204085, 1.000000000000000000, 0.8660254037844387076, 1.000000000000000000, 0.8660254037844387076, 1.000000000000000000, 0.9436068149601996025, 0.9346881722405915305 ) ) 
 REPRESENTATION_ITEM ( '' )  );
#8100=CARTESIAN_POINT ( 'NONE',  ( -83.77821517812500929, -30.96562499938548640, -97.61286128772489690 ) ) ;
#8102=ORIENTED_EDGE ( 'NONE', *, *, #1534, .T. ) ;
#8103=CARTESIAN_POINT ( 'NONE',  ( 79.64356964374998427, -33.14062499938548711, 101.5914258081833879 ) ) ;
#8104=CARTESIAN_POINT ( 'NONE',  ( -79.39999999999999147, -32.86874999877097281, -99.99999999999998579 ) ) ;
#8105=CARTESIAN_POINT ( 'NONE',  ( 79.39999999999999147, -32.96250000000000568, 98.26794919243113213 ) ) ;
#8106=CARTESIAN_POINT ( 'NONE',  ( -85.15643035625001289, -35.20312499938548711, 99.99999999999998579 ) ) ;
#8109=CARTESIAN_POINT ( 'NONE',  ( 85.31192385480649421, -34.99999999999999289, -99.60674545263997004 ) ) ;
#8110=CARTESIAN_POINT ( 'NONE',  ( 82.40000000000000568, -30.00000000000000355, -99.99999999999998579 ) ) ;
#8114=CARTESIAN_POINT ( 'NONE',  ( 83.77821517812500929, -32.01562499938548001, -97.61286128772489690 ) ) ;
#8115=CARTESIAN_POINT ( 'NONE',  ( -82.39999999999999147, -34.75312499938549138, -103.1828516163667899 ) ) ;
#8117=ORIENTED_EDGE ( 'NONE', *, *, #2244, .T. ) ;
#8118=LINE ( 'NONE', #708, #1784 ) ;
#8120=CARTESIAN_POINT ( 'NONE',  ( 82.40000000000001990, -32.13750000000000284, 97.00000000000000000 ) ) ;
#8126=CARTESIAN_POINT ( 'NONE',  ( -79.39999999999999147, -32.02500000000000568, -99.99999999999998579 ) ) ;
#8127=CARTESIAN_POINT ( 'NONE',  ( 83.25523545990762386, -35.19352049914630953, -96.73097394877602540 ) ) ;
#8129=CARTESIAN_POINT ( 'NONE',  ( -79.39999999999999147, -33.76874999877097139, 99.99999999999998579 ) ) ;
#8131=LINE ( 'NONE', #14083, #13354 ) ;
#8132=CARTESIAN_POINT ( 'NONE',  ( 79.39999999999999147, -33.35624999877096997, 98.26794919243113213 ) ) ;
#8133=CARTESIAN_POINT ( 'NONE',  ( 79.64356964374999848, -32.27812499938548996, -99.99999999999998579 ) ) ;
#8134=CARTESIAN_POINT ( 'NONE',  ( -99.99999999999998579, -32.00000000000000000, -150.0000000000000000 ) ) ;
#8135=CARTESIAN_POINT ( 'NONE',  ( -81.02178482187500208, -34.34062499938548285, 97.61286128772489690 ) ) ;
#8136=CARTESIAN_POINT ( 'NONE',  ( 83.77821517812500929, -35.01562499938548711, -102.3871387122750889 ) ) ;
#8139=CARTESIAN_POINT ( 'NONE',  ( -82.39999999999999147, -34.16250000000000142, 96.53589838486223584 ) ) ;
#8144=CARTESIAN_POINT ( 'NONE',  ( -82.39999999999999147, -32.36250000000000426, 96.53589838486223584 ) ) ;
#8146=CARTESIAN_POINT ( 'NONE',  ( -83.20395887649183919, -35.00000000000001421, -97.36341917746362640 ) ) ;
#8149=CARTESIAN_POINT ( 'NONE',  ( 79.64356964375001269, -32.12812499938548427, 101.5914258081833879 ) ) ;
#8151=CARTESIAN_POINT ( 'NONE',  ( 82.40000000000001990, -32.53124999877097423, -103.0000000000000000 ) ) ;
#8153=CARTESIAN_POINT ( 'NONE',  ( 81.68701737470171054, -32.00000000000000000, 97.18802777794500969 ) ) ;
#8154=CARTESIAN_POINT ( 'NONE',  ( 82.39999999999999147, -31.60312499938548569, 103.1828516163667899 ) ) ;
#8155=EDGE_CURVE ( 'NONE', #18433, #729, #2216, .T. ) ;
#8158=CARTESIAN_POINT ( 'NONE',  ( 81.02178482187500208, -31.00312499938548783, -102.3871387122750889 ) ) ;
#8160=CARTESIAN_POINT ( 'NONE',  ( -82.39999999999999147, -33.96562499938548285, 96.81714838363319586 ) ) ;
#8161=CARTESIAN_POINT ( 'NONE',  ( -85.15643035624999868, -31.45312499938548356, -98.40857419181659793 ) ) ;
#8163=CARTESIAN_POINT ( 'NONE',  ( 83.77821517812500929, -33.47812499938548569, 102.3871387122750889 ) ) ;
#8165=CARTESIAN_POINT ( 'NONE',  ( -81.02178482187500208, -30.89062499938548711, 102.3871387122750889 ) ) ;
#8166=CARTESIAN_POINT ( 'NONE',  ( -79.64356964375001269, -33.21562499938548996, 101.5914258081833879 ) ) ;
#8169=CARTESIAN_POINT ( 'NONE',  ( -83.90000000000000568, -34.57500000000000284, -102.5980762113533018 ) ) ;
#8170=EDGE_CURVE ( 'NONE', #5045, #10401, #10881, .T. ) ;
#8172=CARTESIAN_POINT ( 'NONE',  ( 83.04276107155152431, -34.99999999999999289, -97.06242906295997841 ) ) ;
#8175=EDGE_CURVE ( 'NONE', #7020, #13374, #383, .T. ) ;
#8180=CARTESIAN_POINT ( 'NONE',  ( -82.40000000000001990, -33.26250000000000284, 97.00000000000000000 ) ) ;
#8181=CARTESIAN_POINT ( 'NONE',  ( 81.02178482187500208, -31.00312499938548783, 97.61286128772489690 ) ) ;
#8182=CARTESIAN_POINT ( 'NONE',  ( 83.20384757729337366, -32.79240381056766296, -97.00000000000000000 ) ) ;
#8183=CARTESIAN_POINT ( 'NONE',  ( 79.64356964374999848, -31.82812499938548356, -99.99999999999998579 ) ) ;
#8184=LINE ( 'NONE', #11009, #18649 ) ;
#8185=AXIS2_PLACEMENT_3D ( 'NONE', #14750, #13283, #5874 ) ;
#8191=B_SPLINE_CURVE_WITH_KNOTS ( 'NONE', 3,
 ( #3561, #3460, #18229, #18326, #9419, #5133, #2195, #8057, #8153, #18418, #1900, #12641, #9717, #741, #18615, #7862, #4943, #838 ),
 .UNSPECIFIED., .F., .F.,
 ( 4, 2, 2, 2, 2, 2, 2, 2, 4 ),
 ( 0.000000000000000000, 0.0007106627595359841631, 0.001421325519071968326, 0.002131988278607952272, 0.002842651038143936652, 0.003553313797679921032, 0.004263976557215904545, 0.004974639316751888925, 0.005685302076287873305 ),
 .UNSPECIFIED. ) ;
#8196=CARTESIAN_POINT ( 'NONE',  ( -83.77821517812500929, -31.56562499938548427, -102.3871387122750889 ) ) ;
#8198=ORIENTED_EDGE ( 'NONE', *, *, #9468, .F. ) ;
#8199=CARTESIAN_POINT ( 'NONE',  ( 81.02178482187500208, -33.70312499938548711, 97.61286128772489690 ) ) ;
#8200=CARTESIAN_POINT ( 'NONE',  ( -85.40000000000000568, -33.99374999877097281, -99.99999999999998579 ) ) ;
#8201=CARTESIAN_POINT ( 'NONE',  ( 80.90000000000000568, -33.30000000000000426, 102.5980762113533018 ) ) ;
#8204=EDGE_CURVE ( 'NONE', #2256, #5463, #9513, .T. ) ;
#8207=CARTESIAN_POINT ( 'NONE',  ( 84.25709831969352592, -34.99999999999999289, -102.1174602701827752 ) ) ;
#8209=DIRECTION ( 'NONE',  ( 1.000000000000000000, -2.001604010742470847E-15, 0.000000000000000000 ) ) ;
#8213=CARTESIAN_POINT ( 'NONE',  ( 83.77821517812500929, -33.81562499938548427, -97.61286128772489690 ) ) ;
#8218=VECTOR ( 'NONE', #17742, 1000.000000000000000 ) ;
#8219=ORIENTED_EDGE ( 'NONE', *, *, #5596, .T. ) ;
#8225=ORIENTED_EDGE ( 'NONE', *, *, #16083, .F. ) ;
#8227=CARTESIAN_POINT ( 'NONE',  ( 82.39999999999999147, -33.71249999999999858, -96.53589838486223584 ) ) ;
#8229=CARTESIAN_POINT ( 'NONE',  ( -79.39999999999999147, -34.18124999877097281, 98.26794919243110371 ) ) ;
#8233=CARTESIAN_POINT ( 'NONE',  ( 79.64356964374999848, -34.98839802032723867, -100.4359666841259440 ) ) ;
#8235=CARTESIAN_POINT ( 'NONE',  ( -85.15643035625001289, -32.84062499938548285, 99.99999999999998579 ) ) ;
#8236=FACE_OUTER_BOUND ( 'NONE', #17718, .T. ) ;
#8238=CARTESIAN_POINT ( 'NONE',  ( -83.90000000000000568, -34.42500000000000426, 102.5980762113533018 ) ) ;
#8243=ORIENTED_EDGE ( 'NONE', *, *, #17556, .F. ) ;
#8246=CARTESIAN_POINT ( 'NONE',  ( 82.39999999999999147, -33.62812499938549138, 96.81714838363319586 ) ) ;
#8247=EDGE_CURVE ( 'NONE', #14672, #4832, #11518, .T. ) ;
#8252=CARTESIAN_POINT ( 'NONE',  ( 79.64356964375001269, -31.22812499938548925, 101.5914258081833879 ) ) ;
#8253=CARTESIAN_POINT ( 'NONE',  ( 79.64356964375001269, -34.49062499938548854, -98.40857419181659793 ) ) ;
#8257=CARTESIAN_POINT ( 'NONE',  ( 81.02178482187500208, -33.70312499938548711, 97.61286128772489690 ) ) ;
#8262=CARTESIAN_POINT ( 'NONE',  ( -83.77821517812500929, -33.92812499938548854, 97.61286128772489690 ) ) ;
#8264=ORIENTED_EDGE ( 'NONE', *, *, #6247, .T. ) ;
#8265=CARTESIAN_POINT ( 'NONE',  ( -80.90000000000000568, -33.30000000000000426, -102.5980762113533018 ) ) ;
#8270=CARTESIAN_POINT ( 'NONE',  ( -84.57144699476174310, -35.00000000000000000, 97.92073041325134852 ) ) ;
#8273=CARTESIAN_POINT ( 'NONE',  ( 83.77821517812500929, -30.62812499938548783, 97.61286128772489690 ) ) ;
#8275=CARTESIAN_POINT ( 'NONE',  ( -82.39999999999999147, -32.81250000000000000, -103.0000000000000000 ) ) ;
#8276=CARTESIAN_POINT ( 'NONE',  ( 81.02178482187500208, -32.20312499938548711, -97.61286128772489690 ) ) ;
#8277=CARTESIAN_POINT ( 'NONE',  ( -82.40000000000000568, -30.00000000000000355, -96.99999999999998579 ) ) ;
#8278=CIRCLE ( 'NONE', #17335, 2.199999999999993516 ) ;
#8280=ORIENTED_EDGE ( 'NONE', *, *, #1156, .T. ) ;
#8281=CARTESIAN_POINT ( 'NONE',  ( 83.90000000000000568, -31.21874999877097068, 97.40192378864668399 ) ) ;
#8285=CARTESIAN_POINT ( 'NONE',  ( -83.43443729601585801, -35.00000000000000000, -97.42249611015782307 ) ) ;
#8287=CARTESIAN_POINT ( 'NONE',  ( -81.02178482187500208, -30.74062499938548498, -102.3871387122750889 ) ) ;
#8289=EDGE_CURVE ( 'NONE', #12671, #5588, #2160, .T. ) ;
#8290=ORIENTED_EDGE ( 'NONE', *, *, #1284, .F. ) ;
#8291=CARTESIAN_POINT ( 'NONE',  ( 82.39999999999999147, -34.41562499938548569, 103.1828516163667899 ) ) ;
#8292=CARTESIAN_POINT ( 'NONE',  ( -85.15643035624999868, -31.11562499938548854, -98.40857419181659793 ) ) ;
#8294=CARTESIAN_POINT ( 'NONE',  ( 83.90000000000000568, -33.97500000000000853, 97.40192378864668399 ) ) ;
#8300=DIRECTION ( 'NONE',  ( 0.000000000000000000, -1.000000000000000000, 0.000000000000000000 ) ) ;
#8302=VERTEX_POINT ( 'NONE', #9740 ) ;
#8303=CARTESIAN_POINT ( 'NONE',  ( 85.15643035625001289, -32.84062499938548285, -99.99999999999998579 ) ) ;
#8307=AXIS2_PLACEMENT_3D ( 'NONE', #6873, #1007, #8605 ) ;
#8316=CARTESIAN_POINT ( 'NONE',  ( 80.90000000000000568, -31.94999999999999929, -97.40192378864668399 ) ) ;
#8318=CARTESIAN_POINT ( 'NONE',  ( -81.02178482187500208, -31.45312499938549067, 102.3871387122750889 ) ) ;
#8323=CARTESIAN_POINT ( 'NONE',  ( -69.99999999999998579, -32.00000000000000000, -150.0000000000000000 ) ) ;
#8324=CARTESIAN_POINT ( 'NONE',  ( -82.39999999999999147, -32.05312499938548854, 96.81714838363319586 ) ) ;
#8326=CARTESIAN_POINT ( 'NONE',  ( -99.99999999999998579, 0.000000000000000000, 150.0000000000000000 ) ) ;
#8327=ORIENTED_EDGE ( 'NONE', *, *, #6247, .F. ) ;
#8328=CARTESIAN_POINT ( 'NONE',  ( 79.39999999999999147, -32.96250000000000568, 98.26794919243113213 ) ) ;
#8330=CARTESIAN_POINT ( 'NONE',  ( 85.40000000000000568, -34.85624999877096997, 98.26794919243111792 ) ) ;
#8335=ADVANCED_FACE ( 'NONE', ( #5641 ), #859, .F. ) ;
#8338=CARTESIAN_POINT ( 'NONE',  ( -83.90000000000000568, -30.46874999877096712, 97.40192378864668399 ) ) ;
#8339=CARTESIAN_POINT ( 'NONE',  ( 79.64356964374999848, -32.16562499938548569, 99.99999999999998579 ) ) ;
#8341=CARTESIAN_POINT ( 'NONE',  ( 82.40000000000000568, -31.99999999999999289, 99.99999999999998579 ) ) ;
#8345=CARTESIAN_POINT ( 'NONE',  ( -81.02178482187500208, -33.25312499938548427, -97.61286128772489690 ) ) ;
#8346=CARTESIAN_POINT ( 'NONE',  ( 82.39999999999999147, -32.05312499938548854, 103.1828516163667899 ) ) ;
#8348=CARTESIAN_POINT ( 'NONE',  ( 82.39999999999999147, -33.96562499938548285, -96.81714838363319586 ) ) ;
#8350=CARTESIAN_POINT ( 'NONE',  ( -85.15643035625001289, -33.29062499938547859, 99.99999999999998579 ) ) ;
#8351=CARTESIAN_POINT ( 'NONE',  ( 85.15643035624999868, -30.17812499938548498, -98.40857419181659793 ) ) ;
#8353=CARTESIAN_POINT ( 'NONE',  ( 79.64356964375001269, -34.56562499938549138, 98.40857419181659793 ) ) ;
#8356=CARTESIAN_POINT ( 'NONE',  ( -79.64356964375001269, -31.67812499938548143, 98.40857419181659793 ) ) ;
#8357=CARTESIAN_POINT ( 'NONE',  ( -79.64356964375001269, -31.30312499938548854, 101.5914258081833879 ) ) ;
#8360=CARTESIAN_POINT ( 'NONE',  ( -85.40000000000000568, -32.70000000000000284, -99.99999999999998579 ) ) ;
#8369=CARTESIAN_POINT ( 'NONE',  ( -82.40000000000001990, -32.53124999877097423, -97.00000000000000000 ) ) ;
#8373=CARTESIAN_POINT ( 'NONE',  ( 82.39999999999999147, -33.06562499938548427, -96.81714838363319586 ) ) ;
#8375=CARTESIAN_POINT ( 'NONE',  ( -85.40000000000000568, -33.13124999877096855, 98.26794919243111792 ) ) ;
#8382=CARTESIAN_POINT ( 'NONE',  ( -85.10336890117801545, -35.00000000000000711, -99.00607337841718447 ) ) ;
#8384=CARTESIAN_POINT ( 'NONE',  ( -79.64356964374999848, -31.71562499938548285, -99.99999999999998579 ) ) ;
#8385=CARTESIAN_POINT ( 'NONE',  ( -82.40000000000000568, -30.00000000000000355, -103.0000000000000000 ) ) ;
#8387=CARTESIAN_POINT ( 'NONE',  ( 81.02178482187500208, -33.55312499938548854, 102.3871387122750889 ) ) ;
#8388=CARTESIAN_POINT ( 'NONE',  ( -83.77821517812500929, -31.97812499938548925, -97.61286128772489690 ) ) ;
#8389=CARTESIAN_POINT ( 'NONE',  ( -85.40000000000000568, -30.43124999877096926, -101.7320508075688679 ) ) ;
#8394=CARTESIAN_POINT ( 'NONE',  ( -80.90000000000000568, -34.14374999877097139, -102.5980762113533018 ) ) ;
#8397=EDGE_CURVE ( 'NONE', #6950, #518, #15799, .T. ) ;
#8399=CARTESIAN_POINT ( 'NONE',  ( 79.64356964374998427, -33.02812499938548285, -98.40857419181659793 ) ) ;
#8406=ORIENTED_EDGE ( 'NONE', *, *, #9187, .T. ) ;
#8410=CARTESIAN_POINT ( 'NONE',  ( -80.90000000000000568, -32.10000000000000142, -97.40192378864668399 ) ) ;
#8411=CARTESIAN_POINT ( 'NONE',  ( 83.90000000000000568, -33.52499999999999858, -102.5980762113533018 ) ) ;
#8414=CARTESIAN_POINT ( 'NONE',  ( -83.77821517812500929, -31.97812499938548925, 102.3871387122750889 ) ) ;
#8416=CARTESIAN_POINT ( 'NONE',  ( -82.40000000000000568, -34.61250000000001137, -102.9999999999999858 ) ) ;
#8418=CARTESIAN_POINT ( 'NONE',  ( 94.79999999999995453, -32.00000000000000000, -150.0000000000000000 ) ) ;
#8419=CARTESIAN_POINT ( 'NONE',  ( 84.85538848574883275, -34.99999999999999289, 101.7224313860079263 ) ) ;
#8423=LINE ( 'NONE', #1098, #6808 ) ;
#8428=EDGE_CURVE ( 'NONE', #9376, #10447, #16266, .T. ) ;
#8432=CARTESIAN_POINT ( 'NONE',  ( -85.40000000000000568, -30.39374999877097139, 99.99999999999998579 ) ) ;
#8433=CARTESIAN_POINT ( 'NONE',  ( 81.02178482187500208, -34.34062499938548285, 102.3871387122750889 ) ) ;
#8434=DIRECTION ( 'NONE',  ( -0.000000000000000000, -1.000000000000000000, -0.000000000000000000 ) ) ;
#8438=CARTESIAN_POINT ( 'NONE',  ( -85.15643035625001289, -34.26562499938548711, -98.40857419181659793 ) ) ;
#8439=CARTESIAN_POINT ( 'NONE',  ( 79.64356964375001269, -31.30312499938548854, 98.40857419181659793 ) ) ;
#8440=CARTESIAN_POINT ( 'NONE',  ( 81.02178482187500208, -34.45312499938548711, -97.61286128772489690 ) ) ;
#8442=CARTESIAN_POINT ( 'NONE',  ( -85.15643035625001289, -33.25312499938548427, 101.5914258081833879 ) ) ;
#8443=CARTESIAN_POINT ( 'NONE',  ( 85.15643035625001289, -31.49062499938548498, -99.99999999999998579 ) ) ;
#8444=ORIENTED_EDGE ( 'NONE', *, *, #8247, .F. ) ;
#8445=CARTESIAN_POINT ( 'NONE',  ( 83.77821517812500929, -34.82812499938548711, 102.3871387122750889 ) ) ;
#8446=CARTESIAN_POINT ( 'NONE',  ( -82.40000000000000568, -34.38749999999999574, -96.99999999999998579 ) ) ;
#8447=ADVANCED_FACE ( 'NONE', ( #13694 ), #15062, .T. ) ;
#8449=CARTESIAN_POINT ( 'NONE',  ( -79.64356964374999848, -32.16562499938548569, 99.99999999999998579 ) ) ;
#8450=CARTESIAN_POINT ( 'NONE',  ( -82.39999999999999147, -31.82812499938548356, 103.1828516163667899 ) ) ;
#8456=DIRECTION ( 'NONE',  ( 0.000000000000000000, -1.000000000000000000, 0.000000000000000000 ) ) ;
#8461=CARTESIAN_POINT ( 'NONE',  ( -83.90000000000000568, -32.56874999877096855, -97.40192378864668399 ) ) ;
#8462=CARTESIAN_POINT ( 'NONE',  ( 81.02178482187500208, -33.70312499938548711, -102.3871387122750889 ) ) ;
#8465=CARTESIAN_POINT ( 'NONE',  ( 82.39999999999999147, -33.43124999877097281, 96.53589838486223584 ) ) ;
#8470=EDGE_LOOP ( 'NONE', ( #7555, #11939, #15269, #1469 ) ) ;
#8471=CARTESIAN_POINT ( 'NONE',  ( -85.15643035624999868, -34.15312499938548285, -98.40857419181659793 ) ) ;
#8472=DIRECTION ( 'NONE',  ( -1.000000000000000000, 0.000000000000000000, 0.000000000000000000 ) ) ;
#8474=CARTESIAN_POINT ( 'NONE',  ( 81.02178482187500208, -34.15312499938548285, 97.61286128772489690 ) ) ;
#8475=CARTESIAN_POINT ( 'NONE',  ( -82.39999999999999147, -31.94062499938548427, -96.81714838363319586 ) ) ;
#8476=CARTESIAN_POINT ( 'NONE',  ( 82.39999999999999147, -33.26250000000000284, 103.4641016151377499 ) ) ;
#8477=CARTESIAN_POINT ( 'NONE',  ( 82.40000000000001990, -32.08124999877097139, 97.00000000000000000 ) ) ;
#8480=CARTESIAN_POINT ( 'NONE',  ( -81.02178482187500208, -33.44062499938548427, -102.3871387122750889 ) ) ;
#8482=( BOUNDED_CURVE ( )  B_SPLINE_CURVE ( 2, ( #6199, #4829, #13510, #1980, #16449 ),
 .UNSPECIFIED., .F., .F. ) 
 B_SPLINE_CURVE_WITH_KNOTS ( ( 3, 2, 3 ),
 ( 0.2975293541897524041, 0.3055555555555555802, 0.3125000000000001665 ),
 .UNSPECIFIED. ) 
 CURVE ( )  GEOMETRIC_REPRESENTATION_ITEM ( )  RATIONAL_B_SPLINE_CURVE ( ( 0.9346381638529799307, 0.9225778897267649103, 1.000000000000000000, 0.9330127018922177440, 0.9330127018922194093 ) ) 
 REPRESENTATION_ITEM ( '' )  );
#8483=VECTOR ( 'NONE', #4019, 1000.000000000000000 ) ;
#8484=DIRECTION ( 'NONE',  ( -1.000000000000000000, 0.000000000000000000, 0.000000000000000000 ) ) ;
#8485=CARTESIAN_POINT ( 'NONE',  ( 83.90000000000000568, -32.71874999877096712, -97.40192378864668399 ) ) ;
#8487=ORIENTED_EDGE ( 'NONE', *, *, #16270, .F. ) ;
#8488=CARTESIAN_POINT ( 'NONE',  ( 83.77821517812500929, -34.71562499938548285, -97.61286128772489690 ) ) ;
#8497=AXIS2_PLACEMENT_3D ( 'NONE', #11856, #7364, #7462 ) ;
#8500=CARTESIAN_POINT ( 'NONE',  ( 83.90000000000000568, -33.07500000000000284, -102.5980762113533018 ) ) ;
#8504=CARTESIAN_POINT ( 'NONE',  ( -81.02178482187500208, -30.85312499938548569, 97.61286128772489690 ) ) ;
#8508=CARTESIAN_POINT ( 'NONE',  ( 83.77821517812500929, -34.82812499938548711, -97.61286128772489690 ) ) ;
#8509=CARTESIAN_POINT ( 'NONE',  ( 80.32125193361331128, -34.99999999999999289, 102.0234471769926472 ) ) ;
#8510=LINE ( 'NONE', #5691, #9606 ) ;
#8512=DIRECTION ( 'NONE',  ( 0.000000000000000000, -1.000000000000000000, 0.000000000000000000 ) ) ;
#8514=CARTESIAN_POINT ( 'NONE',  ( -79.64356964375001269, -34.94062499938549138, -101.5914258081833879 ) ) ;
#8516=LINE ( 'NONE', #17224, #13026 ) ;
#8517=EDGE_CURVE ( 'NONE', #5861, #9248, #18511, .T. ) ;
#8518=CARTESIAN_POINT ( 'NONE',  ( -82.40000000000000568, -30.00000000000000355, -99.99999999999998579 ) ) ;
#8519=CARTESIAN_POINT ( 'NONE',  ( -83.90000000000000568, -34.87500000000000000, -97.40192378864668399 ) ) ;
#8521=DIRECTION ( 'NONE',  ( 1.000000000000000000, -0.000000000000000000, -2.407412430484046130E-31 ) ) ;
#8522=ADVANCED_FACE ( 'NONE', ( #15350 ), #10951, .F. ) ;
#8527=CARTESIAN_POINT ( 'NONE',  ( -79.39999999999999147, -30.61874999877096926, 99.99999999999998579 ) ) ;
#8528=CARTESIAN_POINT ( 'NONE',  ( 83.77821517812500929, -34.71562499938548285, 102.3871387122750889 ) ) ;
#8529=CARTESIAN_POINT ( 'NONE',  ( -82.40000000000000568, -33.03750000000000142, -96.99999999999998579 ) ) ;
#8531=DIRECTION ( 'NONE',  ( -1.000000000000000000, 1.445602896647337931E-15, 0.000000000000000000 ) ) ;
#8534=CARTESIAN_POINT ( 'NONE',  ( -83.77821517812500929, -32.87812499938548427, -97.61286128772489690 ) ) ;
#8535=CARTESIAN_POINT ( 'NONE',  ( 83.20384757729333103, -33.18615380933863435, -96.99999999999997158 ) ) ;
#8536=CARTESIAN_POINT ( 'NONE',  ( 79.64356964374999848, -33.17812499938548854, -99.99999999999998579 ) ) ;
#8538=CARTESIAN_POINT ( 'NONE',  ( -81.02178482187500208, -33.44062499938548427, 97.61286128772489690 ) ) ;
#8539=CARTESIAN_POINT ( 'NONE',  ( 85.15643035625001289, -31.94062499938548427, -99.99999999999998579 ) ) ;
#8541=CARTESIAN_POINT ( 'NONE',  ( 79.64356964375001269, -34.11562499938548854, 98.40857419181659793 ) ) ;
#8542=CARTESIAN_POINT ( 'NONE',  ( 99.99999999999998579, 0.000000000000000000, 150.0000000000000000 ) ) ;
#8544=CARTESIAN_POINT ( 'NONE',  ( -83.77821517812500929, -34.26562499938548711, 97.61286128772489690 ) ) ;
#8545=CARTESIAN_POINT ( 'NONE',  ( -85.15643035624999868, -30.17812499938548498, 98.40857419181659793 ) ) ;
#8550=CARTESIAN_POINT ( 'NONE',  ( 83.90000000000000568, -33.67500000000000426, -97.40192378864668399 ) ) ;
#8552=ADVANCED_FACE ( 'NONE', ( #12226 ), #3531, .F. ) ;
#8554=CARTESIAN_POINT ( 'NONE',  ( 84.56803305035323604, -32.00000000000000000, 98.28830862702034210 ) ) ;
#8555=CARTESIAN_POINT ( 'NONE',  ( 85.15643035624999868, -30.66562499938548569, 98.40857419181659793 ) ) ;
#8558=CARTESIAN_POINT ( 'NONE',  ( 82.39999999999999147, -34.64062499938548711, -103.1828516163667899 ) ) ;
#8559=CARTESIAN_POINT ( 'NONE',  ( 80.90000000000000568, -32.94374999877096855, 97.40192378864668399 ) ) ;
#8562=CARTESIAN_POINT ( 'NONE',  ( 79.39999999999999147, -32.38124999877096855, 101.7320508075688821 ) ) ;
#8568=VERTEX_POINT ( 'NONE', #4817 ) ;
#8569=CARTESIAN_POINT ( 'NONE',  ( -85.15643035625001289, -33.74062499938548854, -99.99999999999998579 ) ) ;
#8571=EDGE_LOOP ( 'NONE', ( #2928, #16701, #1345, #1754 ) ) ;
#8574=CARTESIAN_POINT ( 'NONE',  ( -79.64356964375001269, -30.51562499938548711, -98.40857419181659793 ) ) ;
#8575=PLANE ( 'NONE',  #5507 ) ;
#8576=CARTESIAN_POINT ( 'NONE',  ( 82.40000000000000568, -34.55624999877097281, -97.00000000000000000 ) ) ;
#8582=CARTESIAN_POINT ( 'NONE',  ( 82.39999999999999147, -30.73124999877096641, -103.4641016151377499 ) ) ;
#8584=VERTEX_POINT ( 'NONE', #10855 ) ;
#8594=CARTESIAN_POINT ( 'NONE',  ( -80.90000000000000568, -34.20000000000000284, -102.5980762113533018 ) ) ;
#8599=CARTESIAN_POINT ( 'NONE',  ( 82.39999999999999147, -33.03750000000000142, -103.4641016151377499 ) ) ;
#8602=CARTESIAN_POINT ( 'NONE',  ( -85.15643035625001289, -30.70312499938548711, 99.99999999999998579 ) ) ;
#8604=CYLINDRICAL_SURFACE ( 'NONE', #13980, 3.000000000000002665 ) ;
#8605=DIRECTION ( 'NONE',  ( 1.000000000000000000, 0.000000000000000000, -0.000000000000000000 ) ) ;
#8606=CARTESIAN_POINT ( 'NONE',  ( 82.65333140691207348, -34.99995246259152992, 102.9892844631211943 ) ) ;
#8607=CARTESIAN_POINT ( 'NONE',  ( -82.40000000000000568, -30.00000000000000355, 103.0000000000000000 ) ) ;
#8612=CARTESIAN_POINT ( 'NONE',  ( -82.39999999999999147, -31.37812499938548427, -96.81714838363319586 ) ) ;
#8621=FACE_OUTER_BOUND ( 'NONE', #4083, .T. ) ;
#8622=CARTESIAN_POINT ( 'NONE',  ( 85.15643035624999868, -35.05312499938548143, 98.40857419181659793 ) ) ;
#8627=CARTESIAN_POINT ( 'NONE',  ( -82.39999999999999147, -33.96562499938548285, -103.1828516163667899 ) ) ;
#8628=CARTESIAN_POINT ( 'NONE',  ( 81.02178482187500208, -34.79062499938548569, 102.3871387122750889 ) ) ;
#8629=CARTESIAN_POINT ( 'NONE',  ( 81.02178482187500208, -35.05312499938548854, -102.3871387122750889 ) ) ;
#8631=CARTESIAN_POINT ( 'NONE',  ( -82.39999999999999147, -33.17812499938548854, 103.1828516163667899 ) ) ;
#8632=CARTESIAN_POINT ( 'NONE',  ( 81.02178482187500208, -31.79062499938548925, -102.3871387122750889 ) ) ;
#8633=EDGE_CURVE ( 'NONE', #13113, #13520, #9446, .T. ) ;
#8634=ORIENTED_EDGE ( 'NONE', *, *, #11640, .F. ) ;
#8635=CARTESIAN_POINT ( 'NONE',  ( 85.15643035625001289, -34.75312499938548427, 99.99999999999998579 ) ) ;
#8636=FACE_OUTER_BOUND ( 'NONE', #11551, .T. ) ;
#8638=CARTESIAN_POINT ( 'NONE',  ( -79.64356964375001269, -32.57812499938548001, 98.40857419181659793 ) ) ;
#8639=ORIENTED_EDGE ( 'NONE', *, *, #15450, .F. ) ;
#8640=DIRECTION ( 'NONE',  ( -0.000000000000000000, -0.000000000000000000, -1.000000000000000000 ) ) ;
#8643=CARTESIAN_POINT ( 'NONE',  ( 79.69416654173913628, -34.99999999999998579, -100.6274906301335648 ) ) ;
#8645=AXIS2_PLACEMENT_3D ( 'NONE', #4762, #8853, #1435 ) ;
#8648=CARTESIAN_POINT ( 'NONE',  ( 82.40000000000000568, -30.00000000000000355, -99.99999999999998579 ) ) ;
#8650=CARTESIAN_POINT ( 'NONE',  ( 85.15643035624999868, -31.64062499938548356, 101.5914258081833879 ) ) ;
#8655=CARTESIAN_POINT ( 'NONE',  ( 79.64356964375001269, -33.59062499938548285, -98.40857419181659793 ) ) ;
#8657=VERTEX_POINT ( 'NONE', #14264 ) ;
#8658=CARTESIAN_POINT ( 'NONE',  ( 83.90000000000000568, -33.01874999877097139, 97.40192378864668399 ) ) ;
#8668=CARTESIAN_POINT ( 'NONE',  ( -85.15643035624999868, -35.11426541925033007, -101.0032526477118751 ) ) ;
#8669=DIRECTION ( 'NONE',  ( -0.000000000000000000, 0.000000000000000000, -1.000000000000000000 ) ) ;
#8673=CARTESIAN_POINT ( 'NONE',  ( -79.64356964374999848, -30.92812499938548498, -99.99999999999998579 ) ) ;
#8675=CARTESIAN_POINT ( 'NONE',  ( -82.39999999999999147, -32.30624999877097281, -103.4641016151377499 ) ) ;
#8680=CARTESIAN_POINT ( 'NONE',  ( -79.64356964374999848, -33.06562499938548427, -99.99999999999998579 ) ) ;
#8681=DIRECTION ( 'NONE',  ( 0.000000000000000000, 0.000000000000000000, 1.000000000000000000 ) ) ;
#8683=( BOUNDED_SURFACE ( )  B_SPLINE_SURFACE ( 1, 2, ( 
 ( #12062, #10884, #2976, #10500, #14895, #8932, #16466, #7857, #7569, #10786, #9218, #7659, #15181, #17933, #1799, #12260, #13718, #6112, #7765, #258, #18037, #4650, #10599, #4843, #1525, #6214, #359, #16748, #16564, #3362, #15089, #15581, #5331, #6594, #18415, #5429, #3558, #12540, #644, #15381, #543, #11268, #2192, #10975, #18612, #3457, #931, #5227, #835, #11074, #6693, #12837, #14197, #8149, #8339, #7953, #9808, #14296, #9515, #6887, #13906, #12636, #18803, #17236, #17141, #11175, #16946, #15481, #16853, #9414, #6795, #12742, #15770, #3746, #1996, #17043, #6499, #12447, #18513, #5035, #18710, #2092, #9712, #3654, #3842, #8050, #14006, #15674, #5130, #2283, #9620, #14100, #738, #8246, #2379, #13117, #7068, #4236, #4334, #11367, #16057, #8723, #17434, #14386, #1108, #14478, #17723, #18899, #10101, #6977, #11753, #5708, #8433, #2565, #5520, #10193, #13313, #1025, #7356, #14676, #2661, #4045, #8528, #10294, #16155, #10004, #12928, #19088, #11467, #19287, #1311, #8622, #15959, #13025, #16254, #2767, #18996 ),
 ( #13214, #5618, #14776, #17333, #7259, #11563, #14573, #19185, #17526, #8820, #5801, #2863, #4138, #1404, #1210, #7167, #3942, #11657, #9908, #15871, #2477, #17621, #16637, #3241, #1689, #7641, #9105, #15068, #4521, #2148, #7454, #2957, #13504, #16546, #17915, #12237, #3053, #12040, #9199, #9016, #143, #3145, #14873, #13595, #15162, #6192, #6093, #13412, #3338, #13700, #12142, #14976, #11944, #16444, #10479, #1599, #14058, #4725, #7546, #18014, #341, #4627, #1780, #42, #6288, #16729, #11848, #5993, #10581, #236, #18111, #10668, #7743, #18205, #16347, #4824, #15531, #10764, #9298, #8105, #8912, #5902, #17816, #4426, #10385, #1502, #5475, #8476, #8201, #6933, #12592, #3892, #15630, #4089, #2519, #15914, #3995, #10051, #14434, #9669, #7024, #18757, #5376, #2330, #18661, #692, #8294, #9960, #17289, #17091, #9762, #11421, #11225, #9860, #17190, #1067, #15724, #6646, #12788, #17381, #5280, #12978, #14152, #3703, #18948, #3794, #5572, #14244, #16010, #18560, #18855, #882, #11324, #11519, #786, #17480, #2614 ) ),
 .UNSPECIFIED., .F., .F., .F. ) 
 B_SPLINE_SURFACE_WITH_KNOTS ( ( 2, 2 ),
 ( 3, 2, 2, 2, 2, 2, 2, 2, 2, 2, 2, 2, 2, 2, 2, 2, 2, 2, 2, 2, 2, 2, 2, 2, 2, 2, 2, 2, 2, 2, 2, 2, 2, 2, 2, 2, 2, 2, 2, 2, 2, 2, 2, 2, 2, 2, 2, 2, 2, 2, 2, 2, 2, 2, 2, 2, 2, 2, 2, 2, 2, 2, 2, 2, 2, 2, 2, 2, 3 ),
 ( 0.000000000000000000, 1.000000000000000000 ),
 ( 0.000000000000000000, 0.01388888888888888812, 0.02777777777777777624, 0.04166666666666666435, 0.05555555555555555247, 0.06944444444444444753, 0.08333333333333332871, 0.09722222222222222376, 0.1111111111111111049, 0.1250000000000000000, 0.1388888888888888951, 0.1527777777777777901, 0.1666666666666666574, 0.1805555555555555525, 0.1944444444444444475, 0.2083333333333333426, 0.2222222222222222099, 0.2361111111111111049, 0.2500000000000000000, 0.2638888888888888951, 0.2777777777777777901, 0.2916666666666666852, 0.3055555555555555802, 0.3194444444444444198, 0.3333333333333333148, 0.3472222222222222099, 0.3611111111111111049, 0.3750000000000000000, 0.3888888888888888951, 0.4027777777777777901, 0.4166666666666666852, 0.4305555555555555802, 0.4444444444444444198, 0.4583333333333333148, 0.4722222222222222099, 0.4861111111111111049, 0.5000000000000000000, 0.5138888888888888395, 0.5277777777777777901, 0.5416666666666666297, 0.5555555555555555802, 0.5694444444444444198, 0.5833333333333333703, 0.5972222222222222099, 0.6111111111111111605, 0.6250000000000000000, 0.6388888888888888395, 0.6527777777777777901, 0.6666666666666666297, 0.6805555555555555802, 0.6944444444444444198, 0.7083333333333333703, 0.7222222222222222099, 0.7361111111111111605, 0.7500000000000000000, 0.7638888888888888395, 0.7777777777777777901, 0.7916666666666666297, 0.8055555555555555802, 0.8194444444444444198, 0.8333333333333333703, 0.8472222222222222099, 0.8611111111111111605, 0.8750000000000000000, 0.8888888888888888395, 0.9027777777777777901, 0.9166666666666666297, 0.9258785066912882389, 0.9351372917582011501 ),
 .UNSPECIFIED. ) 
 GEOMETRIC_REPRESENTATION_ITEM ( )  RATIONAL_B_SPLINE_SURFACE ( (
 ( 1.000000000000000000, 0.8660254037844387076, 1.000000000000000000, 0.8660254037844387076, 1.000000000000000000, 0.8660254037844387076, 1.000000000000000000, 0.8660254037844387076, 1.000000000000000000, 0.8660254037844387076, 1.000000000000000000, 0.8660254037844387076, 1.000000000000000000, 0.8660254037844387076, 1.000000000000000000, 0.8660254037844387076, 1.000000000000000000, 0.8660254037844387076, 1.000000000000000000, 0.8660254037844387076, 1.000000000000000000, 0.8660254037844387076, 1.000000000000000000, 0.8660254037844387076, 1.000000000000000000, 0.8660254037844387076, 1.000000000000000000, 0.8660254037844387076, 1.000000000000000000, 0.8660254037844387076, 1.000000000000000000, 0.8660254037844387076, 1.000000000000000000, 0.8660254037844387076, 1.000000000000000000, 0.8660254037844387076, 1.000000000000000000, 0.8660254037844387076, 1.000000000000000000, 0.8660254037844387076, 1.000000000000000000, 0.8660254037844387076, 1.000000000000000000, 0.8660254037844387076, 1.000000000000000000, 0.8660254037844387076, 1.000000000000000000, 0.8660254037844387076, 1.000000000000000000, 0.8660254037844387076, 1.000000000000000000, 0.8660254037844387076, 1.000000000000000000, 0.8660254037844387076, 1.000000000000000000, 0.8660254037844387076, 1.000000000000000000, 0.8660254037844387076, 1.000000000000000000, 0.8660254037844387076, 1.000000000000000000, 0.8660254037844387076, 1.000000000000000000, 0.8660254037844387076, 1.000000000000000000, 0.8660254037844387076, 1.000000000000000000, 0.8660254037844387076, 1.000000000000000000, 0.8660254037844387076, 1.000000000000000000, 0.8660254037844387076, 1.000000000000000000, 0.8660254037844387076, 1.000000000000000000, 0.8660254037844387076, 1.000000000000000000, 0.8660254037844387076, 1.000000000000000000, 0.8660254037844387076, 1.000000000000000000, 0.8660254037844387076, 1.000000000000000000, 0.8660254037844387076, 1.000000000000000000, 0.8660254037844387076, 1.000000000000000000, 0.8660254037844387076, 1.000000000000000000, 0.8660254037844387076, 1.000000000000000000, 0.8660254037844387076, 1.000000000000000000, 0.8660254037844387076, 1.000000000000000000, 0.8660254037844387076, 1.000000000000000000, 0.8660254037844387076, 1.000000000000000000, 0.8660254037844387076, 1.000000000000000000, 0.8660254037844387076, 1.000000000000000000, 0.8660254037844387076, 1.000000000000000000, 0.8660254037844387076, 1.000000000000000000, 0.8660254037844387076, 1.000000000000000000, 0.8660254037844387076, 1.000000000000000000, 0.8660254037844387076, 1.000000000000000000, 0.8660254037844387076, 1.000000000000000000, 0.8660254037844387076, 1.000000000000000000, 0.8660254037844387076, 1.000000000000000000, 0.8660254037844387076, 1.000000000000000000, 0.8660254037844387076, 1.000000000000000000, 0.8660254037844387076, 1.000000000000000000, 0.8660254037844387076, 1.000000000000000000, 0.8660254037844387076, 1.000000000000000000, 0.8660254037844387076, 1.000000000000000000, 0.8660254037844387076, 1.000000000000000000, 0.9111410165655264848, 0.9401539157124900736, 0.9401539157124900736, 0.9401539157124900736),
 ( 1.000000000000000000, 0.8660254037844387076, 1.000000000000000000, 0.8660254037844387076, 1.000000000000000000, 0.8660254037844387076, 1.000000000000000000, 0.8660254037844387076, 1.000000000000000000, 0.8660254037844387076, 1.000000000000000000, 0.8660254037844387076, 1.000000000000000000, 0.8660254037844387076, 1.000000000000000000, 0.8660254037844387076, 1.000000000000000000, 0.8660254037844387076, 1.000000000000000000, 0.8660254037844387076, 1.000000000000000000, 0.8660254037844387076, 1.000000000000000000, 0.8660254037844387076, 1.000000000000000000, 0.8660254037844387076, 1.000000000000000000, 0.8660254037844387076, 1.000000000000000000, 0.8660254037844387076, 1.000000000000000000, 0.8660254037844387076, 1.000000000000000000, 0.8660254037844387076, 1.000000000000000000, 0.8660254037844387076, 1.000000000000000000, 0.8660254037844387076, 1.000000000000000000, 0.8660254037844387076, 1.000000000000000000, 0.8660254037844387076, 1.000000000000000000, 0.8660254037844387076, 1.000000000000000000, 0.8660254037844387076, 1.000000000000000000, 0.8660254037844387076, 1.000000000000000000, 0.8660254037844387076, 1.000000000000000000, 0.8660254037844387076, 1.000000000000000000, 0.8660254037844387076, 1.000000000000000000, 0.8660254037844387076, 1.000000000000000000, 0.8660254037844387076, 1.000000000000000000, 0.8660254037844387076, 1.000000000000000000, 0.8660254037844387076, 1.000000000000000000, 0.8660254037844387076, 1.000000000000000000, 0.8660254037844387076, 1.000000000000000000, 0.8660254037844387076, 1.000000000000000000, 0.8660254037844387076, 1.000000000000000000, 0.8660254037844387076, 1.000000000000000000, 0.8660254037844387076, 1.000000000000000000, 0.8660254037844387076, 1.000000000000000000, 0.8660254037844387076, 1.000000000000000000, 0.8660254037844387076, 1.000000000000000000, 0.8660254037844387076, 1.000000000000000000, 0.8660254037844387076, 1.000000000000000000, 0.8660254037844387076, 1.000000000000000000, 0.8660254037844387076, 1.000000000000000000, 0.8660254037844387076, 1.000000000000000000, 0.8660254037844387076, 1.000000000000000000, 0.8660254037844387076, 1.000000000000000000, 0.8660254037844387076, 1.000000000000000000, 0.8660254037844387076, 1.000000000000000000, 0.8660254037844387076, 1.000000000000000000, 0.8660254037844387076, 1.000000000000000000, 0.8660254037844387076, 1.000000000000000000, 0.8660254037844387076, 1.000000000000000000, 0.8660254037844387076, 1.000000000000000000, 0.8660254037844387076, 1.000000000000000000, 0.8660254037844387076, 1.000000000000000000, 0.8660254037844387076, 1.000000000000000000, 0.8660254037844387076, 1.000000000000000000, 0.8660254037844387076, 1.000000000000000000, 0.8660254037844387076, 1.000000000000000000, 0.8660254037844387076, 1.000000000000000000, 0.8660254037844387076, 1.000000000000000000, 0.8660254037844387076, 1.000000000000000000, 0.8660254037844387076, 1.000000000000000000, 0.8660254037844387076, 1.000000000000000000, 0.8660254037844387076, 1.000000000000000000, 0.9111410165655264848, 0.9401539157124900736, 0.9401539157124900736, 0.9401539157124900736) ) ) 
 REPRESENTATION_ITEM ( '' )  SURFACE ( )  );
#8686=CARTESIAN_POINT ( 'NONE',  ( 79.39999999999999147, -30.61874999877096926, -99.99999999999998579 ) ) ;
#8698=CARTESIAN_POINT ( 'NONE',  ( -79.90595866893276877, -34.99999999999997868, -98.81289630734772800 ) ) ;
#8702=CARTESIAN_POINT ( 'NONE',  ( 83.41996205656103314, -34.99999999999999289, 102.8282615748025535 ) ) ;
#8704=CARTESIAN_POINT ( 'NONE',  ( -79.64356964374999848, -30.92812499938548498, 99.99999999999998579 ) ) ;
#8707=CARTESIAN_POINT ( 'NONE',  ( 79.91954014136220508, -34.99999999999999289, 101.4427624130899375 ) ) ;
#8708=LINE ( 'NONE', #13011, #7734 ) ;
#8710=CARTESIAN_POINT ( 'NONE',  ( -85.15643035624999868, -30.55312499938548854, -98.40857419181659793 ) ) ;
#8720=CARTESIAN_POINT ( 'NONE',  ( -84.53225329756190831, -32.00000000000000711, 98.24409948398896120 ) ) ;
#8722=CARTESIAN_POINT ( 'NONE',  ( -83.95700771753406855, -35.00000000000000711, -102.5724980549416898 ) ) ;
#8723=CARTESIAN_POINT ( 'NONE',  ( 79.64356964375001269, -33.92812499938548854, 101.5914258081833879 ) ) ;
#8724=CARTESIAN_POINT ( 'NONE',  ( 85.40000000000000568, -34.05000000000000426, -99.99999999999998579 ) ) ;
#8728=CARTESIAN_POINT ( 'NONE',  ( 82.39999999999999147, -32.98124999877096286, -102.9999999999999858 ) ) ;
#8729=CARTESIAN_POINT ( 'NONE',  ( 81.02178482187500208, -31.64062499938548356, -97.61286128772489690 ) ) ;
#8731=CARTESIAN_POINT ( 'NONE',  ( -85.15643035625001289, -32.35312499938548569, 101.5914258081833879 ) ) ;
#8732=CARTESIAN_POINT ( 'NONE',  ( 82.39999999999999147, -32.05312499938548854, -96.81714838363319586 ) ) ;
#8733=ORIENTED_EDGE ( 'NONE', *, *, #12577, .T. ) ;
#8735=CARTESIAN_POINT ( 'NONE',  ( 79.39999999999999147, -33.82500000000000284, -99.99999999999998579 ) ) ;
#8737=CARTESIAN_POINT ( 'NONE',  ( -85.15643035624999868, -32.42812499938548854, 98.40857419181659793 ) ) ;
#8739=CARTESIAN_POINT ( 'NONE',  ( -83.20395887649198130, -35.00000000000002132, 102.6365808225363025 ) ) ;
#8742=CARTESIAN_POINT ( 'NONE',  ( 79.64057174634724845, -34.99999999999999289, -100.3964642588221494 ) ) ;
#8745=EDGE_CURVE ( 'NONE', #14868, #14513, #4065, .T. ) ;
#8746=CARTESIAN_POINT ( 'NONE',  ( -82.40000000000000568, -32.00000000000000000, -99.99999999999998579 ) ) ;
#8750=CARTESIAN_POINT ( 'NONE',  ( 79.64356964375001269, -33.21562499938548996, 98.40857419181659793 ) ) ;
#8751=CARTESIAN_POINT ( 'NONE',  ( 110.9999999999999574, -21.80000000000003268, -139.9999999999999716 ) ) ;
#8753=CARTESIAN_POINT ( 'NONE',  ( 79.64356964375001269, -33.14062499938548711, -98.40857419181659793 ) ) ;
#8754=CARTESIAN_POINT ( 'NONE',  ( -79.64356964374999848, -31.82812499938548356, -99.99999999999998579 ) ) ;
#8756=CARTESIAN_POINT ( 'NONE',  ( 79.39999999999999147, -32.86874999877097281, 99.99999999999998579 ) ) ;
#8761=CARTESIAN_POINT ( 'NONE',  ( -83.77821517812500929, -30.32812499938548711, 97.61286128772489690 ) ) ;
#8762=CARTESIAN_POINT ( 'NONE',  ( 83.52022063339155977, -31.99999999999999289, 102.5731757465994036 ) ) ;
#8765=CARTESIAN_POINT ( 'NONE',  ( -85.15643035625001289, -32.84062499938548285, -99.99999999999998579 ) ) ;
#8770=CARTESIAN_POINT ( 'NONE',  ( -82.39999999999999147, -34.41562499938547859, -103.1828516163667899 ) ) ;
#8771=( BOUNDED_SURFACE ( )  B_SPLINE_SURFACE ( 1, 2, ( 
 ( #11378, #8351, #1221, #6987, #13127, #14305, #17444, #19007, #17632, #13036, #12938, #4151, #4247, #16067, #19097, #11280, #2389, #3855, #941, #5627, #12846, #1034, #15972, #9818, #4055, #11573, #18815, #2485, #5439, #2673, #15780, #17344, #3954, #5718, #10014, #9919, #8443, #2578, #15881, #11668, #10205, #16168, #1120, #14396, #8632, #18910, #5529, #11477, #8539, #2779, #7080, #8732, #1610, #7365, #8830, #16555, #4734, #9117, #3155, #19298, #14986, #10680, #11761, #13515, #2873, #5912, #16649, #9208, #17737, #15173, #6205, #1790, #14787, #17924, #1413, #14884, #15079, #16357, #3064, #2967, #1698, #6102, #16455, #1514, #4343, #4533, #7650, #9026, #10590, #10305, #7755, #13605, #4641, #16262, #4437, #13710, #13322, #246, #6003, #10491, #12153, #11857, #5812, #18120, #3250, #17825, #10395, #8922, #7463, #13424, #53, #11954, #7558, #152, #12051, #18027, #2066, #3628, #11148, #10955, #18296, #6570, #15556, #5109, #717, #9690, #7836, #16832, #4915, #339, #4822, #2170, #6473, #18202, #9489, #12331, #8127 ),
 ( #9590, #8024, #10861, #13790, #16924, #5015, #1778, #14078, #622, #3439, #9390, #6671, #15356, #12518, #3335, #12614, #18587, #7740, #15261, #1973, #3536, #433, #18488, #5201, #17117, #3725, #13698, #6286, #12233, #6378, #10762, #16726, #9296, #1876, #7930, #15456, #11051, #17018, #13881, #520, #13984, #12427, #18395, #11248, #19066, #17503, #11541, #18971, #11633, #3918, #18876, #17595, #8316, #14268, #4113, #1188, #15748, #10076, #11444, #17212, #18688, #7044, #14550, #5595, #13001, #9786, #5498, #2258, #1086, #6956, #17407, #906, #16032, #2635, #4022, #9982, #15937, #2540, #6866, #9883, #12811, #8599, #8500, #12908, #18778, #7145, #5403, #2456, #13095, #11345, #15845, #5685, #810, #5304, #8411, #4207, #14454, #3817, #15652, #8227, #14174, #17311, #2353, #6768, #12714, #14364, #999, #9241, #12084, #19257, #4861, #1383, #1823, #11725, #10806, #1914, #16131, #4307, #4669, #281, #2838, #15205, #12280, #9338, #7877, #2740, #3386, #14651, #16233, #6419, #1286, #17693, #13828, #8792, #6232, #7783, #13737 ) ),
 .UNSPECIFIED., .F., .F., .F. ) 
 B_SPLINE_SURFACE_WITH_KNOTS ( ( 2, 2 ),
 ( 3, 2, 2, 2, 2, 2, 2, 2, 2, 2, 2, 2, 2, 2, 2, 2, 2, 2, 2, 2, 2, 2, 2, 2, 2, 2, 2, 2, 2, 2, 2, 2, 2, 2, 2, 2, 2, 2, 2, 2, 2, 2, 2, 2, 2, 2, 2, 2, 2, 2, 2, 2, 2, 2, 2, 2, 2, 2, 2, 2, 2, 2, 2, 2, 2, 2, 2, 2, 3 ),
 ( 0.000000000000000000, 1.000000000000000000 ),
 ( 0.000000000000000000, 0.01388888888888888812, 0.02777777777777777624, 0.04166666666666666435, 0.05555555555555555247, 0.06944444444444444753, 0.08333333333333332871, 0.09722222222222222376, 0.1111111111111111049, 0.1250000000000000000, 0.1388888888888888951, 0.1527777777777777901, 0.1666666666666666574, 0.1805555555555555525, 0.1944444444444444475, 0.2083333333333333426, 0.2222222222222222099, 0.2361111111111111049, 0.2500000000000000000, 0.2638888888888888951, 0.2777777777777777901, 0.2916666666666666852, 0.3055555555555555802, 0.3194444444444444198, 0.3333333333333333148, 0.3472222222222222099, 0.3611111111111111049, 0.3750000000000000000, 0.3888888888888888951, 0.4027777777777777901, 0.4166666666666666852, 0.4305555555555555802, 0.4444444444444444198, 0.4583333333333333148, 0.4722222222222222099, 0.4861111111111111049, 0.5000000000000000000, 0.5138888888888888395, 0.5277777777777777901, 0.5416666666666666297, 0.5555555555555555802, 0.5694444444444444198, 0.5833333333333333703, 0.5972222222222222099, 0.6111111111111111605, 0.6250000000000000000, 0.6388888888888888395, 0.6527777777777777901, 0.6666666666666666297, 0.6805555555555555802, 0.6944444444444444198, 0.7083333333333333703, 0.7222222222222222099, 0.7361111111111111605, 0.7500000000000000000, 0.7638888888888888395, 0.7777777777777777901, 0.7916666666666666297, 0.8055555555555555802, 0.8194444444444444198, 0.8333333333333333703, 0.8472222222222222099, 0.8611111111111111605, 0.8750000000000000000, 0.8888888888888888395, 0.9027777777777777901, 0.9166666666666666297, 0.9258785066912882389, 0.9351372917582011501 ),
 .UNSPECIFIED. ) 
 GEOMETRIC_REPRESENTATION_ITEM ( )  RATIONAL_B_SPLINE_SURFACE ( (
 ( 1.000000000000000000, 0.8660254037844387076, 1.000000000000000000, 0.8660254037844387076, 1.000000000000000000, 0.8660254037844387076, 1.000000000000000000, 0.8660254037844387076, 1.000000000000000000, 0.8660254037844387076, 1.000000000000000000, 0.8660254037844387076, 1.000000000000000000, 0.8660254037844387076, 1.000000000000000000, 0.8660254037844387076, 1.000000000000000000, 0.8660254037844387076, 1.000000000000000000, 0.8660254037844387076, 1.000000000000000000, 0.8660254037844387076, 1.000000000000000000, 0.8660254037844387076, 1.000000000000000000, 0.8660254037844387076, 1.000000000000000000, 0.8660254037844387076, 1.000000000000000000, 0.8660254037844387076, 1.000000000000000000, 0.8660254037844387076, 1.000000000000000000, 0.8660254037844387076, 1.000000000000000000, 0.8660254037844387076, 1.000000000000000000, 0.8660254037844387076, 1.000000000000000000, 0.8660254037844387076, 1.000000000000000000, 0.8660254037844387076, 1.000000000000000000, 0.8660254037844387076, 1.000000000000000000, 0.8660254037844387076, 1.000000000000000000, 0.8660254037844387076, 1.000000000000000000, 0.8660254037844387076, 1.000000000000000000, 0.8660254037844387076, 1.000000000000000000, 0.8660254037844387076, 1.000000000000000000, 0.8660254037844387076, 1.000000000000000000, 0.8660254037844387076, 1.000000000000000000, 0.8660254037844387076, 1.000000000000000000, 0.8660254037844387076, 1.000000000000000000, 0.8660254037844387076, 1.000000000000000000, 0.8660254037844387076, 1.000000000000000000, 0.8660254037844387076, 1.000000000000000000, 0.8660254037844387076, 1.000000000000000000, 0.8660254037844387076, 1.000000000000000000, 0.8660254037844387076, 1.000000000000000000, 0.8660254037844387076, 1.000000000000000000, 0.8660254037844387076, 1.000000000000000000, 0.8660254037844387076, 1.000000000000000000, 0.8660254037844387076, 1.000000000000000000, 0.8660254037844387076, 1.000000000000000000, 0.8660254037844387076, 1.000000000000000000, 0.8660254037844387076, 1.000000000000000000, 0.8660254037844387076, 1.000000000000000000, 0.8660254037844387076, 1.000000000000000000, 0.8660254037844387076, 1.000000000000000000, 0.8660254037844387076, 1.000000000000000000, 0.8660254037844387076, 1.000000000000000000, 0.8660254037844387076, 1.000000000000000000, 0.8660254037844387076, 1.000000000000000000, 0.8660254037844387076, 1.000000000000000000, 0.8660254037844387076, 1.000000000000000000, 0.8660254037844387076, 1.000000000000000000, 0.8660254037844387076, 1.000000000000000000, 0.8660254037844387076, 1.000000000000000000, 0.8660254037844387076, 1.000000000000000000, 0.8660254037844387076, 1.000000000000000000, 0.8660254037844387076, 1.000000000000000000, 0.8660254037844387076, 1.000000000000000000, 0.8660254037844387076, 1.000000000000000000, 0.8660254037844387076, 1.000000000000000000, 0.8660254037844387076, 1.000000000000000000, 0.8660254037844387076, 1.000000000000000000, 0.8660254037844387076, 1.000000000000000000, 0.8660254037844387076, 1.000000000000000000, 0.9111410165655264848, 0.9401539157124900736, 0.9401539157124900736, 0.9401539157124900736),
 ( 1.000000000000000000, 0.8660254037844387076, 1.000000000000000000, 0.8660254037844387076, 1.000000000000000000, 0.8660254037844387076, 1.000000000000000000, 0.8660254037844387076, 1.000000000000000000, 0.8660254037844387076, 1.000000000000000000, 0.8660254037844387076, 1.000000000000000000, 0.8660254037844387076, 1.000000000000000000, 0.8660254037844387076, 1.000000000000000000, 0.8660254037844387076, 1.000000000000000000, 0.8660254037844387076, 1.000000000000000000, 0.8660254037844387076, 1.000000000000000000, 0.8660254037844387076, 1.000000000000000000, 0.8660254037844387076, 1.000000000000000000, 0.8660254037844387076, 1.000000000000000000, 0.8660254037844387076, 1.000000000000000000, 0.8660254037844387076, 1.000000000000000000, 0.8660254037844387076, 1.000000000000000000, 0.8660254037844387076, 1.000000000000000000, 0.8660254037844387076, 1.000000000000000000, 0.8660254037844387076, 1.000000000000000000, 0.8660254037844387076, 1.000000000000000000, 0.8660254037844387076, 1.000000000000000000, 0.8660254037844387076, 1.000000000000000000, 0.8660254037844387076, 1.000000000000000000, 0.8660254037844387076, 1.000000000000000000, 0.8660254037844387076, 1.000000000000000000, 0.8660254037844387076, 1.000000000000000000, 0.8660254037844387076, 1.000000000000000000, 0.8660254037844387076, 1.000000000000000000, 0.8660254037844387076, 1.000000000000000000, 0.8660254037844387076, 1.000000000000000000, 0.8660254037844387076, 1.000000000000000000, 0.8660254037844387076, 1.000000000000000000, 0.8660254037844387076, 1.000000000000000000, 0.8660254037844387076, 1.000000000000000000, 0.8660254037844387076, 1.000000000000000000, 0.8660254037844387076, 1.000000000000000000, 0.8660254037844387076, 1.000000000000000000, 0.8660254037844387076, 1.000000000000000000, 0.8660254037844387076, 1.000000000000000000, 0.8660254037844387076, 1.000000000000000000, 0.8660254037844387076, 1.000000000000000000, 0.8660254037844387076, 1.000000000000000000, 0.8660254037844387076, 1.000000000000000000, 0.8660254037844387076, 1.000000000000000000, 0.8660254037844387076, 1.000000000000000000, 0.8660254037844387076, 1.000000000000000000, 0.8660254037844387076, 1.000000000000000000, 0.8660254037844387076, 1.000000000000000000, 0.8660254037844387076, 1.000000000000000000, 0.8660254037844387076, 1.000000000000000000, 0.8660254037844387076, 1.000000000000000000, 0.8660254037844387076, 1.000000000000000000, 0.8660254037844387076, 1.000000000000000000, 0.8660254037844387076, 1.000000000000000000, 0.8660254037844387076, 1.000000000000000000, 0.8660254037844387076, 1.000000000000000000, 0.8660254037844387076, 1.000000000000000000, 0.8660254037844387076, 1.000000000000000000, 0.8660254037844387076, 1.000000000000000000, 0.8660254037844387076, 1.000000000000000000, 0.8660254037844387076, 1.000000000000000000, 0.8660254037844387076, 1.000000000000000000, 0.8660254037844387076, 1.000000000000000000, 0.8660254037844387076, 1.000000000000000000, 0.8660254037844387076, 1.000000000000000000, 0.9111410165655264848, 0.9401539157124900736, 0.9401539157124900736, 0.9401539157124900736) ) ) 
 REPRESENTATION_ITEM ( '' )  SURFACE ( )  );
#8773=CARTESIAN_POINT ( 'NONE',  ( -79.39999999999999147, -31.03124999877097068, -101.7320508075688821 ) ) ;
#8779=CARTESIAN_POINT ( 'NONE',  ( 82.39999999999999147, -31.40624999877097068, -96.53589838486223584 ) ) ;
#8786=ORIENTED_EDGE ( 'NONE', *, *, #12126, .T. ) ;
#8788=CARTESIAN_POINT ( 'NONE',  ( -79.39999999999999147, -32.01330983656955453, 99.46005447972481761 ) ) ;
#8791=CARTESIAN_POINT ( 'NONE',  ( -81.28488860390729087, -34.99999999999999289, 102.5271494742948590 ) ) ;
#8792=CARTESIAN_POINT ( 'NONE',  ( 85.39999999999999147, -34.97364041986484295, -98.90809577818232867 ) ) ;
#8793=EDGE_CURVE ( 'NONE', #11084, #14672, #84, .T. ) ;
#8795=VECTOR ( 'NONE', #11988, 1000.000000000000000 ) ;
#8796=VECTOR ( 'NONE', #17888, 1000.000000000000000 ) ;
#8797=CARTESIAN_POINT ( 'NONE',  ( -83.77821517812500929, -35.12812499938548427, 102.3871387122750889 ) ) ;
#8800=CARTESIAN_POINT ( 'NONE',  ( 82.39999999999999147, -33.43124999877097281, 96.99999999999998579 ) ) ;
#8801=EDGE_CURVE ( 'NONE', #13499, #16790, #8054, .T. ) ;
#8802=CARTESIAN_POINT ( 'NONE',  ( 79.69416654173916470, -35.00000000000000711, 99.37250936986644945 ) ) ;
#8803=CARTESIAN_POINT ( 'NONE',  ( 85.29357727954827340, -35.00000000000000711, 99.68450386720812162 ) ) ;
#8805=ORIENTED_EDGE ( 'NONE', *, *, #11373, .F. ) ;
#8806=CARTESIAN_POINT ( 'NONE',  ( -82.39999999999999147, -34.86562499938548854, -103.1828516163667899 ) ) ;
#8807=CARTESIAN_POINT ( 'NONE',  ( -85.40000000000000568, -33.56250000000000000, 101.7320508075688821 ) ) ;
#8813=CARTESIAN_POINT ( 'NONE',  ( 79.39999999999999147, -33.37500000000000000, 99.99999999999998579 ) ) ;
#8816=ORIENTED_EDGE ( 'NONE', *, *, #14008, .T. ) ;
#8819=CARTESIAN_POINT ( 'NONE',  ( -80.90000000000000568, -32.04374999877096997, 102.5980762113533018 ) ) ;
#8820=CARTESIAN_POINT ( 'NONE',  ( 82.39999999999999147, -30.33750000000000213, 96.53589838486223584 ) ) ;
#8826=CARTESIAN_POINT ( 'NONE',  ( 83.77821517812500929, -34.56562499938548427, 97.61286128772489690 ) ) ;
#8827=CARTESIAN_POINT ( 'NONE',  ( 83.77821517812500929, -31.86562499938548498, -102.3871387122750889 ) ) ;
#8829=CARTESIAN_POINT ( 'NONE',  ( -79.64356964374999848, -34.86562499938548143, 99.99999999999998579 ) ) ;
#8830=CARTESIAN_POINT ( 'NONE',  ( 79.64356964374999848, -32.16562499938548569, -99.99999999999998579 ) ) ;
#8836=CARTESIAN_POINT ( 'NONE',  ( -79.64356964374999848, -32.61562499938548854, 99.99999999999998579 ) ) ;
#8842=DIRECTION ( 'NONE',  ( 2.312964634635742582E-14, -1.000000000000000000, 0.000000000000000000 ) ) ;
#8843=CARTESIAN_POINT ( 'NONE',  ( -85.40000000000000568, -32.25000000000000000, 99.99999999999998579 ) ) ;
#8846=CARTESIAN_POINT ( 'NONE',  ( 85.15643035624999868, -33.44062499938548427, 101.5914258081833879 ) ) ;
#8847=DIRECTION ( 'NONE',  ( 0.000000000000000000, 0.000000000000000000, 1.000000000000000000 ) ) ;
#8848=CARTESIAN_POINT ( 'NONE',  ( -82.39999999999999147, -32.58749999999999858, -96.99999999999998579 ) ) ;
#8849=CARTESIAN_POINT ( 'NONE',  ( -84.44763168836716716, -32.00000000000000000, 101.8452947671445799 ) ) ;
#8850=CARTESIAN_POINT ( 'NONE',  ( -79.64356964375001269, -30.44062499938548783, -101.5914258081833879 ) ) ;
#8851=ORIENTED_EDGE ( 'NONE', *, *, #1842, .T. ) ;
#8852=CARTESIAN_POINT ( 'NONE',  ( 83.90000000000000568, -33.91874999877096997, 97.40192378864668399 ) ) ;
#8853=DIRECTION ( 'NONE',  ( 0.000000000000000000, -1.000000000000000000, 0.000000000000000000 ) ) ;
#8854=CARTESIAN_POINT ( 'NONE',  ( 83.20384757729335945, -32.73615380933863150, 102.9999999999999716 ) ) ;
#8856=CARTESIAN_POINT ( 'NONE',  ( -85.15643035625001289, -31.15312499938548996, 99.99999999999998579 ) ) ;
#8857=CARTESIAN_POINT ( 'NONE',  ( 81.90908125320002853, -31.99999999999999289, 102.8381494550125126 ) ) ;
#8859=CARTESIAN_POINT ( 'NONE',  ( -85.15643035624999868, -32.87812499938549138, -101.5914258081833879 ) ) ;
#8861=CARTESIAN_POINT ( 'NONE',  ( -85.15643035625001289, -32.50312499938548427, -99.99999999999998579 ) ) ;
#8863=CARTESIAN_POINT ( 'NONE',  ( -83.90000000000000568, -31.36874999877096926, -102.5980762113533018 ) ) ;
#8867=CARTESIAN_POINT ( 'NONE',  ( -85.15643035625001289, -34.22812499938548569, -101.5914258081833879 ) ) ;
#8870=DIRECTION ( 'NONE',  ( 0.000000000000000000, 1.000000000000000000, 0.000000000000000000 ) ) ;
#8871=CARTESIAN_POINT ( 'NONE',  ( 79.39999999999999147, -33.76874999877097139, -99.99999999999998579 ) ) ;
#8873=ORIENTED_EDGE ( 'NONE', *, *, #18365, .T. ) ;
#8874=CARTESIAN_POINT ( 'NONE',  ( 99.99999999999994316, -29.80000000000000782, 150.0000000000000000 ) ) ;
#8881=CARTESIAN_POINT ( 'NONE',  ( -79.39999999999999147, -34.31250000000000000, -98.26794919243113213 ) ) ;
#8882=( BOUNDED_CURVE ( )  B_SPLINE_CURVE ( 2, ( #2139, #10826, #9556, #18362, #6540, #7706, #15131 ),
 .UNSPECIFIED., .F., .F. ) 
 B_SPLINE_CURVE_WITH_KNOTS ( ( 3, 2, 2, 3 ),
 ( 0.8958333333333333703, 0.9027777777777777901, 0.9166666666666666297, 0.9258785066912882389 ),
 .UNSPECIFIED. ) 
 CURVE ( )  GEOMETRIC_REPRESENTATION_ITEM ( )  RATIONAL_B_SPLINE_CURVE ( ( 0.9330127018922192983, 0.9330127018922198534, 1.000000000000000000, 0.8660254037844387076, 1.000000000000000000, 0.9111410165655264848, 0.9401539157124900736 ) ) 
 REPRESENTATION_ITEM ( '' )  );
#8886=CARTESIAN_POINT ( 'NONE',  ( -81.96801452314031167, -35.00000000000000000, 102.7281823352556529 ) ) ;
#8888=CARTESIAN_POINT ( 'NONE',  ( -85.15643035624999868, -34.79062499938548569, 98.40857419181659793 ) ) ;
#8892=EDGE_CURVE ( 'NONE', #11060, #14, #14042, .T. ) ;
#8893=DIRECTION ( 'NONE',  ( -2.312964634635742582E-14, 1.000000000000000000, 0.000000000000000000 ) ) ;
#8894=CARTESIAN_POINT ( 'NONE',  ( -82.40000000000000568, -34.55624999877097281, -102.9999999999999858 ) ) ;
#8897=CARTESIAN_POINT ( 'NONE',  ( -81.02178482187500208, -34.04062499938548569, -97.61286128772489690 ) ) ;
#8898=CARTESIAN_POINT ( 'NONE',  ( -83.20384757729335945, -33.69240381056766154, 96.99999999999998579 ) ) ;
#8911=CARTESIAN_POINT ( 'NONE',  ( -85.40000000000000568, -31.70624999877096784, 101.7320508075688679 ) ) ;
#8912=CARTESIAN_POINT ( 'NONE',  ( 80.90000000000000568, -33.00000000000000000, 97.40192378864668399 ) ) ;
#8913=CARTESIAN_POINT ( 'NONE',  ( 85.40000000000000568, -33.54374999877096286, 99.99999999999998579 ) ) ;
#8915=AXIS2_PLACEMENT_3D ( 'NONE', #9033, #13523, #14997 ) ;
#8917=CARTESIAN_POINT ( 'NONE',  ( 82.39999999999999147, -34.30312499938548143, 103.1828516163667899 ) ) ;
#8918=CARTESIAN_POINT ( 'NONE',  ( 81.02178482187500208, -30.29062499938548569, -97.61286128772489690 ) ) ;
#8921=CARTESIAN_POINT ( 'NONE',  ( 82.39999999999999147, -34.83749999999999858, -103.0000000000000000 ) ) ;
#8922=CARTESIAN_POINT ( 'NONE',  ( 85.15643035624999868, -34.15312499938548285, -101.5914258081833879 ) ) ;
#8924=CARTESIAN_POINT ( 'NONE',  ( -82.40000000000000568, -30.00000000000000355, -99.99999999999998579 ) ) ;
#8928=CARTESIAN_POINT ( 'NONE',  ( -85.40000000000000568, -30.41249999999999787, 101.7320508075688679 ) ) ;
#8929=EDGE_LOOP ( 'NONE', ( #10000, #1055, #18553, #11594 ) ) ;
#8930=CARTESIAN_POINT ( 'NONE',  ( -79.39999999999999147, -32.92500000000000426, 99.99999999999998579 ) ) ;
#8932=CARTESIAN_POINT ( 'NONE',  ( 79.64356964375001269, -30.32812499938548711, 101.5914258081833879 ) ) ;
#8934=CARTESIAN_POINT ( 'NONE',  ( 82.40000000000000568, -30.00000000000000355, 96.99999999999998579 ) ) ;
#8935=CARTESIAN_POINT ( 'NONE',  ( -82.40000000000001990, -32.13750000000000284, 103.0000000000000000 ) ) ;
#8937=CARTESIAN_POINT ( 'NONE',  ( 84.41281071784439405, -31.99999999999999289, 101.8917842577544519 ) ) ;
#8938=CARTESIAN_POINT ( 'NONE',  ( 79.64356964375001269, -32.69062499938548427, 101.5914258081833879 ) ) ;
#8939=CARTESIAN_POINT ( 'NONE',  ( 81.59615242270662350, -32.06115380933863435, 96.99999999999997158 ) ) ;
#8941=CARTESIAN_POINT ( 'NONE',  ( -84.41281071784422352, -32.00000000000000000, -101.8917842577546651 ) ) ;
#8942=CARTESIAN_POINT ( 'NONE',  ( -83.77821517812500929, -30.62812499938548783, -97.61286128772489690 ) ) ;
#8944=CARTESIAN_POINT ( 'NONE',  ( 79.39999999999999147, -35.11874999877096570, 99.99999999999998579 ) ) ;
#8945=STYLED_ITEM('',(#19350),#3164);
#8946=CARTESIAN_POINT ( 'NONE',  ( 82.40000000000001990, -33.93750000000000711, -103.0000000000000000 ) ) ;
#8947=CARTESIAN_POINT ( 'NONE',  ( 85.40000000000000568, -32.64374999877097139, 99.99999999999998579 ) ) ;
#8948=DIRECTION ( 'NONE',  ( 0.000000000000000000, -1.000000000000000000, 0.000000000000000000 ) ) ;
#8949=CARTESIAN_POINT ( 'NONE',  ( -81.02178482187500208, -31.75312499938548427, 97.61286128772489690 ) ) ;
#8950=CARTESIAN_POINT ( 'NONE',  ( 79.39999999999999147, -33.76874999877097139, -99.99999999999998579 ) ) ;
#8952=CARTESIAN_POINT ( 'NONE',  ( -85.40000000000000568, -30.03750000000000497, -101.7320508075688679 ) ) ;
#8955=CARTESIAN_POINT ( 'NONE',  ( -82.39999999999999147, -33.96562499938548285, -103.1828516163667899 ) ) ;
#8956=DIRECTION ( 'NONE',  ( 0.000000000000000000, -1.000000000000000000, 0.000000000000000000 ) ) ;
#8957=CARTESIAN_POINT ( 'NONE',  ( -82.39999999999999147, -32.08124999877097139, -96.53589838486223584 ) ) ;
#8958=EDGE_CURVE ( 'NONE', #15307, #11060, #5040, .T. ) ;
#8965=CARTESIAN_POINT ( 'NONE',  ( 82.39999999999999147, -33.62812499938548427, 96.81714838363319586 ) ) ;
#8966=CARTESIAN_POINT ( 'NONE',  ( -82.39999999999999147, -32.36250000000000426, -102.9999999999999858 ) ) ;
#8967=DIRECTION ( 'NONE',  ( 0.000000000000000000, 0.000000000000000000, 1.000000000000000000 ) ) ;
#8968=CARTESIAN_POINT ( 'NONE',  ( 79.39999999999999147, -35.15624999877096712, -101.7320508075688537 ) ) ;
#8971=ORIENTED_EDGE ( 'NONE', *, *, #6864, .T. ) ;
#8980=CARTESIAN_POINT ( 'NONE',  ( 79.39999999999999147, -34.27499999999999858, -99.99999999999998579 ) ) ;
#8984=CARTESIAN_POINT ( 'NONE',  ( 79.39999999999999147, -32.41874999877096997, -99.99999999999998579 ) ) ;
#8985=DIRECTION ( 'NONE',  ( -0.000000000000000000, -0.000000000000000000, -1.000000000000000000 ) ) ;
#8989=CARTESIAN_POINT ( 'NONE',  ( -79.64356964375001269, -33.21562499938548996, 101.5914258081833879 ) ) ;
#8997=CARTESIAN_POINT ( 'NONE',  ( -81.59615242270662350, -34.57634618820329564, -103.0000000000000000 ) ) ;
#9001=CARTESIAN_POINT ( 'NONE',  ( -83.77821517812500929, -32.76562499938548711, -97.61286128772489690 ) ) ;
#9002=CARTESIAN_POINT ( 'NONE',  ( -82.39999999999999147, -33.48750000000000426, 103.0000000000000000 ) ) ;
#9003=VECTOR ( 'NONE', #8893, 1000.000000000000000 ) ;
#9005=CARTESIAN_POINT ( 'NONE',  ( 81.79008970393682887, -35.00000000000001421, -102.6939647107542299 ) ) ;
#9007=DIRECTION ( 'NONE',  ( 0.000000000000000000, 0.000000000000000000, 1.000000000000000000 ) ) ;
#9011=ORIENTED_EDGE ( 'NONE', *, *, #5069, .F. ) ;
#9012=DIRECTION ( 'NONE',  ( 1.000000000000000000, -4.625929269271494788E-16, 0.000000000000000000 ) ) ;
#9015=CARTESIAN_POINT ( 'NONE',  ( -82.39999999999999147, -31.85624999877097352, 96.53589838486223584 ) ) ;
#9016=CARTESIAN_POINT ( 'NONE',  ( 82.39999999999999147, -31.46250000000000568, 103.4641016151377499 ) ) ;
#9022=CARTESIAN_POINT ( 'NONE',  ( 82.39999999999999147, -30.92812499938548143, -103.1828516163667899 ) ) ;
#9026=CARTESIAN_POINT ( 'NONE',  ( 82.39999999999999147, -33.40312499938548285, -96.81714838363319586 ) ) ;
#9030=CARTESIAN_POINT ( 'NONE',  ( -83.88339518848731302, -35.16733441503058089, 97.47959136244114120 ) ) ;
#9033=CARTESIAN_POINT ( 'NONE',  ( -94.79999999999999716, -5.200000000000000178, 150.0000000000000000 ) ) ;
#9036=CARTESIAN_POINT ( 'NONE',  ( -82.40000000000001990, -32.53124999877097423, 103.0000000000000000 ) ) ;
#9039=CARTESIAN_POINT ( 'NONE',  ( 85.15643035625001289, -33.40312499938548285, 99.99999999999998579 ) ) ;
#9041=ADVANCED_FACE ( 'NONE', ( #7614 ), #16673, .F. ) ;
#9044=CARTESIAN_POINT ( 'NONE',  ( -84.44763168836720979, -32.00000000000001421, -98.15470523285542015 ) ) ;
#9046=CARTESIAN_POINT ( 'NONE',  ( 85.15643035624999868, -30.29062499938548925, 101.5914258081833879 ) ) ;
#9049=CARTESIAN_POINT ( 'NONE',  ( -85.15643035624999868, -32.54062499938548569, 98.40857419181659793 ) ) ;
#9050=CARTESIAN_POINT ( 'NONE',  ( -85.16220480609813137, -35.00000000000002132, -101.0868535717099661 ) ) ;
#9052=CARTESIAN_POINT ( 'NONE',  ( -85.40000000000000568, -31.83750000000000568, -101.7320508075688679 ) ) ;
#9054=CARTESIAN_POINT ( 'NONE',  ( 94.79999999999995453, -29.80000000000000071, 150.0000000000000000 ) ) ;
#9055=CARTESIAN_POINT ( 'NONE',  ( -79.64356964375001269, -34.04062499938549280, -101.5914258081833879 ) ) ;
#9056=CARTESIAN_POINT ( 'NONE',  ( 82.40000000000000568, -30.00000000000000355, -96.99999999999998579 ) ) ;
#9061=CARTESIAN_POINT ( 'NONE',  ( 83.77821517812500929, -34.11562499938548854, 97.61286128772489690 ) ) ;
#9062=CARTESIAN_POINT ( 'NONE',  ( -96.99999999999998579, -5.200000000000000178, 150.0000000000000000 ) ) ;
#9063=CYLINDRICAL_SURFACE ( 'NONE', #5844, 3.000000000000002665 ) ;
#9064=CARTESIAN_POINT ( 'NONE',  ( 85.40000000000000568, -35.30624999877096570, -101.7320508075688679 ) ) ;
#9075=CARTESIAN_POINT ( 'NONE',  ( -82.40000000000000568, -30.00000000000000355, 96.99999999999998579 ) ) ;
#9077=DIRECTION ( 'NONE',  ( -0.000000000000000000, -0.000000000000000000, -1.000000000000000000 ) ) ;
#9079=CARTESIAN_POINT ( 'NONE',  ( -81.02178482187500208, -34.15312499938548285, 102.3871387122750889 ) ) ;
#9086=CARTESIAN_POINT ( 'NONE',  ( -81.59615242270662350, -33.46740381056766722, 102.9999999999999716 ) ) ;
#9087=DIRECTION ( 'NONE',  ( 0.000000000000000000, 0.000000000000000000, -1.000000000000000000 ) ) ;
#9091=CARTESIAN_POINT ( 'NONE',  ( -81.02178482187500208, -34.34062499938548285, -102.3871387122750889 ) ) ;
#9093=LINE ( 'NONE', #13400, #4597 ) ;
#9094=CARTESIAN_POINT ( 'NONE',  ( 79.77811200999867935, -34.99999999999999289, -100.8506536761476013 ) ) ;
#9099=ADVANCED_FACE ( 'NONE', ( #16152, #10291, #19182 ), #3141, .F. ) ;
#9104=CARTESIAN_POINT ( 'NONE',  ( -85.40000000000000568, -30.80624999877096926, 101.7320508075688679 ) ) ;
#9105=CARTESIAN_POINT ( 'NONE',  ( 83.90000000000000568, -30.97500000000000142, 102.5980762113533018 ) ) ;
#9108=CARTESIAN_POINT ( 'NONE',  ( 85.40000000000000568, -32.23124999877096997, 101.7320508075688821 ) ) ;
#9109=CARTESIAN_POINT ( 'NONE',  ( 82.85293433256528317, -31.99999999999999289, -97.19890519203640622 ) ) ;
#9110=VECTOR ( 'NONE', #13072, 1000.000000000000000 ) ;
#9113=CARTESIAN_POINT ( 'NONE',  ( 85.15643035625001289, -32.39062499938548711, -99.99999999999998579 ) ) ;
#9114=ORIENTED_EDGE ( 'NONE', *, *, #7252, .F. ) ;
#9116=CARTESIAN_POINT ( 'NONE',  ( -79.64356964374998427, -34.82812499938548711, 98.40857419181659793 ) ) ;
#9117=CARTESIAN_POINT ( 'NONE',  ( 82.39999999999999147, -32.27812499938548285, -103.1828516163667899 ) ) ;
#9118=DIRECTION ( 'NONE',  ( 0.000000000000000000, 0.000000000000000000, 1.000000000000000000 ) ) ;
#9121=CARTESIAN_POINT ( 'NONE',  ( -85.15643035625001289, -35.09062499938548285, 99.99999999999998579 ) ) ;
#9122=ADVANCED_FACE ( 'NONE', ( #11749 ), #13309, .T. ) ;
#9123=EDGE_LOOP ( 'NONE', ( #3305, #16935, #18701, #14491 ) ) ;
#9124=CARTESIAN_POINT ( 'NONE',  ( -85.23110191009446623, -35.00000000000000000, 99.14248198118166044 ) ) ;
#9132=CARTESIAN_POINT ( 'NONE',  ( 81.02178482187500208, -30.74062499938548498, 102.3871387122750889 ) ) ;
#9133=LINE ( 'NONE', #1533, #247 ) ;
#9135=CARTESIAN_POINT ( 'NONE',  ( -84.82992844608099858, -32.00000000000000000, -101.3134070403134928 ) ) ;
#9136=CARTESIAN_POINT ( 'NONE',  ( -81.02178482187500208, -32.35312499938548569, -97.61286128772489690 ) ) ;
#9137=AXIS2_PLACEMENT_3D ( 'NONE', #14062, #16811, #12499 ) ;
#9139=CARTESIAN_POINT ( 'NONE',  ( 83.90000000000000568, -35.26874999877097139, 97.40192378864668399 ) ) ;
#9140=CARTESIAN_POINT ( 'NONE',  ( 83.90000000000000568, -34.51874999877097139, 102.5980762113533018 ) ) ;
#9141=CARTESIAN_POINT ( 'NONE',  ( -94.79999999999999716, -3.000000000000000000, 150.0000000000000000 ) ) ;
#9142=CARTESIAN_POINT ( 'NONE',  ( -81.02178482187500208, -32.20312499938548711, 97.61286128772489690 ) ) ;
#9145=CARTESIAN_POINT ( 'NONE',  ( -82.39999999999999147, -30.56250000000000355, -103.4641016151377499 ) ) ;
#9147=CARTESIAN_POINT ( 'NONE',  ( 82.65333140691205926, -34.99995246259152282, -97.01071553687880566 ) ) ;
#9149=CARTESIAN_POINT ( 'NONE',  ( -79.64356964375001269, -33.66562499938549280, -98.40857419181659793 ) ) ;
#9153=ORIENTED_EDGE ( 'NONE', *, *, #16494, .F. ) ;
#9155=CARTESIAN_POINT ( 'NONE',  ( -82.40000000000000568, -33.43124999877096570, 102.9999999999999858 ) ) ;
#9156=CARTESIAN_POINT ( 'NONE',  ( 82.39999999999999147, -33.85312499938548569, 103.1828516163667899 ) ) ;
#9160=CARTESIAN_POINT ( 'NONE',  ( 80.90000000000000568, -33.69374999877096855, -97.40192378864668399 ) ) ;
#9177=CARTESIAN_POINT ( 'NONE',  ( -85.15643035624999868, -34.71562499938548285, 101.5914258081833879 ) ) ;
#9184=DIRECTION ( 'NONE',  ( -0.000000000000000000, -1.000000000000000000, -0.000000000000000000 ) ) ;
#9187=EDGE_CURVE ( 'NONE', #4798, #15307, #6674, .T. ) ;
#9188=CARTESIAN_POINT ( 'NONE',  ( -83.77821517812500929, -32.91562499938547859, -102.3871387122750889 ) ) ;
#9191=DIRECTION ( 'NONE',  ( 0.000000000000000000, 1.000000000000000000, 0.000000000000000000 ) ) ;
#9196=CARTESIAN_POINT ( 'NONE',  ( -83.09162395290292125, -32.00000000000000711, 102.7516965079135787 ) ) ;
#9198=CARTESIAN_POINT ( 'NONE',  ( -85.40000000000000568, -30.84374999877096712, 99.99999999999998579 ) ) ;
#9199=CARTESIAN_POINT ( 'NONE',  ( 83.90000000000000568, -31.42500000000000071, 102.5980762113533018 ) ) ;
#9202=CARTESIAN_POINT ( 'NONE',  ( 85.15643035625001289, -32.95312499938548711, -99.99999999999998579 ) ) ;
#9203=CARTESIAN_POINT ( 'NONE',  ( 82.40000000000000568, -30.00000000000000355, 99.99999999999998579 ) ) ;
#9204=CARTESIAN_POINT ( 'NONE',  ( 81.02178482187500208, -34.94062499938548427, -102.3871387122750889 ) ) ;
#9207=CARTESIAN_POINT ( 'NONE',  ( 83.77821517812500929, -32.91562499938547859, -97.61286128772489690 ) ) ;
#9208=CARTESIAN_POINT ( 'NONE',  ( 79.64356964375001269, -32.65312499938548285, -101.5914258081833879 ) ) ;
#9209=DIRECTION ( 'NONE',  ( 0.000000000000000000, -1.000000000000000000, 0.000000000000000000 ) ) ;
#9212=CARTESIAN_POINT ( 'NONE',  ( -80.90000000000000568, -30.60000000000000142, 97.40192378864668399 ) ) ;
#9213=ORIENTED_EDGE ( 'NONE', *, *, #14147, .T. ) ;
#9216=AXIS2_PLACEMENT_3D ( 'NONE', #6818, #5638, #16079 ) ;
#9218=CARTESIAN_POINT ( 'NONE',  ( 83.77821517812500929, -30.51562499938548711, 97.61286128772489690 ) ) ;
#9219=( BOUNDED_CURVE ( )  B_SPLINE_CURVE ( 2, ( #6773, #18493, #11054, #2072, #16928, #9494, #9395, #2358, #3633 ),
 .UNSPECIFIED., .F., .F. ) 
 B_SPLINE_CURVE_WITH_KNOTS ( ( 3, 2, 2, 2, 3 ),
 ( 0.5208333333333334814, 0.5277777777777777901, 0.5416666666666666297, 0.5555555555555555802, 0.5625000000000000000 ),
 .UNSPECIFIED. ) 
 CURVE ( )  GEOMETRIC_REPRESENTATION_ITEM ( )  RATIONAL_B_SPLINE_CURVE ( ( 0.9330127018922194093, 0.9330127018922209636, 1.000000000000000000, 0.8660254037844387076, 1.000000000000000000, 0.8660254037844387076, 1.000000000000000000, 0.9330127018922194093, 0.9330127018922194093 ) ) 
 REPRESENTATION_ITEM ( '' )  );
#9222=CARTESIAN_POINT ( 'NONE',  ( -79.39999999999999147, -32.43750000000000000, 98.26794919243110371 ) ) ;
#9223=CARTESIAN_POINT ( 'NONE',  ( 83.77821517812500929, -34.82812499938548711, 102.3871387122750889 ) ) ;
#9225=CARTESIAN_POINT ( 'NONE',  ( 81.02178482187500208, -31.30312499938548498, -97.61286128772489690 ) ) ;
#9227=CARTESIAN_POINT ( 'NONE',  ( -85.03799702444354125, -32.00000000000001421, -100.8187845449568130 ) ) ;
#9228=CARTESIAN_POINT ( 'NONE',  ( -83.77821517812500929, -34.82812499938548711, -102.3871387122750889 ) ) ;
#9229=CIRCLE ( 'NONE', #17362, 3.000000000000002665 ) ;
#9232=CARTESIAN_POINT ( 'NONE',  ( 82.39999999999999147, -35.23124999877096997, 96.53589838486223584 ) ) ;
#9235=CARTESIAN_POINT ( 'NONE',  ( -81.02178482187500208, -32.65312499938548996, 97.61286128772489690 ) ) ;
#9238=EDGE_CURVE ( 'NONE', #3130, #4798, #15968, .T. ) ;
#9239=CARTESIAN_POINT ( 'NONE',  ( -83.90000000000000568, -31.72500000000000142, -97.40192378864668399 ) ) ;
#9240=EDGE_CURVE ( 'NONE', #4006, #5317, #17425, .T. ) ;
#9241=CARTESIAN_POINT ( 'NONE',  ( 85.40000000000000568, -34.01250000000000284, -101.7320508075688679 ) ) ;
#9243=LINE ( 'NONE', #18437, #12353 ) ;
#9244=EDGE_CURVE ( 'NONE', #6950, #15931, #10674, .T. ) ;
#9245=DIRECTION ( 'NONE',  ( 4.625929269271494788E-16, 1.000000000000000000, -0.000000000000000000 ) ) ;
#9248=VERTEX_POINT ( 'NONE', #1875 ) ;
#9251=CARTESIAN_POINT ( 'NONE',  ( 81.02178482187500208, -33.44062499938548427, 102.3871387122750889 ) ) ;
#9252=CARTESIAN_POINT ( 'NONE',  ( 80.90000000000000568, -34.20000000000000284, 102.5980762113533018 ) ) ;
#9254=CARTESIAN_POINT ( 'NONE',  ( 82.39999999999999147, -34.33124999877097139, -103.4641016151377499 ) ) ;
#9255=CARTESIAN_POINT ( 'NONE',  ( 82.40000000000000568, -34.78124999877096712, 96.99999999999998579 ) ) ;
#9256=CARTESIAN_POINT ( 'NONE',  ( -79.64356964374999848, -33.06562499938548427, -99.99999999999998579 ) ) ;
#9266=CARTESIAN_POINT ( 'NONE',  ( -83.77821517812500929, -30.21562499938548285, -102.3871387122750889 ) ) ;
#9268=CARTESIAN_POINT ( 'NONE',  ( -85.40000000000000568, -34.01250000000000284, -98.26794919243111792 ) ) ;
#9273=( BOUNDED_CURVE ( )  B_SPLINE_CURVE ( 2, ( #11722, #12999, #17500, #13383, #7042, #17, #3023, #11823, #17792 ),
 .UNSPECIFIED., .F., .F. ) 
 B_SPLINE_CURVE_WITH_KNOTS ( ( 3, 2, 2, 2, 3 ),
 ( 0.3125000000000001665, 0.3194444444444444198, 0.3333333333333333148, 0.3472222222222222099, 0.3541666666666666297 ),
 .UNSPECIFIED. ) 
 CURVE ( )  GEOMETRIC_REPRESENTATION_ITEM ( )  RATIONAL_B_SPLINE_CURVE ( ( 0.9330127018922194093, 0.9330127018922209636, 1.000000000000000000, 0.8660254037844387076, 1.000000000000000000, 0.8660254037844387076, 1.000000000000000000, 0.9330127018922196314, 0.9330127018922194093 ) ) 
 REPRESENTATION_ITEM ( '' )  );
#9278=CARTESIAN_POINT ( 'NONE',  ( -82.40000000000000568, -33.71249999999998437, 96.99999999999998579 ) ) ;
#9279=DIRECTION ( 'NONE',  ( 0.000000000000000000, -1.000000000000000000, 0.000000000000000000 ) ) ;
#9283=ORIENTED_EDGE ( 'NONE', *, *, #18203, .F. ) ;
#9284=CARTESIAN_POINT ( 'NONE',  ( -85.15643035624999868, -33.70312499938548711, -98.40857419181659793 ) ) ;
#9288=CARTESIAN_POINT ( 'NONE',  ( 83.03192786677293213, -35.00000000000000000, -102.6890373435400221 ) ) ;
#9294=ORIENTED_EDGE ( 'NONE', *, *, #6043, .T. ) ;
#9296=CARTESIAN_POINT ( 'NONE',  ( 80.90000000000000568, -31.20000000000000284, -102.5980762113533018 ) ) ;
#9297=CARTESIAN_POINT ( 'NONE',  ( -82.39999999999999147, -33.43124999877097281, 103.4641016151377499 ) ) ;
#9298=CARTESIAN_POINT ( 'NONE',  ( 79.39999999999999147, -32.92500000000000426, 99.99999999999998579 ) ) ;
#9300=CARTESIAN_POINT ( 'NONE',  ( -79.79666399293490997, -31.99999999999999289, -98.51078102784448731 ) ) ;
#9302=CARTESIAN_POINT ( 'NONE',  ( 79.64356964374999848, -33.17812499938548854, -99.99999999999998579 ) ) ;
#9303=VECTOR ( 'NONE', #6776, 1000.000000000000000 ) ;
#9306=CARTESIAN_POINT ( 'NONE',  ( 85.15643035624999868, -34.15312499938548285, -101.5914258081833879 ) ) ;
#9307=ORIENTED_EDGE ( 'NONE', *, *, #16365, .F. ) ;
#9309=CARTESIAN_POINT ( 'NONE',  ( -79.39999999999999147, -34.68750000000000000, 98.26794919243110371 ) ) ;
#9311=CARTESIAN_POINT ( 'NONE',  ( 83.90000000000000568, -33.67500000000000426, 102.5980762113533018 ) ) ;
#9314=CARTESIAN_POINT ( 'NONE',  ( -79.64356964375001269, -34.82812499938548711, 98.40857419181659793 ) ) ;
#9317=CARTESIAN_POINT ( 'NONE',  ( -79.39999999999999147, -34.23750000000000426, 98.26794919243110371 ) ) ;
#9321=CARTESIAN_POINT ( 'NONE',  ( -94.79999999999999716, -5.200000000000000178, -150.0000000000000000 ) ) ;
#9322=CARTESIAN_POINT ( 'NONE',  ( 85.15643035624999868, -31.00312499938548072, 98.40857419181659793 ) ) ;
#9323=CARTESIAN_POINT ( 'NONE',  ( 85.15643035624999868, -31.19062499938548783, -98.40857419181659793 ) ) ;
#9325=CARTESIAN_POINT ( 'NONE',  ( -82.39999999999999147, -34.86562499938548854, 96.81714838363319586 ) ) ;
#9326=CARTESIAN_POINT ( 'NONE',  ( -85.15643035625001289, -32.95312499938548711, -99.99999999999998579 ) ) ;
#9328=CARTESIAN_POINT ( 'NONE',  ( 82.39999999999999147, -31.04062499938548569, 96.81714838363319586 ) ) ;
#9331=CARTESIAN_POINT ( 'NONE',  ( -85.15643035624999868, -32.99062499938548854, 98.40857419181659793 ) ) ;
#9334=CARTESIAN_POINT ( 'NONE',  ( -83.90000000000000568, -31.27500000000000568, -97.40192378864668399 ) ) ;
#9335=EDGE_CURVE ( 'NONE', #7020, #5172, #18487, .T. ) ;
#9336=( BOUNDED_SURFACE ( )  B_SPLINE_SURFACE ( 1, 2, ( 
 ( #11692, #11315, #8761, #14713, #15812, #1351, #12873, #18144, #13537, #7779, #12078, #2901, #17763, #1437, #16291, #15106, #18055, #4466, #16672, #7492, #11793, #4766, #83, #1720, #8856, #7587, #14811, #11983, #179, #12176, #10420, #16384, #2993, #277, #5840, #10518, #3183, #11884, #7392, #14917, #8949, #10707, #1633, #1544, #3278, #4370, #6128, #13355, #13447, #13305, #16486, #5937, #9142, #17855, #10614, #7678, #6034, #15199, #17951, #4561, #3088, #9049, #4664, #13632, #9235, #15013, #16580, #6228, #1817, #13733, #10329, #5244, #10899, #9331, #18430, #9531, #3382, #2109, #12557, #8166, #560, #2297, #15296, #5142, #14115, #12370, #16866, #5049, #14024, #13824, #18526, #12654, #10801, #3472, #8070, #18239, #18336, #18626, #8262, #6414, #15398, #9432, #659, #4957, #2008, #15693, #11089, #7968, #13922, #752, #372, #6518, #12460, #10994, #6324, #17058, #16960, #11193, #16765, #17156, #3764, #3571, #9729, #6607, #6707, #12276, #15597, #9636, #3671, #4857, #466, #1909, #7873, #15496, #2205 ),
 ( #17450, #8545, #9824, #17542, #15788, #11287, #18824, #5446, #6994, #10021, #19013, #12852, #4061, #1041, #11484, #9926, #2395, #5633, #949, #17257, #15887, #14402, #3862, #12945, #15980, #14496, #17350, #10118, #5347, #2584, #1129, #8357, #6904, #2492, #18917, #14311, #7086, #13042, #18726, #11384, #5536, #6811, #3960, #11579, #16073, #8450, #4160, #14211, #848, #12757, #2077, #8324, #17128, #630, #18402, #819, #916, #3543, #5022, #9499, #14280, #9698, #11058, #3825, #3446, #5315, #9795, #10963, #15756, #14087, #6777, #2363, #8235, #2267, #18595, #11256, #12434, #12338, #18304, #15660, #14183, #17220, #725, #4924, #5212, #9401, #10869, #7938, #15363, #12727, #11159, #16931, #16840, #13991, #1981, #13889, #6578, #18699, #527, #6680, #6482, #18497, #12623, #15466, #8033, #12526, #5118, #17028, #3639, #9601, #15565, #2178, #8135, #3733, #9991, #13197, #2642, #17419, #5781, #18786, #1196, #12916, #14660, #14758, #5605, #12821, #16139, #1295, #13103, #4031, #18884, #15947, #5506, #11453, #6874 ) ),
 .UNSPECIFIED., .F., .F., .F. ) 
 B_SPLINE_SURFACE_WITH_KNOTS ( ( 2, 2 ),
 ( 3, 2, 2, 2, 2, 2, 2, 2, 2, 2, 2, 2, 2, 2, 2, 2, 2, 2, 2, 2, 2, 2, 2, 2, 2, 2, 2, 2, 2, 2, 2, 2, 2, 2, 2, 2, 2, 2, 2, 2, 2, 2, 2, 2, 2, 2, 2, 2, 2, 2, 2, 2, 2, 2, 2, 2, 2, 2, 2, 2, 2, 2, 2, 2, 2, 2, 2, 3 ),
 ( 0.000000000000000000, 1.000000000000000000 ),
 ( 0.000000000000000000, 0.01388888888888888812, 0.02777777777777777624, 0.04166666666666666435, 0.05555555555555555247, 0.06944444444444444753, 0.08333333333333332871, 0.09722222222222222376, 0.1111111111111111049, 0.1250000000000000000, 0.1388888888888888951, 0.1527777777777777901, 0.1666666666666666574, 0.1805555555555555525, 0.1944444444444444475, 0.2083333333333333426, 0.2222222222222222099, 0.2361111111111111049, 0.2500000000000000000, 0.2638888888888888951, 0.2777777777777777901, 0.2916666666666666852, 0.3055555555555555802, 0.3194444444444444198, 0.3333333333333333148, 0.3472222222222222099, 0.3611111111111111049, 0.3750000000000000000, 0.3888888888888888951, 0.4027777777777777901, 0.4166666666666666852, 0.4305555555555555802, 0.4444444444444444198, 0.4583333333333333148, 0.4722222222222222099, 0.4861111111111111049, 0.5000000000000000000, 0.5138888888888888395, 0.5277777777777777901, 0.5416666666666666297, 0.5555555555555555802, 0.5694444444444444198, 0.5833333333333333703, 0.5972222222222222099, 0.6111111111111111605, 0.6250000000000000000, 0.6388888888888888395, 0.6527777777777777901, 0.6666666666666666297, 0.6805555555555555802, 0.6944444444444444198, 0.7083333333333333703, 0.7222222222222222099, 0.7361111111111111605, 0.7500000000000000000, 0.7638888888888888395, 0.7777777777777777901, 0.7916666666666666297, 0.8055555555555555802, 0.8194444444444444198, 0.8333333333333333703, 0.8472222222222222099, 0.8611111111111111605, 0.8750000000000000000, 0.8888888888888888395, 0.9027777777777777901, 0.9166666666666666297, 0.9258785565094813652 ),
 .UNSPECIFIED. ) 
 GEOMETRIC_REPRESENTATION_ITEM ( )  RATIONAL_B_SPLINE_SURFACE ( (
 ( 1.000000000000000000, 0.8660254037844387076, 1.000000000000000000, 0.8660254037844387076, 1.000000000000000000, 0.8660254037844387076, 1.000000000000000000, 0.8660254037844387076, 1.000000000000000000, 0.8660254037844387076, 1.000000000000000000, 0.8660254037844387076, 1.000000000000000000, 0.8660254037844387076, 1.000000000000000000, 0.8660254037844387076, 1.000000000000000000, 0.8660254037844387076, 1.000000000000000000, 0.8660254037844387076, 1.000000000000000000, 0.8660254037844387076, 1.000000000000000000, 0.8660254037844387076, 1.000000000000000000, 0.8660254037844387076, 1.000000000000000000, 0.8660254037844387076, 1.000000000000000000, 0.8660254037844387076, 1.000000000000000000, 0.8660254037844387076, 1.000000000000000000, 0.8660254037844387076, 1.000000000000000000, 0.8660254037844387076, 1.000000000000000000, 0.8660254037844387076, 1.000000000000000000, 0.8660254037844387076, 1.000000000000000000, 0.8660254037844387076, 1.000000000000000000, 0.8660254037844387076, 1.000000000000000000, 0.8660254037844387076, 1.000000000000000000, 0.8660254037844387076, 1.000000000000000000, 0.8660254037844387076, 1.000000000000000000, 0.8660254037844387076, 1.000000000000000000, 0.8660254037844387076, 1.000000000000000000, 0.8660254037844387076, 1.000000000000000000, 0.8660254037844387076, 1.000000000000000000, 0.8660254037844387076, 1.000000000000000000, 0.8660254037844387076, 1.000000000000000000, 0.8660254037844387076, 1.000000000000000000, 0.8660254037844387076, 1.000000000000000000, 0.8660254037844387076, 1.000000000000000000, 0.8660254037844387076, 1.000000000000000000, 0.8660254037844387076, 1.000000000000000000, 0.8660254037844387076, 1.000000000000000000, 0.8660254037844387076, 1.000000000000000000, 0.8660254037844387076, 1.000000000000000000, 0.8660254037844387076, 1.000000000000000000, 0.8660254037844387076, 1.000000000000000000, 0.8660254037844387076, 1.000000000000000000, 0.8660254037844387076, 1.000000000000000000, 0.8660254037844387076, 1.000000000000000000, 0.8660254037844387076, 1.000000000000000000, 0.8660254037844387076, 1.000000000000000000, 0.8660254037844387076, 1.000000000000000000, 0.8660254037844387076, 1.000000000000000000, 0.8660254037844387076, 1.000000000000000000, 0.8660254037844387076, 1.000000000000000000, 0.8660254037844387076, 1.000000000000000000, 0.8660254037844387076, 1.000000000000000000, 0.8660254037844387076, 1.000000000000000000, 0.8660254037844387076, 1.000000000000000000, 0.8660254037844387076, 1.000000000000000000, 0.8660254037844387076, 1.000000000000000000, 0.8660254037844387076, 1.000000000000000000, 0.8660254037844387076, 1.000000000000000000, 0.8660254037844387076, 1.000000000000000000, 0.8660254037844387076, 1.000000000000000000, 0.8660254037844387076, 1.000000000000000000, 0.8660254037844387076, 1.000000000000000000, 0.8660254037844387076, 1.000000000000000000, 0.8660254037844387076, 1.000000000000000000, 0.8660254037844387076, 1.000000000000000000, 0.8660254037844387076, 1.000000000000000000, 0.9111405360107203144, 0.9401542295229963209),
 ( 1.000000000000000000, 0.8660254037844387076, 1.000000000000000000, 0.8660254037844387076, 1.000000000000000000, 0.8660254037844387076, 1.000000000000000000, 0.8660254037844387076, 1.000000000000000000, 0.8660254037844387076, 1.000000000000000000, 0.8660254037844387076, 1.000000000000000000, 0.8660254037844387076, 1.000000000000000000, 0.8660254037844387076, 1.000000000000000000, 0.8660254037844387076, 1.000000000000000000, 0.8660254037844387076, 1.000000000000000000, 0.8660254037844387076, 1.000000000000000000, 0.8660254037844387076, 1.000000000000000000, 0.8660254037844387076, 1.000000000000000000, 0.8660254037844387076, 1.000000000000000000, 0.8660254037844387076, 1.000000000000000000, 0.8660254037844387076, 1.000000000000000000, 0.8660254037844387076, 1.000000000000000000, 0.8660254037844387076, 1.000000000000000000, 0.8660254037844387076, 1.000000000000000000, 0.8660254037844387076, 1.000000000000000000, 0.8660254037844387076, 1.000000000000000000, 0.8660254037844387076, 1.000000000000000000, 0.8660254037844387076, 1.000000000000000000, 0.8660254037844387076, 1.000000000000000000, 0.8660254037844387076, 1.000000000000000000, 0.8660254037844387076, 1.000000000000000000, 0.8660254037844387076, 1.000000000000000000, 0.8660254037844387076, 1.000000000000000000, 0.8660254037844387076, 1.000000000000000000, 0.8660254037844387076, 1.000000000000000000, 0.8660254037844387076, 1.000000000000000000, 0.8660254037844387076, 1.000000000000000000, 0.8660254037844387076, 1.000000000000000000, 0.8660254037844387076, 1.000000000000000000, 0.8660254037844387076, 1.000000000000000000, 0.8660254037844387076, 1.000000000000000000, 0.8660254037844387076, 1.000000000000000000, 0.8660254037844387076, 1.000000000000000000, 0.8660254037844387076, 1.000000000000000000, 0.8660254037844387076, 1.000000000000000000, 0.8660254037844387076, 1.000000000000000000, 0.8660254037844387076, 1.000000000000000000, 0.8660254037844387076, 1.000000000000000000, 0.8660254037844387076, 1.000000000000000000, 0.8660254037844387076, 1.000000000000000000, 0.8660254037844387076, 1.000000000000000000, 0.8660254037844387076, 1.000000000000000000, 0.8660254037844387076, 1.000000000000000000, 0.8660254037844387076, 1.000000000000000000, 0.8660254037844387076, 1.000000000000000000, 0.8660254037844387076, 1.000000000000000000, 0.8660254037844387076, 1.000000000000000000, 0.8660254037844387076, 1.000000000000000000, 0.8660254037844387076, 1.000000000000000000, 0.8660254037844387076, 1.000000000000000000, 0.8660254037844387076, 1.000000000000000000, 0.8660254037844387076, 1.000000000000000000, 0.8660254037844387076, 1.000000000000000000, 0.8660254037844387076, 1.000000000000000000, 0.8660254037844387076, 1.000000000000000000, 0.8660254037844387076, 1.000000000000000000, 0.8660254037844387076, 1.000000000000000000, 0.8660254037844387076, 1.000000000000000000, 0.8660254037844387076, 1.000000000000000000, 0.8660254037844387076, 1.000000000000000000, 0.8660254037844387076, 1.000000000000000000, 0.9111405360107203144, 0.9401542295229963209) ) ) 
 REPRESENTATION_ITEM ( '' )  SURFACE ( )  );
#9338=CARTESIAN_POINT ( 'NONE',  ( 82.39999999999999147, -34.61250000000000426, -96.53589838486223584 ) ) ;
#9339=LINE ( 'NONE', #10807, #7029 ) ;
#9340=CARTESIAN_POINT ( 'NONE',  ( -83.77821517812500929, -35.12812499938548427, -97.61286128772489690 ) ) ;
#9348=CARTESIAN_POINT ( 'NONE',  ( 79.39999999999999147, -34.27499999999999858, 99.99999999999998579 ) ) ;
#9349=CARTESIAN_POINT ( 'NONE',  ( 85.40000000000000568, -32.73750000000000426, -98.26794919243111792 ) ) ;
#9350=CARTESIAN_POINT ( 'NONE',  ( 82.39999999999999147, -32.16562499938549280, -96.81714838363319586 ) ) ;
#9363=CARTESIAN_POINT ( 'NONE',  ( -80.60346964444562445, -32.00000000000000000, 97.67482724152021945 ) ) ;
#9364=LINE ( 'NONE', #15326, #1015 ) ;
#9365=ORIENTED_EDGE ( 'NONE', *, *, #18905, .T. ) ;
#9367=CARTESIAN_POINT ( 'NONE',  ( -83.90000000000000568, -33.16874999877096286, -102.5980762113533018 ) ) ;
#9371=CARTESIAN_POINT ( 'NONE',  ( 84.97511176746692740, -34.99999999999998579, -98.48300226792312628 ) ) ;
#9373=FACE_BOUND ( 'NONE', #29, .T. ) ;
#9376=VERTEX_POINT ( 'NONE', #6955 ) ;
#9383=CARTESIAN_POINT ( 'NONE',  ( 81.59615242270662350, -33.46740381056766722, 96.99999999999998579 ) ) ;
#9388=( BOUNDED_CURVE ( )  B_SPLINE_CURVE ( 2, ( #18026, #4733, #10679, #3249, #14685, #1320, #2157, #350, #1789 ),
 .UNSPECIFIED., .F., .F. ) 
 B_SPLINE_CURVE_WITH_KNOTS ( ( 3, 2, 2, 2, 3 ),
 ( 0.7291666666666668517, 0.7361111111111111605, 0.7500000000000000000, 0.7638888888888888395, 0.7708333333333332593 ),
 .UNSPECIFIED. ) 
 CURVE ( )  GEOMETRIC_REPRESENTATION_ITEM ( )  RATIONAL_B_SPLINE_CURVE ( ( 0.9330127018922194093, 0.9330127018922209636, 1.000000000000000000, 0.8660254037844387076, 1.000000000000000000, 0.8660254037844387076, 1.000000000000000000, 0.9330127018922198534, 0.9330127018922192983 ) ) 
 REPRESENTATION_ITEM ( '' )  );
#9389=CARTESIAN_POINT ( 'NONE',  ( -81.01744233620662783, -32.00000000000001421, 102.5835086888313015 ) ) ;
#9390=CARTESIAN_POINT ( 'NONE',  ( 83.90000000000000568, -30.37500000000000355, -102.5980762113533018 ) ) ;
#9392=CARTESIAN_POINT ( 'NONE',  ( -85.40000000000000568, -35.30624999877096570, 101.7320508075688679 ) ) ;
#9393=EDGE_CURVE ( 'NONE', #5172, #9425, #8278, .T. ) ;
#9395=CARTESIAN_POINT ( 'NONE',  ( -80.90000000000000568, -33.39374999877097139, 102.5980762113533018 ) ) ;
#9396=CARTESIAN_POINT ( 'NONE',  ( 79.39999999999999147, -33.31874999877096855, 99.99999999999998579 ) ) ;
#9397=( BOUNDED_CURVE ( )  B_SPLINE_CURVE ( 2, ( #8576, #3996, #11422, #883, #11607, #5377, #14341, #18949, #2431 ),
 .UNSPECIFIED., .F., .F. ) 
 B_SPLINE_CURVE_WITH_KNOTS ( ( 3, 2, 2, 2, 3 ),
 ( 0.7708333333333331483, 0.7777777777777777901, 0.7916666666666666297, 0.8055555555555555802, 0.8125000000000001110 ),
 .UNSPECIFIED. ) 
 CURVE ( )  GEOMETRIC_REPRESENTATION_ITEM ( )  RATIONAL_B_SPLINE_CURVE ( ( 0.9330127018922194093, 0.9330127018922177440, 1.000000000000000000, 0.8660254037844387076, 1.000000000000000000, 0.8660254037844387076, 1.000000000000000000, 0.9330127018922182991, 0.9330127018922194093 ) ) 
 REPRESENTATION_ITEM ( '' )  );
#9398=CARTESIAN_POINT ( 'NONE',  ( 82.39999999999999147, -33.51562499938548711, -96.81714838363319586 ) ) ;
#9401=CARTESIAN_POINT ( 'NONE',  ( -85.15643035624999868, -33.32812499938548001, 98.40857419181659793 ) ) ;
#9402=CARTESIAN_POINT ( 'NONE',  ( 81.02178482187500208, -34.79062499938548569, -97.61286128772489690 ) ) ;
#9406=CARTESIAN_POINT ( 'NONE',  ( 83.90000000000000568, -33.61874999877097281, -97.40192378864668399 ) ) ;
#9407=CARTESIAN_POINT ( 'NONE',  ( 85.40000000000000568, -33.56250000000000000, 98.26794919243111792 ) ) ;
#9410=CARTESIAN_POINT ( 'NONE',  ( -80.90000000000000568, -32.10000000000000142, 102.5980762113533018 ) ) ;
#9412=CARTESIAN_POINT ( 'NONE',  ( -85.10336890117802966, -34.99999999999999289, 100.9939266215828724 ) ) ;
#9414=CARTESIAN_POINT ( 'NONE',  ( 82.39999999999999147, -32.72812499938548569, 96.81714838363319586 ) ) ;
#9417=( BOUNDED_CURVE ( )  B_SPLINE_CURVE ( 2, ( #15207, #377, #17263, #2401, #17549 ),
 .UNSPECIFIED., .F., .F. ) 
 B_SPLINE_CURVE_WITH_KNOTS ( ( 3, 2, 3 ),
 ( 0.2975293541897461869, 0.3055555555555555802, 0.3125000000000001665 ),
 .UNSPECIFIED. ) 
 CURVE ( )  GEOMETRIC_REPRESENTATION_ITEM ( )  RATIONAL_B_SPLINE_CURVE ( ( 0.9346381638529985825, 0.9225778897267049583, 1.000000000000000000, 0.9330127018922177440, 0.9330127018922194093 ) ) 
 REPRESENTATION_ITEM ( '' )  );
#9419=CARTESIAN_POINT ( 'NONE',  ( 80.42036527867306006, -31.99999999999999289, 97.80162405160976391 ) ) ;
#9420=CARTESIAN_POINT ( 'NONE',  ( 79.64356964375001269, -35.01562499938548711, 98.40857419181659793 ) ) ;
#9421=CARTESIAN_POINT ( 'NONE',  ( 82.39999999999999147, -31.49062499938548854, -103.1828516163667899 ) ) ;
#9423=CARTESIAN_POINT ( 'NONE',  ( -79.64356964374999848, -34.07812499938548711, 99.99999999999998579 ) ) ;
#9424=CARTESIAN_POINT ( 'NONE',  ( -82.39999999999999147, -33.29062499938549280, -96.81714838363319586 ) ) ;
#9425=VERTEX_POINT ( 'NONE', #9785 ) ;
#9426=CARTESIAN_POINT ( 'NONE',  ( 85.15643035625001289, -33.85312499938549280, 99.99999999999998579 ) ) ;
#9430=CARTESIAN_POINT ( 'NONE',  ( -81.02178482187500208, -30.29062499938548569, 97.61286128772489690 ) ) ;
#9432=CARTESIAN_POINT ( 'NONE',  ( -79.64356964375001269, -34.04062499938549280, 98.40857419181659793 ) ) ;
#9435=CARTESIAN_POINT ( 'NONE',  ( -85.40000000000000568, -34.53750000000000142, -101.7320508075688679 ) ) ;
#9438=CARTESIAN_POINT ( 'NONE',  ( -79.64356964374999848, -34.97812499938548569, -99.99999999999998579 ) ) ;
#9442=CYLINDRICAL_SURFACE ( 'NONE', #15552, 3.000000000000002665 ) ;
#9443=DIRECTION ( 'NONE',  ( -1.000000000000000000, 4.625929269271494788E-16, 0.000000000000000000 ) ) ;
#9444=CARTESIAN_POINT ( 'NONE',  ( -82.40000000000000568, -33.03750000000000142, 102.9999999999999858 ) ) ;
#9445=CARTESIAN_POINT ( 'NONE',  ( 79.39999999999999147, -34.23750000000000426, 101.7320508075688963 ) ) ;
#9446=CIRCLE ( 'NONE', #13198, 2.649999999999982148 ) ;
#9447=CARTESIAN_POINT ( 'NONE',  ( -82.39999999999999147, -34.33124999877097139, 103.0000000000000000 ) ) ;
#9448=CARTESIAN_POINT ( 'NONE',  ( 79.64356964375001269, -30.96562499938548640, -101.5914258081833879 ) ) ;
#9451=FACE_OUTER_BOUND ( 'NONE', #6062, .T. ) ;
#9455=( BOUNDED_CURVE ( )  B_SPLINE_CURVE ( 2, ( #17294, #1168, #8394, #7216, #15826, #7127, #14439, #10255, #16216 ),
 .UNSPECIFIED., .F., .F. ) 
 B_SPLINE_CURVE_WITH_KNOTS ( ( 3, 2, 2, 2, 3 ),
 ( 0.6875000000000000000, 0.6944444444444444198, 0.7083333333333333703, 0.7222222222222222099, 0.7291666666666666297 ),
 .UNSPECIFIED. ) 
 CURVE ( )  GEOMETRIC_REPRESENTATION_ITEM ( )  RATIONAL_B_SPLINE_CURVE ( ( 0.9330127018922194093, 0.9330127018922194093, 1.000000000000000000, 0.8660254037844387076, 1.000000000000000000, 0.8660254037844387076, 1.000000000000000000, 0.9330127018922198534, 0.9330127018922192983 ) ) 
 REPRESENTATION_ITEM ( '' )  );
#9458=ORIENTED_EDGE ( 'NONE', *, *, #3170, .F. ) ;
#9462=DIRECTION ( 'NONE',  ( 1.000000000000000000, 0.000000000000000000, 0.000000000000000000 ) ) ;
#9465=CARTESIAN_POINT ( 'NONE',  ( -82.39999999999999147, -34.78124999877096712, -96.53589838486223584 ) ) ;
#9468=EDGE_CURVE ( 'NONE', #5107, #5933, #15297, .T. ) ;
#9478=CARTESIAN_POINT ( 'NONE',  ( -85.15643035624999868, -35.11426555956768425, -101.0032586025029815 ) ) ;
#9481=CARTESIAN_POINT ( 'NONE',  ( -80.90000000000000568, -33.45000000000000284, -97.40192378864668399 ) ) ;
#9483=CARTESIAN_POINT ( 'NONE',  ( 80.90000000000000568, -32.10000000000000142, 97.40192378864668399 ) ) ;
#9487=ORIENTED_EDGE ( 'NONE', *, *, #6998, .F. ) ;
#9489=CARTESIAN_POINT ( 'NONE',  ( 84.51155491706698797, -35.14114833091483803, -98.22820877610629964 ) ) ;
#9490=CARTESIAN_POINT ( 'NONE',  ( -82.40000000000000568, -30.00000000000000355, -99.99999999999998579 ) ) ;
#9492=CARTESIAN_POINT ( 'NONE',  ( -85.40000000000000568, -33.95624999877097139, 101.7320508075688679 ) ) ;
#9494=CARTESIAN_POINT ( 'NONE',  ( -79.39999999999999147, -33.35624999877096997, 101.7320508075688537 ) ) ;
#9497=CARTESIAN_POINT ( 'NONE',  ( 81.02178482187500208, -34.15312499938548285, -102.3871387122750889 ) ) ;
#9499=CARTESIAN_POINT ( 'NONE',  ( -85.15643035624999868, -32.35312499938549280, 101.5914258081833879 ) ) ;
#9500=CARTESIAN_POINT ( 'NONE',  ( 79.64356964374999848, -34.41562499938548569, -99.99999999999998579 ) ) ;
#9503=CARTESIAN_POINT ( 'NONE',  ( -79.39999999999999147, -33.78750000000000142, 98.26794919243110371 ) ) ;
#9510=CARTESIAN_POINT ( 'NONE',  ( -82.39999999999999147, -32.58750000000000568, 103.4641016151377499 ) ) ;
#9512=CARTESIAN_POINT ( 'NONE',  ( -94.79999999999999716, -32.00000000000000000, -150.0000000000000000 ) ) ;
#9513=( BOUNDED_CURVE ( )  B_SPLINE_CURVE ( 2, ( #8083, #9649, #6240, #4778, #3290, #15215, #18253, #1831, #6336 ),
 .UNSPECIFIED., .F., .F. ) 
 B_SPLINE_CURVE_WITH_KNOTS ( ( 3, 2, 2, 2, 3 ),
 ( 0.3958333333333334259, 0.4027777777777777901, 0.4166666666666666852, 0.4305555555555555802, 0.4375000000000000555 ),
 .UNSPECIFIED. ) 
 CURVE ( )  GEOMETRIC_REPRESENTATION_ITEM ( )  RATIONAL_B_SPLINE_CURVE ( ( 0.9330127018922192983, 0.9330127018922200755, 1.000000000000000000, 0.8660254037844387076, 1.000000000000000000, 0.8660254037844387076, 1.000000000000000000, 0.9330127018922187432, 0.9330127018922192983 ) ) 
 REPRESENTATION_ITEM ( '' )  );
#9515=CARTESIAN_POINT ( 'NONE',  ( 83.77821517812500929, -32.31562499938548427, 97.61286128772489690 ) ) ;
#9520=CARTESIAN_POINT ( 'NONE',  ( -79.64356964374998427, -32.69062499938548427, -101.5914258081833879 ) ) ;
#9521=CARTESIAN_POINT ( 'NONE',  ( 82.39999999999999147, -30.47812499938548569, 96.81714838363319586 ) ) ;
#9522=CARTESIAN_POINT ( 'NONE',  ( 85.15643035625001289, -31.15312499938548996, -99.99999999999998579 ) ) ;
#9524=CARTESIAN_POINT ( 'NONE',  ( -79.64356964374998427, -33.21562499938548996, 101.5914258081833879 ) ) ;
#9525=CARTESIAN_POINT ( 'NONE',  ( -85.15643035624999868, -33.36562499938548854, -98.40857419181659793 ) ) ;
#9526=ORIENTED_EDGE ( 'NONE', *, *, #2437, .T. ) ;
#9527=CARTESIAN_POINT ( 'NONE',  ( 81.02178482187500208, -32.65312499938548996, 102.3871387122750889 ) ) ;
#9530=CARTESIAN_POINT ( 'NONE',  ( -85.15643035625001289, -31.49062499938548498, 99.99999999999998579 ) ) ;
#9531=CARTESIAN_POINT ( 'NONE',  ( -82.39999999999999147, -33.06562499938548427, 96.81714838363319586 ) ) ;
#9534=CARTESIAN_POINT ( 'NONE',  ( -79.39999999999999147, -33.86250000000000426, -98.26794919243113213 ) ) ;
#9537=CARTESIAN_POINT ( 'NONE',  ( -83.77821517812500929, -34.67812499938548854, -97.61286128772489690 ) ) ;
#9540=ORIENTED_EDGE ( 'NONE', *, *, #10001, .T. ) ;
#9544=CARTESIAN_POINT ( 'NONE',  ( 94.79999999999995453, -32.00000000000000000, -150.0000000000000000 ) ) ;
#9547=CARTESIAN_POINT ( 'NONE',  ( 79.64356964375001269, -31.34062499938548640, -98.40857419181659793 ) ) ;
#9548=DIRECTION ( 'NONE',  ( 0.000000000000000000, -1.000000000000000000, 0.000000000000000000 ) ) ;
#9549=ORIENTED_EDGE ( 'NONE', *, *, #1020, .T. ) ;
#9550=CARTESIAN_POINT ( 'NONE',  ( 82.39999999999999147, -31.18124999877096926, 96.53589838486223584 ) ) ;
#9556=CARTESIAN_POINT ( 'NONE',  ( -83.90000000000000568, -34.87500000000000000, 102.5980762113533018 ) ) ;
#9559=CARTESIAN_POINT ( 'NONE',  ( -79.64356964375001269, -30.77812499938548285, -101.5914258081833879 ) ) ;
#9560=CIRCLE ( 'NONE', #12055, 5.199999999999996625 ) ;
#9561=CARTESIAN_POINT ( 'NONE',  ( 83.20384757729335945, -33.05759618943233136, 96.99999999999998579 ) ) ;
#9562=VERTEX_POINT ( 'NONE', #14549 ) ;
#9563=CARTESIAN_POINT ( 'NONE',  ( 79.64356964374998427, -34.56562499938548427, 98.40857419181659793 ) ) ;
#9564=CARTESIAN_POINT ( 'NONE',  ( -85.40000000000000568, -33.54374999877096286, -99.99999999999998579 ) ) ;
#9571=CARTESIAN_POINT ( 'NONE',  ( -80.90000000000000568, -34.29374999877096997, 102.5980762113533018 ) ) ;
#9575=CARTESIAN_POINT ( 'NONE',  ( 85.15643035625001289, -33.32812499938548711, -98.40857419181659793 ) ) ;
#9577=CARTESIAN_POINT ( 'NONE',  ( -82.39999999999999147, -34.52812499938548996, -96.81714838363319586 ) ) ;
#9586=EDGE_CURVE ( 'NONE', #11098, #10346, #7432, .T. ) ;
#9589=CARTESIAN_POINT ( 'NONE',  ( 79.39999999999999147, -33.31874999877096855, -99.99999999999998579 ) ) ;
#9590=CARTESIAN_POINT ( 'NONE',  ( 85.40000000000000568, -30.00000000000000355, -99.99999999999998579 ) ) ;
#9594=CARTESIAN_POINT ( 'NONE',  ( -85.40000000000000568, -34.93124999877096570, 98.26794919243111792 ) ) ;
#9597=CARTESIAN_POINT ( 'NONE',  ( 82.40000000000000568, -30.00000000000000355, 103.0000000000000000 ) ) ;
#9598=CARTESIAN_POINT ( 'NONE',  ( 85.15643035625001289, -32.46562499938548996, -101.5914258081833879 ) ) ;
#9600=CARTESIAN_POINT ( 'NONE',  ( -79.39999999999999147, -33.76874999877097139, 99.99999999999998579 ) ) ;
#9601=CARTESIAN_POINT ( 'NONE',  ( -85.15643035624999868, -34.22812499938547859, 98.40857419181659793 ) ) ;
#9602=CARTESIAN_POINT ( 'NONE',  ( 79.64356964374999848, -32.61562499938548854, -99.99999999999998579 ) ) ;
#9605=CARTESIAN_POINT ( 'NONE',  ( -85.40000000000000568, -33.56250000000000000, 101.7320508075688679 ) ) ;
#9606=VECTOR ( 'NONE', #11642, 1000.000000000000000 ) ;
#9607=EDGE_CURVE ( 'NONE', #17054, #16462, #2225, .T. ) ;
#9609=CARTESIAN_POINT ( 'NONE',  ( 83.20384757729337366, -33.50759618943233420, 97.00000000000000000 ) ) ;
#9611=EDGE_CURVE ( 'NONE', #13408, #5861, #3025, .T. ) ;
#9613=EDGE_CURVE ( 'NONE', #14621, #729, #13478, .T. ) ;
#9614=CARTESIAN_POINT ( 'NONE',  ( -83.90000000000000568, -32.77499999999999858, 97.40192378864668399 ) ) ;
#9616=ORIENTED_EDGE ( 'NONE', *, *, #9613, .T. ) ;
#9618=AXIS2_PLACEMENT_3D ( 'NONE', #4767, #14025, #15298 ) ;
#9619=CARTESIAN_POINT ( 'NONE',  ( 83.20395887649176814, -35.00000000000001421, 97.36341917746361219 ) ) ;
#9620=CARTESIAN_POINT ( 'NONE',  ( 79.64356964374999848, -33.51562499938548711, 99.99999999999998579 ) ) ;
#9621=AXIS2_PLACEMENT_3D ( 'NONE', #14576, #8434, #1109 ) ;
#9624=CARTESIAN_POINT ( 'NONE',  ( -82.39999999999999147, -32.61562499938548854, -103.1828516163667899 ) ) ;
#9625=CARTESIAN_POINT ( 'NONE',  ( 85.15643035624999868, -32.42812499938548854, 101.5914258081833879 ) ) ;
#9626=CARTESIAN_POINT ( 'NONE',  ( 81.02178482187500208, -31.45312499938549067, -102.3871387122750889 ) ) ;
#9628=CARTESIAN_POINT ( 'NONE',  ( -83.77821517812500929, -33.77812499938548285, 102.3871387122750889 ) ) ;
#9629=CARTESIAN_POINT ( 'NONE',  ( -79.64356964374999848, -34.07812499938548711, -99.99999999999998579 ) ) ;
#9631=CARTESIAN_POINT ( 'NONE',  ( 79.64356964374999848, -33.17812499938548854, 99.99999999999998579 ) ) ;
#9635=CARTESIAN_POINT ( 'NONE',  ( -83.77821517812500929, -31.86562499938548498, 102.3871387122750889 ) ) ;
#9636=CARTESIAN_POINT ( 'NONE',  ( -79.64356964375001269, -35.01562499938548711, 101.5914258081833879 ) ) ;
#9641=CARTESIAN_POINT ( 'NONE',  ( -82.39999999999999147, -32.58750000000000568, -96.53589838486223584 ) ) ;
#9643=DIRECTION ( 'NONE',  ( 1.000000000000000000, 0.000000000000000000, 0.000000000000000000 ) ) ;
#9649=CARTESIAN_POINT ( 'NONE',  ( 83.20384757729337366, -32.15759618943233278, 97.00000000000000000 ) ) ;
#9651=CARTESIAN_POINT ( 'NONE',  ( 79.64356964375001269, -30.96562499938548640, 98.40857419181659793 ) ) ;
#9652=CARTESIAN_POINT ( 'NONE',  ( -69.99999999999998579, -35.00000000000000000, 150.0000000000000000 ) ) ;
#9653=CARTESIAN_POINT ( 'NONE',  ( 83.77821517812500929, -31.67812499938548498, -97.61286128772489690 ) ) ;
#9654=CARTESIAN_POINT ( 'NONE',  ( 82.40000000000000568, -34.61250000000001137, 102.9999999999999858 ) ) ;
#9655=ORIENTED_EDGE ( 'NONE', *, *, #1928, .F. ) ;
#9656=CARTESIAN_POINT ( 'NONE',  ( 80.90000000000000568, -31.89374999877096784, 102.5980762113533018 ) ) ;
#9657=PRODUCT_CONTEXT ( 'NONE', #11203, 'mechanical' ) ;
#9662=ORIENTED_EDGE ( 'NONE', *, *, #11128, .F. ) ;
#9664=CARTESIAN_POINT ( 'NONE',  ( -85.15643035625001289, -31.94062499938548427, -99.99999999999998579 ) ) ;
#9667=CARTESIAN_POINT ( 'NONE',  ( 79.64356964374998427, -33.66562499938548569, 98.40857419181659793 ) ) ;
#9668=CARTESIAN_POINT ( 'NONE',  ( -79.39999999999999147, -32.90624999877096712, -98.26794919243113213 ) ) ;
#9669=CARTESIAN_POINT ( 'NONE',  ( 82.39999999999999147, -33.71249999999999858, 103.4641016151377499 ) ) ;
#9673=CARTESIAN_POINT ( 'NONE',  ( 85.23110191008899506, -34.99999999999998579, -99.14248198115983257 ) ) ;
#9675=CARTESIAN_POINT ( 'NONE',  ( 80.90000000000000568, -30.54374999877096997, -97.40192378864668399 ) ) ;
#9678=CARTESIAN_POINT ( 'NONE',  ( 85.15643035625001289, -33.70312499938548711, -101.5914258081833879 ) ) ;
#9687=LINE ( 'NONE', #903, #8483 ) ;
#9690=CARTESIAN_POINT ( 'NONE',  ( 79.64356964375001269, -34.82812499938548711, -98.40857419181659793 ) ) ;
#9692=CARTESIAN_POINT ( 'NONE',  ( -80.90000000000000568, -33.24374999877097281, 97.40192378864668399 ) ) ;
#9696=CARTESIAN_POINT ( 'NONE',  ( 85.40000000000000568, -33.99374999877097281, 99.99999999999998579 ) ) ;
#9698=CARTESIAN_POINT ( 'NONE',  ( -85.15643035624999868, -32.42812499938548854, 98.40857419181659793 ) ) ;
#9701=CARTESIAN_POINT ( 'NONE',  ( 79.39999999999999147, -32.92500000000000426, 99.99999999999998579 ) ) ;
#9702=CARTESIAN_POINT ( 'NONE',  ( -79.39999999999999147, -33.82500000000000284, 99.99999999999998579 ) ) ;
#9709=ORIENTED_EDGE ( 'NONE', *, *, #8289, .T. ) ;
#9710=LINE ( 'NONE', #9905, #12541 ) ;
#9711=CARTESIAN_POINT ( 'NONE',  ( 81.44948931429641448, -35.00000000000001421, 97.40655328406457159 ) ) ;
#9712=CARTESIAN_POINT ( 'NONE',  ( 83.77821517812500929, -33.21562499938548285, 97.61286128772489690 ) ) ;
#9713=CARTESIAN_POINT ( 'NONE',  ( -96.99999999999998579, -5.200000000000000178, 150.0000000000000000 ) ) ;
#9717=CARTESIAN_POINT ( 'NONE',  ( 83.09162395290300651, -31.99999999999999289, 97.24830349208647817 ) ) ;
#9718=CARTESIAN_POINT ( 'NONE',  ( 85.15643035624999868, -31.97812499938548925, 101.5914258081833879 ) ) ;
#9719=CARTESIAN_POINT ( 'NONE',  ( 79.64356964375001269, -34.56562499938549138, -101.5914258081833879 ) ) ;
#9721=CARTESIAN_POINT ( 'NONE',  ( -79.64356964374999848, -34.97812499938548569, 99.99999999999998579 ) ) ;
#9722=CARTESIAN_POINT ( 'NONE',  ( -79.64356964375001269, -31.75312499938548427, -98.40857419181659793 ) ) ;
#9725=CARTESIAN_POINT ( 'NONE',  ( 79.64356964375001269, -33.59062499938548285, 101.5914258081833879 ) ) ;
#9726=DIRECTION ( 'NONE',  ( 1.586032892321652285E-15, 1.000000000000000000, 0.000000000000000000 ) ) ;
#9729=CARTESIAN_POINT ( 'NONE',  ( -83.77821517812500929, -34.82812499938548711, 97.61286128772489690 ) ) ;
#9732=CARTESIAN_POINT ( 'NONE',  ( -79.39999999999999147, -34.72500000000000142, -99.99999999999998579 ) ) ;
#9739=CARTESIAN_POINT ( 'NONE',  ( 85.40000000000000568, -33.99374999877097281, -99.99999999999998579 ) ) ;
#9740=CARTESIAN_POINT ( 'NONE',  ( 96.99999999999997158, -5.200000000000003730, 150.0000000000000000 ) ) ;
#9742=DIRECTION ( 'NONE',  ( -0.000000000000000000, -0.000000000000000000, -1.000000000000000000 ) ) ;
#9744=CARTESIAN_POINT ( 'NONE',  ( 82.65333140691207348, -34.99995246259152992, 102.9892844631211943 ) ) ;
#9745=CARTESIAN_POINT ( 'NONE',  ( 83.77821517812500929, -30.32812499938548711, -97.61286128772489690 ) ) ;
#9746=CARTESIAN_POINT ( 'NONE',  ( 82.39999999999999147, -34.83749999999999858, -103.0000000000000000 ) ) ;
#9747=EDGE_LOOP ( 'NONE', ( #1414, #2803, #231, #3203 ) ) ;
#9753=CARTESIAN_POINT ( 'NONE',  ( 83.20384757729335945, -34.14240381056767148, 102.9999999999999716 ) ) ;
#9755=ADVANCED_FACE ( 'NONE', ( #13672 ), #18272, .T. ) ;
#9756=CARTESIAN_POINT ( 'NONE',  ( -83.77821517812500929, -32.46562499938548285, -102.3871387122750889 ) ) ;
#9757=CARTESIAN_POINT ( 'NONE',  ( 94.79999999999995453, -29.80000000000000071, -150.0000000000000000 ) ) ;
#9759=CARTESIAN_POINT ( 'NONE',  ( 85.15643035625001289, -32.99062499938548854, 101.5914258081833879 ) ) ;
#9760=CARTESIAN_POINT ( 'NONE',  ( -79.39999999999999147, -33.80624999877097281, -98.26794919243113213 ) ) ;
#9762=CARTESIAN_POINT ( 'NONE',  ( 83.90000000000000568, -34.12500000000000000, 102.5980762113533018 ) ) ;
#9763=AXIS2_PLACEMENT_3D ( 'NONE', #7651, #9209, #16359 ) ;
#9767=CARTESIAN_POINT ( 'NONE',  ( -82.39999999999999147, -32.27812499938548285, -96.81714838363319586 ) ) ;
#9769=CARTESIAN_POINT ( 'NONE',  ( -81.59615242270662350, -34.31115380933863435, 102.9999999999999716 ) ) ;
#9773=CARTESIAN_POINT ( 'NONE',  ( 79.64356964374998427, -32.57812499938548711, -98.40857419181659793 ) ) ;
#9775=CARTESIAN_POINT ( 'NONE',  ( -82.40000000000001990, -32.30624999877097281, 97.00000000000000000 ) ) ;
#9782=CARTESIAN_POINT ( 'NONE',  ( -85.40000000000000568, -34.03124999877096712, -101.7320508075688821 ) ) ;
#9784=ORIENTED_EDGE ( 'NONE', *, *, #15435, .F. ) ;
#9785=CARTESIAN_POINT ( 'NONE',  ( -96.99999999999998579, -29.80000000000000426, 150.0000000000000000 ) ) ;
#9786=CARTESIAN_POINT ( 'NONE',  ( 79.39999999999999147, -32.43750000000000000, -98.26794919243110371 ) ) ;
#9787=DIRECTION ( 'NONE',  ( 0.000000000000000000, 0.000000000000000000, 1.000000000000000000 ) ) ;
#9788=CARTESIAN_POINT ( 'NONE',  ( -79.64356964375001269, -32.31562499938548427, 101.5914258081833879 ) ) ;
#9794=CARTESIAN_POINT ( 'NONE',  ( -82.40000000000001990, -33.88124999877096855, 103.0000000000000000 ) ) ;
#9795=CARTESIAN_POINT ( 'NONE',  ( -79.64356964374999848, -32.61562499938548854, 99.99999999999998579 ) ) ;
#9798=( LENGTH_UNIT ( ) NAMED_UNIT ( * ) SI_UNIT ( .MILLI., .METRE. ) );
#9800=DIRECTION ( 'NONE',  ( -0.000000000000000000, -1.000000000000000000, -0.000000000000000000 ) ) ;
#9805=CARTESIAN_POINT ( 'NONE',  ( -81.44948931429648553, -34.99999999999999289, -97.40655328406454316 ) ) ;
#9808=CARTESIAN_POINT ( 'NONE',  ( 81.02178482187500208, -32.24062499938548854, 97.61286128772489690 ) ) ;
#9813=CARTESIAN_POINT ( 'NONE',  ( -83.77821517812500929, -33.32812499938548711, -97.61286128772489690 ) ) ;
#9814=CARTESIAN_POINT ( 'NONE',  ( 79.64356964374999848, -31.26562499938548356, 99.99999999999998579 ) ) ;
#9815=CARTESIAN_POINT ( 'NONE',  ( 79.64356964375001269, -33.14062499938548711, -98.40857419181659793 ) ) ;
#9817=CARTESIAN_POINT ( 'NONE',  ( -85.15643035625001289, -32.42812499938548854, 98.40857419181659793 ) ) ;
#9818=CARTESIAN_POINT ( 'NONE',  ( 85.15643035624999868, -31.00312499938548072, -101.5914258081833879 ) ) ;
#9820=CARTESIAN_POINT ( 'NONE',  ( 82.39999999999999147, -34.64062499938548711, 96.81714838363319586 ) ) ;
#9823=CARTESIAN_POINT ( 'NONE',  ( -85.15643035625001289, -31.04062499938548569, 99.99999999999998579 ) ) ;
#9824=CARTESIAN_POINT ( 'NONE',  ( -83.77821517812500929, -30.21562499938548285, 97.61286128772489690 ) ) ;
#9827=CARTESIAN_POINT ( 'NONE',  ( -80.90000000000000568, -33.89999999999999858, -97.40192378864668399 ) ) ;
#9829=DIRECTION ( 'NONE',  ( 1.000000000000000000, 0.000000000000000000, 0.000000000000000000 ) ) ;
#9834=CARTESIAN_POINT ( 'NONE',  ( -83.41996205656103314, -35.00000000000000000, 97.17173842519740390 ) ) ;
#9837=CARTESIAN_POINT ( 'NONE',  ( 81.02178482187500208, -31.30312499938548498, 102.3871387122750889 ) ) ;
#9840=CARTESIAN_POINT ( 'NONE',  ( 81.02178482187500208, -33.10312499938548569, -97.61286128772489690 ) ) ;
#9841=CARTESIAN_POINT ( 'NONE',  ( 79.39999999999999147, -32.90624999877096712, 98.26794919243113213 ) ) ;
#9844=CARTESIAN_POINT ( 'NONE',  ( 80.90000000000000568, -30.99374999877096926, 102.5980762113533018 ) ) ;
#9846=EDGE_CURVE ( 'NONE', #2874, #7323, #3946, .T. ) ;
#9851=CARTESIAN_POINT ( 'NONE',  ( 82.39999999999999147, -34.83749999999999858, 97.00000000000000000 ) ) ;
#9853=CARTESIAN_POINT ( 'NONE',  ( -79.64356964375001269, -30.85312499938548569, -98.40857419181659793 ) ) ;
#9857=CARTESIAN_POINT ( 'NONE',  ( 82.39999999999999147, -33.96562499938548285, 103.1828516163667899 ) ) ;
#9858=CARTESIAN_POINT ( 'NONE',  ( -79.64356964374999848, -30.47812499938548569, -99.99999999999998579 ) ) ;
#9860=CARTESIAN_POINT ( 'NONE',  ( 79.39999999999999147, -34.23750000000000426, 101.7320508075688821 ) ) ;
#9869=CARTESIAN_POINT ( 'NONE',  ( 85.15643035625001289, -32.80312499938548854, -101.5914258081833879 ) ) ;
#9878=ORIENTED_EDGE ( 'NONE', *, *, #18087, .F. ) ;
#9881=ORIENTED_EDGE ( 'NONE', *, *, #516, .F. ) ;
#9883=CARTESIAN_POINT ( 'NONE',  ( 79.39999999999999147, -32.96250000000000568, -101.7320508075688537 ) ) ;
#9887=CARTESIAN_POINT ( 'NONE',  ( -82.39999999999999147, -31.26562499938549067, 96.81714838363319586 ) ) ;
#9890=DIRECTION ( 'NONE',  ( -1.586032892321652088E-15, -1.000000000000000000, 0.000000000000000000 ) ) ;
#9891=CARTESIAN_POINT ( 'NONE',  ( 83.77821517812500929, -34.67812499938548854, -102.3871387122750889 ) ) ;
#9894=CARTESIAN_POINT ( 'NONE',  ( 85.16220480609830190, -35.00000000000000000, 101.0868535717095682 ) ) ;
#9903=CIRCLE ( 'NONE', #1476, 2.199999999999993516 ) ;
#9905=CARTESIAN_POINT ( 'NONE',  ( 96.99999999999998579, 4.758098676964956264E-15, 150.0000000000000000 ) ) ;
#9907=CARTESIAN_POINT ( 'NONE',  ( -85.40000000000000568, -30.43124999877096926, 98.26794919243111792 ) ) ;
#9908=CARTESIAN_POINT ( 'NONE',  ( 79.39999999999999147, -30.67500000000000071, 99.99999999999998579 ) ) ;
#9913=CARTESIAN_POINT ( 'NONE',  ( -85.15643035625001289, -34.75312499938548427, -99.99999999999998579 ) ) ;
#9914=CARTESIAN_POINT ( 'NONE',  ( 81.02178482187500208, -32.69062499938548427, 97.61286128772489690 ) ) ;
#9916=CARTESIAN_POINT ( 'NONE',  ( 79.64356964375001269, -34.94062499938549138, -98.40857419181659793 ) ) ;
#9918=CARTESIAN_POINT ( 'NONE',  ( -81.02178482187500208, -32.24062499938548854, 102.3871387122750889 ) ) ;
#9919=CARTESIAN_POINT ( 'NONE',  ( 85.15643035624999868, -31.45312499938548356, -101.5914258081833879 ) ) ;
#9920=ORIENTED_EDGE ( 'NONE', *, *, #17017, .T. ) ;
#9925=CARTESIAN_POINT ( 'NONE',  ( -81.02178482187500208, -33.14062499938548711, 102.3871387122750889 ) ) ;
#9926=CARTESIAN_POINT ( 'NONE',  ( -82.39999999999999147, -30.70312499938548711, 96.81714838363319586 ) ) ;
#9929=AXIS2_PLACEMENT_3D ( 'NONE', #671, #15608, #2124 ) ;
#9935=CARTESIAN_POINT ( 'NONE',  ( -80.90000000000000568, -32.79374999877096997, 97.40192378864668399 ) ) ;
#9940=CARTESIAN_POINT ( 'NONE',  ( 83.77821517812500929, -33.02812499938548285, -97.61286128772489690 ) ) ;
#9942=CARTESIAN_POINT ( 'NONE',  ( 80.90000000000000568, -32.79374999877096997, 102.5980762113533018 ) ) ;
#9945=CARTESIAN_POINT ( 'NONE',  ( 79.39999999999999147, -32.83124999877097139, 101.7320508075688821 ) ) ;
#9950=ADVANCED_FACE ( 'NONE', ( #5661 ), #17667, .F. ) ;
#9953=ORIENTED_EDGE ( 'NONE', *, *, #17646, .T. ) ;
#9954=CARTESIAN_POINT ( 'NONE',  ( -83.77821517812500929, -31.11562499938548498, -102.3871387122750889 ) ) ;
#9955=CARTESIAN_POINT ( 'NONE',  ( 83.90000000000000568, -33.22500000000000142, 102.5980762113533018 ) ) ;
#9958=CARTESIAN_POINT ( 'NONE',  ( 82.39999999999999147, -34.19062499938548427, 96.81714838363319586 ) ) ;
#9959=CARTESIAN_POINT ( 'NONE',  ( -82.39999999999999147, -31.04062499938548569, -96.81714838363319586 ) ) ;
#9960=CARTESIAN_POINT ( 'NONE',  ( 85.40000000000000568, -34.01250000000000284, 98.26794919243111792 ) ) ;
#9961=LINE ( 'NONE', #15725, #15677 ) ;
#9964=CARTESIAN_POINT ( 'NONE',  ( -83.77821517812500929, -33.81562499938548427, -102.3871387122750889 ) ) ;
#9965=ADVANCED_FACE ( 'NONE', ( #1443 ), #2813, .T. ) ;
#9967=EDGE_CURVE ( 'NONE', #10928, #9562, #7310, .T. ) ;
#9968=CARTESIAN_POINT ( 'NONE',  ( 79.39999999999999147, -31.10624999877097352, -101.7320508075688537 ) ) ;
#9975=CARTESIAN_POINT ( 'NONE',  ( 83.20384757729337366, -32.79240381056766296, 103.0000000000000000 ) ) ;
#9978=ORIENTED_EDGE ( 'NONE', *, *, #9240, .T. ) ;
#9982=CARTESIAN_POINT ( 'NONE',  ( 82.39999999999999147, -32.81250000000000000, -96.53589838486223584 ) ) ;
#9983=FACE_OUTER_BOUND ( 'NONE', #18847, .T. ) ;
#9984=( BOUNDED_CURVE ( )  B_SPLINE_CURVE ( 2, ( #12774, #3879, #11502, #4076, #2506, #8375, #7008, #2313, #10133 ),
 .UNSPECIFIED., .F., .F. ) 
 B_SPLINE_CURVE_WITH_KNOTS ( ( 3, 2, 2, 2, 3 ),
 ( 0.4791666666666666297, 0.4861111111111111049, 0.5000000000000000000, 0.5138888888888888395, 0.5208333333333334814 ),
 .UNSPECIFIED. ) 
 CURVE ( )  GEOMETRIC_REPRESENTATION_ITEM ( )  RATIONAL_B_SPLINE_CURVE ( ( 0.9330127018922194093, 0.9330127018922190762, 1.000000000000000000, 0.8660254037844387076, 1.000000000000000000, 0.8660254037844387076, 1.000000000000000000, 0.9330127018922177440, 0.9330127018922194093 ) ) 
 REPRESENTATION_ITEM ( '' )  );
#9985=CARTESIAN_POINT ( 'NONE',  ( -85.15643035624999868, -32.46562499938548996, 101.5914258081833879 ) ) ;
#9989=CARTESIAN_POINT ( 'NONE',  ( 79.64356964374999848, -34.97812499938548569, -99.99999999999998579 ) ) ;
#9991=CARTESIAN_POINT ( 'NONE',  ( -79.64356964374999848, -34.41562499938548569, 99.99999999999998579 ) ) ;
#9992=DIRECTION ( 'NONE',  ( 0.000000000000000000, -1.000000000000000000, 0.000000000000000000 ) ) ;
#9993=ORIENTED_EDGE ( 'NONE', *, *, #14393, .F. ) ;
#9997=CARTESIAN_POINT ( 'NONE',  ( 82.40000000000000568, -34.78124999877096712, 96.99999999999998579 ) ) ;
#10000=ORIENTED_EDGE ( 'NONE', *, *, #6947, .F. ) ;
#10001=EDGE_CURVE ( 'NONE', #17378, #16799, #1478, .T. ) ;
#10003=DIRECTION ( 'NONE',  ( -0.000000000000000000, -1.000000000000000000, -0.000000000000000000 ) ) ;
#10004=CARTESIAN_POINT ( 'NONE',  ( 79.64356964375001269, -34.82812499938548711, 101.5914258081833879 ) ) ;
#10009=CARTESIAN_POINT ( 'NONE',  ( -85.15643035625001289, -33.81562499938548427, -98.40857419181659793 ) ) ;
#10010=CARTESIAN_POINT ( 'NONE',  ( 85.15643035625001289, -33.29062499938547859, 99.99999999999998579 ) ) ;
#10011=CARTESIAN_POINT ( 'NONE',  ( 81.02178482187500208, -34.60312499938549280, -102.3871387122750889 ) ) ;
#10013=CARTESIAN_POINT ( 'NONE',  ( -79.64356964374998427, -33.92812499938548854, 98.40857419181659793 ) ) ;
#10014=CARTESIAN_POINT ( 'NONE',  ( 83.77821517812500929, -31.41562499938548569, -102.3871387122750889 ) ) ;
#10016=CARTESIAN_POINT ( 'NONE',  ( 81.02178482187500208, -34.60312499938549280, 97.61286128772489690 ) ) ;
#10017=EDGE_CURVE ( 'NONE', #16451, #13073, #6695, .T. ) ;
#10020=CARTESIAN_POINT ( 'NONE',  ( -83.77821517812500929, -34.11562499938548854, 102.3871387122750889 ) ) ;
#10021=CARTESIAN_POINT ( 'NONE',  ( -82.39999999999999147, -30.47812499938548569, 103.1828516163667899 ) ) ;
#10023=CARTESIAN_POINT ( 'NONE',  ( 85.39999999999999147, -34.97364041986484295, 101.0919042218176287 ) ) ;
#10024=CARTESIAN_POINT ( 'NONE',  ( 79.77811200999867935, -34.99999999999999289, -100.8506536761476013 ) ) ;
#10025=CARTESIAN_POINT ( 'NONE',  ( 82.65333140691205926, -34.99995246259152282, -97.01071553687880566 ) ) ;
#10026=( BOUNDED_CURVE ( )  B_SPLINE_CURVE ( 2, ( #9997, #15762, #14469, #8330, #13108, #6969, #16048, #14286, #5610 ),
 .UNSPECIFIED., .F., .F. ) 
 B_SPLINE_CURVE_WITH_KNOTS ( ( 3, 2, 2, 2, 3 ),
 ( 0.8125000000000001110, 0.8194444444444444198, 0.8333333333333333703, 0.8472222222222222099, 0.8530683953269213582 ),
 .UNSPECIFIED. ) 
 CURVE ( )  GEOMETRIC_REPRESENTATION_ITEM ( )  RATIONAL_B_SPLINE_CURVE ( ( 0.9330127018922194093, 0.9330127018922204085, 1.000000000000000000, 0.8660254037844387076, 1.000000000000000000, 0.8660254037844387076, 1.000000000000000000, 0.9436068149601996025, 0.9346881722405915305 ) ) 
 REPRESENTATION_ITEM ( '' )  );
#10030=DIRECTION ( 'NONE',  ( -0.000000000000000000, -1.000000000000000000, -0.000000000000000000 ) ) ;
#10032=CARTESIAN_POINT ( 'NONE',  ( 79.64356964374999848, -30.47812499938548569, 99.99999999999998579 ) ) ;
#10034=DIRECTION ( 'NONE',  ( 1.000000000000000000, -1.586032892321652285E-15, 0.000000000000000000 ) ) ;
#10035=CARTESIAN_POINT ( 'NONE',  ( 79.64356964375001269, -34.49062499938548854, -98.40857419181659793 ) ) ;
#10039=CARTESIAN_POINT ( 'NONE',  ( 79.39999999999999147, -34.25624999877096855, 98.26794919243113213 ) ) ;
#10043=CARTESIAN_POINT ( 'NONE',  ( 82.40000000000000568, -34.61250000000001137, 102.9999999999999858 ) ) ;
#10046=CARTESIAN_POINT ( 'NONE',  ( -79.64356964375001269, -33.47812499938547859, -101.5914258081833879 ) ) ;
#10047=CARTESIAN_POINT ( 'NONE',  ( -82.40000000000000568, -30.00000000000000355, -99.99999999999998579 ) ) ;
#10048=ORIENTED_EDGE ( 'NONE', *, *, #11184, .F. ) ;
#10049=CARTESIAN_POINT ( 'NONE',  ( -82.40000000000000568, -34.78124999877096712, -96.99999999999998579 ) ) ;
#10050=CARTESIAN_POINT ( 'NONE',  ( -80.90000000000000568, -35.19374999877096855, -97.40192378864668399 ) ) ;
#10051=CARTESIAN_POINT ( 'NONE',  ( 85.40000000000000568, -33.63750000000000284, 101.7320508075688679 ) ) ;
#10055=CARTESIAN_POINT ( 'NONE',  ( -83.77821517812500929, -33.21562499938548285, -97.61286128772489690 ) ) ;
#10058=( BOUNDED_CURVE ( )  B_SPLINE_CURVE ( 2, ( #1046, #5353, #11296, #13136, #7187, #2589, #8550, #4165, #18923 ),
 .UNSPECIFIED., .F., .F. ) 
 B_SPLINE_CURVE_WITH_KNOTS ( ( 3, 2, 2, 2, 3 ),
 ( 0.6458333333333332593, 0.6527777777777777901, 0.6666666666666666297, 0.6805555555555555802, 0.6875000000000000000 ),
 .UNSPECIFIED. ) 
 CURVE ( )  GEOMETRIC_REPRESENTATION_ITEM ( )  RATIONAL_B_SPLINE_CURVE ( ( 0.9330127018922192983, 0.9330127018922187432, 1.000000000000000000, 0.8660254037844387076, 1.000000000000000000, 0.8660254037844387076, 1.000000000000000000, 0.9330127018922194093, 0.9330127018922194093 ) ) 
 REPRESENTATION_ITEM ( '' )  );
#10060=CARTESIAN_POINT ( 'NONE',  ( 82.39999999999999147, -31.18124999877096926, -103.4641016151377499 ) ) ;
#10069=ORIENTED_EDGE ( 'NONE', *, *, #11276, .T. ) ;
#10072=AXIS2_PLACEMENT_3D ( 'NONE', #3034, #9279, #11925 ) ;
#10074=EDGE_LOOP ( 'NONE', ( #13785, #13981, #5400, #16404 ) ) ;
#10076=CARTESIAN_POINT ( 'NONE',  ( 82.39999999999999147, -32.13749999999999574, -103.4641016151377499 ) ) ;
#10077=CARTESIAN_POINT ( 'NONE',  ( 79.93183330737450376, -31.99999999999999289, -101.6855250459189648 ) ) ;
#10078=CARTESIAN_POINT ( 'NONE',  ( -85.15643035624999868, -30.66562499938548569, 101.5914258081833879 ) ) ;
#10080=CARTESIAN_POINT ( 'NONE',  ( -79.39999999999999147, -34.76250000000000284, -98.26794919243113213 ) ) ;
#10081=EDGE_CURVE ( 'NONE', #1717, #9376, #16705, .T. ) ;
#10082=FACE_OUTER_BOUND ( 'NONE', #1695, .T. ) ;
#10084=CARTESIAN_POINT ( 'NONE',  ( 94.79999999999995453, -29.80000000000000071, 150.0000000000000000 ) ) ;
#10086=CARTESIAN_POINT ( 'NONE',  ( -83.90000000000000568, -34.36874999877097281, -97.40192378864668399 ) ) ;
#10088=CARTESIAN_POINT ( 'NONE',  ( -85.15643035624999868, -31.97812499938548925, -101.5914258081833879 ) ) ;
#10093=CARTESIAN_POINT ( 'NONE',  ( 79.39999999999999147, -32.51250000000000284, 98.26794919243113213 ) ) ;
#10095=( BOUNDED_CURVE ( )  B_SPLINE_CURVE ( 2, ( #5266, #17274, #9942, #5362, #19026, #9841, #8559, #866, #5554 ),
 .UNSPECIFIED., .F., .T. ) 
 B_SPLINE_CURVE_WITH_KNOTS ( ( 3, 2, 2, 2, 3 ),
 ( 0.4374999999999999445, 0.4444444444444444198, 0.4583333333333333148, 0.4722222222222222099, 0.4791666666666666297 ),
 .UNSPECIFIED. ) 
 CURVE ( )  GEOMETRIC_REPRESENTATION_ITEM ( )  RATIONAL_B_SPLINE_CURVE ( ( 0.9330127018922192983, 0.9330127018922187432, 1.000000000000000000, 0.8660254037844387076, 1.000000000000000000, 0.8660254037844387076, 1.000000000000000000, 0.9330127018922196314, 0.9330127018922194093 ) ) 
 REPRESENTATION_ITEM ( '' )  );
#10096=EDGE_CURVE ( 'NONE', #12925, #3019, #9339, .T. ) ;
#10100=CARTESIAN_POINT ( 'NONE',  ( -83.41996205656103314, -35.00000000000000000, -102.8282615748025108 ) ) ;
#10101=CARTESIAN_POINT ( 'NONE',  ( 85.15643035625001289, -34.19062499938548427, 99.99999999999998579 ) ) ;
#10106=CARTESIAN_POINT ( 'NONE',  ( -85.15643035625001289, -32.99062499938548854, -101.5914258081833879 ) ) ;
#10108=CARTESIAN_POINT ( 'NONE',  ( 85.15643035625001289, -35.20312499938548711, -99.99999999999998579 ) ) ;
#10111=CARTESIAN_POINT ( 'NONE',  ( -82.39999999999999147, -32.50312499938548427, 96.81714838363319586 ) ) ;
#10112=DIRECTION ( 'NONE',  ( -0.000000000000000000, -0.000000000000000000, -1.000000000000000000 ) ) ;
#10114=CARTESIAN_POINT ( 'NONE',  ( 84.51155386534844638, -35.25364837475780888, 101.7717924772919957 ) ) ;
#10115=FACE_BOUND ( 'NONE', #11951, .T. ) ;
#10117=CARTESIAN_POINT ( 'NONE',  ( -85.15643035624999868, -33.32812499938548001, 98.40857419181659793 ) ) ;
#10118=CARTESIAN_POINT ( 'NONE',  ( -82.39999999999999147, -31.15312499938548640, 96.81714838363319586 ) ) ;
#10122=CARTESIAN_POINT ( 'NONE',  ( 84.70388354820681798, -35.00002705695767702, 101.9214814096700934 ) ) ;
#10129=CARTESIAN_POINT ( 'NONE',  ( 82.39999999999999147, -33.51562499938548001, 103.1828516163667899 ) ) ;
#10132=CARTESIAN_POINT ( 'NONE',  ( 81.02178482187500208, -34.60312499938549280, -102.3871387122750889 ) ) ;
#10133=CARTESIAN_POINT ( 'NONE',  ( -82.39999999999999147, -33.20624999877097849, 97.00000000000000000 ) ) ;
#10135=CARTESIAN_POINT ( 'NONE',  ( 82.39999999999999147, -33.65624999877096712, 103.4641016151377499 ) ) ;
#10138=DIRECTION ( 'NONE',  ( 0.000000000000000000, 0.000000000000000000, -1.000000000000000000 ) ) ;
#10139=CARTESIAN_POINT ( 'NONE',  ( -84.85538848574856274, -35.00000000000001421, -101.7224313860082674 ) ) ;
#10141=CARTESIAN_POINT ( 'NONE',  ( -81.02178482187500208, -34.79062499938548569, -102.3871387122750889 ) ) ;
#10142=CARTESIAN_POINT ( 'NONE',  ( 79.39999999999999147, -32.38124999877096855, 101.7320508075688963 ) ) ;
#10144=CARTESIAN_POINT ( 'NONE',  ( -79.64356964375001269, -30.44062499938548783, -101.5914258081833879 ) ) ;
#10146=CARTESIAN_POINT ( 'NONE',  ( -80.90000000000000568, -31.89374999877096784, -102.5980762113533018 ) ) ;
#10150=CARTESIAN_POINT ( 'NONE',  ( -84.05108659120797654, -32.00820041275124339, -102.2295963284774842 ) ) ;
#10154=CARTESIAN_POINT ( 'NONE',  ( 79.39999999999999147, -31.51874999877096784, -99.99999999999998579 ) ) ;
#10157=CARTESIAN_POINT ( 'NONE',  ( 83.77821517812500929, -34.26562499938548711, -97.61286128772489690 ) ) ;
#10161=ORIENTED_EDGE ( 'NONE', *, *, #5795, .F. ) ;
#10163=CARTESIAN_POINT ( 'NONE',  ( -79.39999999999999147, -32.02500000000000568, 99.99999999999998579 ) ) ;
#10164=CIRCLE ( 'NONE', #17966, 3.000000000000002665 ) ;
#10169=CARTESIAN_POINT ( 'NONE',  ( 84.44763168836730927, -32.00000000000000711, -101.8452947671444093 ) ) ;
#10170=CARTESIAN_POINT ( 'NONE',  ( -85.15643035625001289, -32.50312499938548427, 99.99999999999998579 ) ) ;
#10175=CARTESIAN_POINT ( 'NONE',  ( 84.75088379146879447, -34.99999999999999289, 98.39201219457936531 ) ) ;
#10177=EDGE_LOOP ( 'NONE', ( #14397, #14420, #13230, #12759 ) ) ;
#10178=CARTESIAN_POINT ( 'NONE',  ( -83.77821517812500929, -30.51562499938548711, -97.61286128772489690 ) ) ;
#10179=CYLINDRICAL_SURFACE ( 'NONE', #1485, 3.000000000000002665 ) ;
#10186=EDGE_CURVE ( 'NONE', #8568, #12074, #2350, .T. ) ;
#10189=ORIENTED_EDGE ( 'NONE', *, *, #14158, .T. ) ;
#10192=CARTESIAN_POINT ( 'NONE',  ( 85.40000000000000568, -32.15624999877096712, -101.7320508075688821 ) ) ;
#10193=CARTESIAN_POINT ( 'NONE',  ( 79.64356964375001269, -34.45312499938548711, 98.40857419181659793 ) ) ;
#10194=CARTESIAN_POINT ( 'NONE',  ( 82.40000000000000568, -33.93750000000000711, -102.9999999999999858 ) ) ;
#10201=CARTESIAN_POINT ( 'NONE',  ( 83.77821517812500929, -31.41562499938548569, -102.3871387122750889 ) ) ;
#10204=CARTESIAN_POINT ( 'NONE',  ( -85.15643035625001289, -34.19062499938548427, 99.99999999999998579 ) ) ;
#10205=CARTESIAN_POINT ( 'NONE',  ( 81.02178482187500208, -31.64062499938548356, -97.61286128772489690 ) ) ;
#10208=ORIENTED_EDGE ( 'NONE', *, *, #4005, .F. ) ;
#10209=CARTESIAN_POINT ( 'NONE',  ( 79.64356964375001269, -34.04062499938549280, 101.5914258081833879 ) ) ;
#10210=CARTESIAN_POINT ( 'NONE',  ( -80.90000000000000568, -34.59374999877096712, 97.40192378864668399 ) ) ;
#10212=CARTESIAN_POINT ( 'NONE',  ( -81.02178482187500208, -34.49062499938548854, 102.3871387122750889 ) ) ;
#10213=ORIENTED_EDGE ( 'NONE', *, *, #10081, .F. ) ;
#10220=CARTESIAN_POINT ( 'NONE',  ( 83.20395887649171129, -35.00000000000000711, -102.6365808225363878 ) ) ;
#10223=CARTESIAN_POINT ( 'NONE',  ( 81.02178482187500208, -32.35312499938548569, 97.61286128772489690 ) ) ;
#10224=DIRECTION ( 'NONE',  ( 0.000000000000000000, 0.000000000000000000, -1.000000000000000000 ) ) ;
#10226=CARTESIAN_POINT ( 'NONE',  ( -82.39999999999999147, -33.48750000000000426, -97.00000000000000000 ) ) ;
#10227=CARTESIAN_POINT ( 'NONE',  ( 79.64356964374999848, -34.52812499938548285, -99.99999999999998579 ) ) ;
#10228=CARTESIAN_POINT ( 'NONE',  ( -81.02178482187500208, -31.30312499938548498, -102.3871387122750889 ) ) ;
#10229=ORIENTED_EDGE ( 'NONE', *, *, #15817, .T. ) ;
#10231=CARTESIAN_POINT ( 'NONE',  ( 79.39999999999999147, -34.18124999877097281, 101.7320508075688821 ) ) ;
#10234=EDGE_CURVE ( 'NONE', #18009, #5078, #14316, .T. ) ;
#10238=CARTESIAN_POINT ( 'NONE',  ( 83.30522522564156418, -32.00000000000000000, 102.6670244572690365 ) ) ;
#10240=CARTESIAN_POINT ( 'NONE',  ( -83.77821517812500929, -33.36562499938548854, -102.3871387122750889 ) ) ;
#10242=EDGE_LOOP ( 'NONE', ( #4913, #8280, #16363, #2927 ) ) ;
#10244=VECTOR ( 'NONE', #3089, 1000.000000000000000 ) ;
#10245=EDGE_CURVE ( 'NONE', #13073, #14240, #3365, .T. ) ;
#10246=CARTESIAN_POINT ( 'NONE',  ( -82.39999999999999147, -35.00624999877097565, -103.4641016151377499 ) ) ;
#10247=CARTESIAN_POINT ( 'NONE',  ( -83.30522522562117160, -32.00000000000001421, -102.6670244572773498 ) ) ;
#10248=CARTESIAN_POINT ( 'NONE',  ( -79.39999999999999147, -31.96874999877096712, -99.99999999999998579 ) ) ;
#10252=CARTESIAN_POINT ( 'NONE',  ( -85.15643035625001289, -34.15312499938548285, -98.40857419181659793 ) ) ;
#10254=VECTOR ( 'NONE', #5644, 1000.000000000000000 ) ;
#10255=CARTESIAN_POINT ( 'NONE',  ( -81.59615242270662350, -34.31115380933863435, -96.99999999999998579 ) ) ;
#10256=CARTESIAN_POINT ( 'NONE',  ( 85.40000000000000568, -31.25624999877096855, -101.7320508075688679 ) ) ;
#10259=DIRECTION ( 'NONE',  ( 1.586032892321652285E-15, 1.000000000000000000, 0.000000000000000000 ) ) ;
#10265=CARTESIAN_POINT ( 'NONE',  ( -84.28136653320154892, -32.00000000000001421, 97.98546077809197641 ) ) ;
#10272=CYLINDRICAL_SURFACE ( 'NONE', #8185, 3.000000000000002665 ) ;
#10274=CARTESIAN_POINT ( 'NONE',  ( -79.64356964375001269, -34.94062499938549138, 98.40857419181659793 ) ) ;
#10277=CARTESIAN_POINT ( 'NONE',  ( 82.41196654184807358, -35.00000000000000711, 102.9991646027828835 ) ) ;
#10278=CARTESIAN_POINT ( 'NONE',  ( 84.59935209580183368, -34.99999999999999289, 98.20719995774791755 ) ) ;
#10282=CARTESIAN_POINT ( 'NONE',  ( -81.02178482187500208, -35.05312499938548854, -97.61286128772489690 ) ) ;
#10289=ORIENTED_EDGE ( 'NONE', *, *, #8745, .F. ) ;
#10291=FACE_OUTER_BOUND ( 'NONE', #15973, .T. ) ;
#10294=CARTESIAN_POINT ( 'NONE',  ( 82.39999999999999147, -34.75312499938549138, 103.1828516163667899 ) ) ;
#10295=CARTESIAN_POINT ( 'NONE',  ( -82.40000000000000568, -30.00000000000000355, 99.99999999999998579 ) ) ;
#10299=CARTESIAN_POINT ( 'NONE',  ( 79.64356964375001269, -33.55312499938548854, 98.40857419181659793 ) ) ;
#10301=CARTESIAN_POINT ( 'NONE',  ( 79.64356964375001269, -31.22812499938548925, -98.40857419181659793 ) ) ;
#10304=CARTESIAN_POINT ( 'NONE',  ( -83.77821517812500929, -34.71562499938548285, 97.61286128772489690 ) ) ;
#10305=CARTESIAN_POINT ( 'NONE',  ( 79.64356964375001269, -33.47812499938547859, -98.40857419181659793 ) ) ;
#10309=CARTESIAN_POINT ( 'NONE',  ( -83.77821517812500929, -32.31562499938548427, 102.3871387122750889 ) ) ;
#10311=CARTESIAN_POINT ( 'NONE',  ( -79.39999999999999147, -32.96250000000000568, 101.7320508075688537 ) ) ;
#10312=EDGE_CURVE ( 'NONE', #17007, #5783, #16965, .T. ) ;
#10320=CARTESIAN_POINT ( 'NONE',  ( 81.02178482187500208, -31.75312499938548427, 102.3871387122750889 ) ) ;
#10322=CARTESIAN_POINT ( 'NONE',  ( -83.90000000000000568, -32.77499999999999858, 97.40192378864668399 ) ) ;
#10324=CARTESIAN_POINT ( 'NONE',  ( -85.15643035625001289, -32.46562499938548996, 101.5914258081833879 ) ) ;
#10325=CARTESIAN_POINT ( 'NONE',  ( -85.15643035624999868, -31.56562499938548427, -98.40857419181659793 ) ) ;
#10326=VERTEX_POINT ( 'NONE', #19310 ) ;
#10327=CARTESIAN_POINT ( 'NONE',  ( 80.90000000000000568, -34.14374999877097139, 102.5980762113533018 ) ) ;
#10329=CARTESIAN_POINT ( 'NONE',  ( -83.77821517812500929, -32.87812499938548427, 102.3871387122750889 ) ) ;
#10331=ORIENTED_EDGE ( 'NONE', *, *, #12234, .F. ) ;
#10332=CARTESIAN_POINT ( 'NONE',  ( -82.39999999999999147, -33.85312499938547859, -103.1828516163667899 ) ) ;
#10333=LINE ( 'NONE', #2905, #8795 ) ;
#10336=CARTESIAN_POINT ( 'NONE',  ( -79.64356964375001269, -33.59062499938548285, -101.5914258081833879 ) ) ;
#10337=CARTESIAN_POINT ( 'NONE',  ( -82.39999999999999147, -32.53124999877096712, -96.53589838486223584 ) ) ;
#10341=CARTESIAN_POINT ( 'NONE',  ( -81.02178482187500208, -34.79062499938548569, -102.3871387122750889 ) ) ;
#10343=CARTESIAN_POINT ( 'NONE',  ( 96.99999999999994316, -21.80000000000003268, -139.9999999999999716 ) ) ;
#10344=CARTESIAN_POINT ( 'NONE',  ( 79.39999999999999147, -32.00624999877096855, -101.7320508075688537 ) ) ;
#10346=VERTEX_POINT ( 'NONE', #5543 ) ;
#10348=EDGE_CURVE ( 'NONE', #13073, #6638, #825, .T. ) ;
#10352=EDGE_LOOP ( 'NONE', ( #10498, #18080, #15259, #9616 ) ) ;
#10354=CARTESIAN_POINT ( 'NONE',  ( 80.90000000000000568, -34.20000000000000284, -97.40192378864668399 ) ) ;
#10362=CARTESIAN_POINT ( 'NONE',  ( -85.15643035625001289, -32.95312499938548711, 99.99999999999998579 ) ) ;
#10366=CARTESIAN_POINT ( 'NONE',  ( -82.40000000000000568, -30.00000000000000355, 99.99999999999998579 ) ) ;
#10367=CARTESIAN_POINT ( 'NONE',  ( -79.69416654173919312, -35.00000000000002132, -99.37250936986646366 ) ) ;
#10370=( NAMED_UNIT ( * ) SI_UNIT ( $, .STERADIAN. ) SOLID_ANGLE_UNIT ( ) );
#10371=CARTESIAN_POINT ( 'NONE',  ( -85.15643035624999868, -32.80312499938548854, -98.40857419181659793 ) ) ;
#10380=ORIENTED_EDGE ( 'NONE', *, *, #11281, .T. ) ;
#10382=CARTESIAN_POINT ( 'NONE',  ( -84.67508262029694777, -32.00000000000000711, 101.5663513044662665 ) ) ;
#10384=CARTESIAN_POINT ( 'NONE',  ( -79.39999999999999147, -31.96874999877096712, 99.99999999999998579 ) ) ;
#10385=CARTESIAN_POINT ( 'NONE',  ( 85.40000000000000568, -33.14999999999999858, 99.99999999999998579 ) ) ;
#10386=CARTESIAN_POINT ( 'NONE',  ( -94.79999999999999716, 0.000000000000000000, 150.0000000000000000 ) ) ;
#10390=CARTESIAN_POINT ( 'NONE',  ( 79.64356964374999848, -33.96562499938548285, 99.99999999999998579 ) ) ;
#10391=CARTESIAN_POINT ( 'NONE',  ( 85.15643035624999868, -31.45312499938548356, -101.5914258081833879 ) ) ;
#10392=ORIENTED_EDGE ( 'NONE', *, *, #18134, .T. ) ;
#10394=CARTESIAN_POINT ( 'NONE',  ( 79.39999999999999147, -34.21874999877096712, 99.99999999999998579 ) ) ;
#10395=CARTESIAN_POINT ( 'NONE',  ( 83.77821517812500929, -34.11562499938548854, -102.3871387122750889 ) ) ;
#10397=DIRECTION ( 'NONE',  ( 2.312964634635740689E-14, 0.000000000000000000, -1.000000000000000000 ) ) ;
#10398=CARTESIAN_POINT ( 'NONE',  ( -82.40000000000000568, -34.55624999877097281, 97.00000000000000000 ) ) ;
#10400=CARTESIAN_POINT ( 'NONE',  ( -85.15643035624999868, -35.11426541925033007, 98.99674735228809652 ) ) ;
#10401=VERTEX_POINT ( 'NONE', #4352 ) ;
#10402=CARTESIAN_POINT ( 'NONE',  ( -85.40000000000000568, -33.95624999877097139, 101.7320508075688821 ) ) ;
#10406=DIRECTION ( 'NONE',  ( -0.000000000000000000, 1.000000000000000000, 0.000000000000000000 ) ) ;
#10407=CARTESIAN_POINT ( 'NONE',  ( -79.68596062386968981, -32.00000000000002132, 101.2782762865727619 ) ) ;
#10409=CARTESIAN_POINT ( 'NONE',  ( -81.59615242270662350, -32.38259618943233420, 96.99999999999998579 ) ) ;
#10410=CARTESIAN_POINT ( 'NONE',  ( 83.77821517812500929, -32.42812499938548854, 97.61286128772489690 ) ) ;
#10414=CARTESIAN_POINT ( 'NONE',  ( -79.64356964375001269, -32.24062499938548854, -101.5914258081833879 ) ) ;
#10415=ORIENTED_EDGE ( 'NONE', *, *, #3294, .F. ) ;
#10416=CARTESIAN_POINT ( 'NONE',  ( 85.15643035624999868, -31.19062499938548783, 101.5914258081833879 ) ) ;
#10418=DIRECTION ( 'NONE',  ( 1.000000000000000000, 0.000000000000000000, -0.000000000000000000 ) ) ;
#10420=CARTESIAN_POINT ( 'NONE',  ( -79.64356964374999848, -31.37812499938548427, 99.99999999999998579 ) ) ;
#10423=CARTESIAN_POINT ( 'NONE',  ( -85.40000000000000568, -31.35000000000000142, -99.99999999999998579 ) ) ;
#10426=CARTESIAN_POINT ( 'NONE',  ( -82.39999999999999147, -33.51562499938548001, -103.1828516163667899 ) ) ;
#10428=CARTESIAN_POINT ( 'NONE',  ( -79.39999999999999147, -32.00624999877096855, -98.26794919243113213 ) ) ;
#10432=FACE_OUTER_BOUND ( 'NONE', #14313, .T. ) ;
#10433=CARTESIAN_POINT ( 'NONE',  ( 85.15643035625001289, -32.87812499938548427, 101.5914258081833879 ) ) ;
#10434=DIRECTION ( 'NONE',  ( 1.000000000000000000, 0.000000000000000000, -0.000000000000000000 ) ) ;
#10435=DIRECTION ( 'NONE',  ( 1.000000000000000000, -0.000000000000000000, -2.407412430484046130E-31 ) ) ;
#10436=CARTESIAN_POINT ( 'NONE',  ( 85.40000000000000568, -34.40624999877096712, -101.7320508075688679 ) ) ;
#10439=ORIENTED_EDGE ( 'NONE', *, *, #18544, .F. ) ;
#10447=VERTEX_POINT ( 'NONE', #16181 ) ;
#10452=CARTESIAN_POINT ( 'NONE',  ( 81.59615242270663771, -32.51115380933863008, -103.0000000000000000 ) ) ;
#10453=DIRECTION ( 'NONE',  ( -0.000000000000000000, -0.000000000000000000, -1.000000000000000000 ) ) ;
#10455=CARTESIAN_POINT ( 'NONE',  ( -83.77821517812500929, -33.47812499938548569, 97.61286128772489690 ) ) ;
#10457=EDGE_CURVE ( 'NONE', #5172, #6865, #2791, .T. ) ;
#10464=CARTESIAN_POINT ( 'NONE',  ( -85.15643035625001289, -32.84062499938548285, -99.99999999999998579 ) ) ;
#10468=CARTESIAN_POINT ( 'NONE',  ( 80.80861089413672005, -34.99999999999999289, -102.2789443502789055 ) ) ;
#10470=CARTESIAN_POINT ( 'NONE',  ( 82.39999999999999147, -32.36250000000000426, 102.9999999999999858 ) ) ;
#10473=ORIENTED_EDGE ( 'NONE', *, *, #2775, .F. ) ;
#10474=VERTEX_POINT ( 'NONE', #17835 ) ;
#10478=CARTESIAN_POINT ( 'NONE',  ( -79.39999999999999147, -32.86874999877097281, 99.99999999999998579 ) ) ;
#10479=CARTESIAN_POINT ( 'NONE',  ( 79.39999999999999147, -32.02500000000000568, 99.99999999999998579 ) ) ;
#10485=CARTESIAN_POINT ( 'NONE',  ( 82.61711639270117757, -31.99999999999999289, -97.16008101252806739 ) ) ;
#10486=( BOUNDED_CURVE ( )  B_SPLINE_CURVE ( 2, ( #12820, #17027, #14086, #15465, #2177, #15856, #3824, #17318, #2076 ),
 .UNSPECIFIED., .F., .F. ) 
 B_SPLINE_CURVE_WITH_KNOTS ( ( 3, 2, 2, 2, 3 ),
 ( 0.6875000000000000000, 0.6944444444444444198, 0.7083333333333333703, 0.7222222222222222099, 0.7291666666666668517 ),
 .UNSPECIFIED. ) 
 CURVE ( )  GEOMETRIC_REPRESENTATION_ITEM ( )  RATIONAL_B_SPLINE_CURVE ( ( 0.9330127018922194093, 0.9330127018922194093, 1.000000000000000000, 0.8660254037844387076, 1.000000000000000000, 0.8660254037844387076, 1.000000000000000000, 0.9330127018922177440, 0.9330127018922194093 ) ) 
 REPRESENTATION_ITEM ( '' )  );
#10487=CARTESIAN_POINT ( 'NONE',  ( 82.39999999999999147, -30.70312499938548711, -96.81714838363319586 ) ) ;
#10490=CARTESIAN_POINT ( 'NONE',  ( 80.90000000000000568, -34.14374999877097139, 102.5980762113533018 ) ) ;
#10491=CARTESIAN_POINT ( 'NONE',  ( 82.39999999999999147, -33.85312499938547859, -96.81714838363319586 ) ) ;
#10497=CARTESIAN_POINT ( 'NONE',  ( -82.39999999999999147, -30.33750000000000213, 103.4641016151377499 ) ) ;
#10498=ORIENTED_EDGE ( 'NONE', *, *, #2437, .F. ) ;
#10499=CARTESIAN_POINT ( 'NONE',  ( -80.90000000000000568, -34.35000000000000853, 102.5980762113533018 ) ) ;
#10500=CARTESIAN_POINT ( 'NONE',  ( 82.39999999999999147, -30.25312499938548783, 103.1828516163667899 ) ) ;
#10503=LINE ( 'NONE', #1528, #6432 ) ;
#10507=CARTESIAN_POINT ( 'NONE',  ( 82.39999999999999147, -32.61562499938548854, 103.1828516163667899 ) ) ;
#10508=CARTESIAN_POINT ( 'NONE',  ( 83.77821517812500929, -30.32812499938548711, -97.61286128772489690 ) ) ;
#10510=CARTESIAN_POINT ( 'NONE',  ( -85.14613134194615895, -31.99999999999997868, -100.2978599400816364 ) ) ;
#10511=CARTESIAN_POINT ( 'NONE',  ( -83.77821517812500929, -32.12812499938548427, -102.3871387122750889 ) ) ;
#10513=CARTESIAN_POINT ( 'NONE',  ( 79.39999999999999147, -35.08124999877097139, 101.7320508075688821 ) ) ;
#10515=CARTESIAN_POINT ( 'NONE',  ( 83.20384757729338787, -34.53615380933862866, 102.9999999999999858 ) ) ;
#10518=CARTESIAN_POINT ( 'NONE',  ( -85.15643035624999868, -31.56562499938548427, 101.5914258081833879 ) ) ;
#10519=CARTESIAN_POINT ( 'NONE',  ( 82.39999999999999147, -33.65624999877097423, -97.00000000000000000 ) ) ;
#10520=VERTEX_POINT ( 'NONE', #10122 ) ;
#10521=CARTESIAN_POINT ( 'NONE',  ( -80.90000000000000568, -31.05000000000000071, -102.5980762113533018 ) ) ;
#10522=AXIS2_PLACEMENT_3D ( 'NONE', #14184, #9992, #15567 ) ;
#10525=CARTESIAN_POINT ( 'NONE',  ( -79.64356964374999848, -33.62812499938548427, -99.99999999999998579 ) ) ;
#10531=CARTESIAN_POINT ( 'NONE',  ( -79.64356964374998427, -34.90312499938548285, -98.40857419181659793 ) ) ;
#10532=CARTESIAN_POINT ( 'NONE',  ( 79.64356964374999848, -32.61562499938548854, 99.99999999999998579 ) ) ;
#10533=CARTESIAN_POINT ( 'NONE',  ( 81.59615242270662350, -32.56740381056766864, -103.0000000000000000 ) ) ;
#10534=( BOUNDED_CURVE ( )  B_SPLINE_CURVE ( 2, ( #4714, #4325, #15059, #7633, #3231, #6084, #6280, #7346, #5891 ),
 .UNSPECIFIED., .F., .F. ) 
 B_SPLINE_CURVE_WITH_KNOTS ( ( 3, 2, 2, 2, 3 ),
 ( 0.3958333333333334259, 0.4027777777777777901, 0.4166666666666666852, 0.4305555555555555802, 0.4374999999999999445 ),
 .UNSPECIFIED. ) 
 CURVE ( )  GEOMETRIC_REPRESENTATION_ITEM ( )  RATIONAL_B_SPLINE_CURVE ( ( 0.9330127018922192983, 0.9330127018922200755, 1.000000000000000000, 0.8660254037844387076, 1.000000000000000000, 0.8660254037844387076, 1.000000000000000000, 0.9330127018922198534, 0.9330127018922192983 ) ) 
 REPRESENTATION_ITEM ( '' )  );
#10535=DIRECTION ( 'NONE',  ( 0.000000000000000000, 0.000000000000000000, -1.000000000000000000 ) ) ;
#10536=CARTESIAN_POINT ( 'NONE',  ( 79.39999999999999147, -35.08124999877097139, -98.26794919243110371 ) ) ;
#10540=AXIS2_PLACEMENT_3D ( 'NONE', #7341, #19270, #11738 ) ;
#10551=PLANE ( 'NONE',  #4128 ) ;
#10552=CARTESIAN_POINT ( 'NONE',  ( -83.20384757729335945, -33.69240381056766154, -102.9999999999999858 ) ) ;
#10553=ORIENTED_EDGE ( 'NONE', *, *, #315, .F. ) ;
#10556=AXIS2_PLACEMENT_3D ( 'NONE', #7528, #4505, #6173 ) ;
#10558=CARTESIAN_POINT ( 'NONE',  ( -82.39999999999999147, -33.06562499938548427, 96.81714838363319586 ) ) ;
#10564=EDGE_CURVE ( 'NONE', #12925, #2988, #194, .T. ) ;
#10567=CARTESIAN_POINT ( 'NONE',  ( -85.15643035624999868, -33.25312499938548427, -98.40857419181659793 ) ) ;
#10571=DIRECTION ( 'NONE',  ( 0.000000000000000000, 1.000000000000000000, 0.000000000000000000 ) ) ;
#10573=DIRECTION ( 'NONE',  ( 0.000000000000000000, -1.000000000000000000, 0.000000000000000000 ) ) ;
#10575=ORIENTED_EDGE ( 'NONE', *, *, #10788, .F. ) ;
#10579=CARTESIAN_POINT ( 'NONE',  ( -85.40000000000000568, -31.33124999877096428, 98.26794919243111792 ) ) ;
#10581=CARTESIAN_POINT ( 'NONE',  ( 80.90000000000000568, -32.55000000000000426, 97.40192378864668399 ) ) ;
#10582=CARTESIAN_POINT ( 'NONE',  ( -80.24533121543035463, -32.00000000000000711, -97.95829548583749613 ) ) ;
#10586=CARTESIAN_POINT ( 'NONE',  ( 81.02178482187500208, -32.24062499938548854, -102.3871387122750889 ) ) ;
#10589=CARTESIAN_POINT ( 'NONE',  ( 83.20384757729335945, -34.85759618943233562, -102.9999999999999716 ) ) ;
#10590=CARTESIAN_POINT ( 'NONE',  ( 81.02178482187500208, -33.44062499938548427, -97.61286128772489690 ) ) ;
#10591=DIRECTION ( 'NONE',  ( 0.000000000000000000, 0.000000000000000000, -1.000000000000000000 ) ) ;
#10593=EDGE_CURVE ( 'NONE', #15647, #18009, #13432, .T. ) ;
#10595=CARTESIAN_POINT ( 'NONE',  ( -85.15643035624999868, -34.67812499938548143, 98.40857419181659793 ) ) ;
#10596=ORIENTED_EDGE ( 'NONE', *, *, #9611, .F. ) ;
#10599=CARTESIAN_POINT ( 'NONE',  ( 83.77821517812500929, -30.96562499938548640, 97.61286128772489690 ) ) ;
#10603=CARTESIAN_POINT ( 'NONE',  ( -83.20384757729335945, -33.24240381056766580, -102.9999999999999716 ) ) ;
#10604=CARTESIAN_POINT ( 'NONE',  ( -80.90000000000000568, -32.40000000000000568, 97.40192378864668399 ) ) ;
#10605=CARTESIAN_POINT ( 'NONE',  ( 85.15643035624999868, -30.62812499938548427, 101.5914258081833879 ) ) ;
#10606=CARTESIAN_POINT ( 'NONE',  ( 80.08630547029510183, -32.02340763552835057, 97.87171054440995022 ) ) ;
#10607=CARTESIAN_POINT ( 'NONE',  ( -79.39999999999999147, -32.47500000000000142, -99.99999999999998579 ) ) ;
#10608=CARTESIAN_POINT ( 'NONE',  ( -94.79999999999999716, -35.00000000000000000, -150.0000000000000000 ) ) ;
#10609=CARTESIAN_POINT ( 'NONE',  ( -82.39999999999999147, -30.59062499938548640, -96.81714838363319586 ) ) ;
#10610=EDGE_LOOP ( 'NONE', ( #12833, #17979, #2734, #1912, #7797, #10189, #18983, #5373, #6619, #7063, #17105, #6921, #17184, #7220, #14358, #9920, #4205 ) ) ;
#10611=CARTESIAN_POINT ( 'NONE',  ( 81.02178482187500208, -30.40312499938548640, 102.3871387122750889 ) ) ;
#10614=CARTESIAN_POINT ( 'NONE',  ( -79.64356964374999848, -32.27812499938548996, 99.99999999999998579 ) ) ;
#10615=CARTESIAN_POINT ( 'NONE',  ( 85.40000000000000568, -33.09374999877096712, 99.99999999999998579 ) ) ;
#10617=CARTESIAN_POINT ( 'NONE',  ( -80.90000000000000568, -31.94999999999999929, -102.5980762113533018 ) ) ;
#10618=CARTESIAN_POINT ( 'NONE',  ( 82.85024983566745505, -34.99999999999999289, 102.9730910282409440 ) ) ;
#10619=CARTESIAN_POINT ( 'NONE',  ( 83.90000000000000568, -34.96874999877096712, -97.40192378864668399 ) ) ;
#10620=CARTESIAN_POINT ( 'NONE',  ( -85.15643035625001289, -33.40312499938548285, -99.99999999999998579 ) ) ;
#10621=CARTESIAN_POINT ( 'NONE',  ( 94.79999999999995453, -5.200000000000000178, -150.0000000000000000 ) ) ;
#10626=CARTESIAN_POINT ( 'NONE',  ( -79.64356964374999848, -33.96562499938548285, -99.99999999999998579 ) ) ;
#10627=CARTESIAN_POINT ( 'NONE',  ( 81.02178482187500208, -33.89062499938548711, 102.3871387122750889 ) ) ;
#10629=CARTESIAN_POINT ( 'NONE',  ( 85.40000000000000568, -32.66250000000000142, -101.7320508075688821 ) ) ;
#10630=CARTESIAN_POINT ( 'NONE',  ( 80.90000000000000568, -35.04374999877096997, -97.40192378864668399 ) ) ;
#10639=EDGE_LOOP ( 'NONE', ( #12272, #15721, #8102, #2995 ) ) ;
#10641=CARTESIAN_POINT ( 'NONE',  ( -79.39999999999999147, -34.68750000000000000, 98.26794919243110371 ) ) ;
#10642=ORIENTED_EDGE ( 'NONE', *, *, #16927, .F. ) ;
#10645=CARTESIAN_POINT ( 'NONE',  ( -83.77821517812500929, -34.67812499938548854, 102.3871387122750889 ) ) ;
#10653=CARTESIAN_POINT ( 'NONE',  ( -81.05805657947830412, -35.00000000000000711, -102.6149389257478362 ) ) ;
#10655=VERTEX_POINT ( 'NONE', #1618 ) ;
#10656=CARTESIAN_POINT ( 'NONE',  ( -85.15643035625001289, -32.39062499938548711, -99.99999999999998579 ) ) ;
#10658=DIRECTION ( 'NONE',  ( 0.000000000000000000, 0.000000000000000000, 1.000000000000000000 ) ) ;
#10659=CARTESIAN_POINT ( 'NONE',  ( -85.39999999999999147, -34.97364041986484295, -101.0919042218176287 ) ) ;
#10667=CARTESIAN_POINT ( 'NONE',  ( -83.90000000000000568, -31.81874999877096855, 97.40192378864668399 ) ) ;
#10668=CARTESIAN_POINT ( 'NONE',  ( 85.40000000000000568, -32.66250000000000142, 98.26794919243111792 ) ) ;
#10669=CARTESIAN_POINT ( 'NONE',  ( 83.90000000000000568, -33.61874999877097281, 102.5980762113533018 ) ) ;
#10671=CARTESIAN_POINT ( 'NONE',  ( 81.02178482187500208, -32.80312499938548854, -102.3871387122750889 ) ) ;
#10672=CARTESIAN_POINT ( 'NONE',  ( 81.59615242270665192, -33.28259618943233278, -97.00000000000000000 ) ) ;
#10674=( BOUNDED_CURVE ( )  B_SPLINE_CURVE ( 2, ( #6189, #18295, #3534, #337, #3627, #15159, #1972, #7738, #4720 ),
 .UNSPECIFIED., .F., .F. ) 
 B_SPLINE_CURVE_WITH_KNOTS ( ( 3, 2, 2, 2, 3 ),
 ( 0.7708333333333331483, 0.7777777777777777901, 0.7916666666666666297, 0.8055555555555555802, 0.8125000000000001110 ),
 .UNSPECIFIED. ) 
 CURVE ( )  GEOMETRIC_REPRESENTATION_ITEM ( )  RATIONAL_B_SPLINE_CURVE ( ( 0.9330127018922194093, 0.9330127018922177440, 1.000000000000000000, 0.8660254037844387076, 1.000000000000000000, 0.8660254037844387076, 1.000000000000000000, 0.9330127018922182991, 0.9330127018922194093 ) ) 
 REPRESENTATION_ITEM ( '' )  );
#10675=CARTESIAN_POINT ( 'NONE',  ( 85.15643035625001289, -34.19062499938548427, -99.99999999999998579 ) ) ;
#10679=CARTESIAN_POINT ( 'NONE',  ( -83.90000000000000568, -33.97500000000000853, 102.5980762113533018 ) ) ;
#10680=CARTESIAN_POINT ( 'NONE',  ( 85.15643035624999868, -32.42812499938548854, -98.40857419181659793 ) ) ;
#10681=ADVANCED_FACE ( 'NONE', ( #4938 ), #8683, .F. ) ;
#10682=DIRECTION ( 'NONE',  ( 0.000000000000000000, 0.000000000000000000, 1.000000000000000000 ) ) ;
#10685=ADVANCED_FACE ( 'NONE', ( #5176 ), #8575, .F. ) ;
#10686=CARTESIAN_POINT ( 'NONE',  ( -84.51155491706698797, -35.14114833091483803, 98.22820877610629964 ) ) ;
#10693=CARTESIAN_POINT ( 'NONE',  ( -83.20384757729335945, -33.05759618943233136, -96.99999999999998579 ) ) ;
#10694=ADVANCED_FACE ( 'NONE', ( #12688 ), #603, .F. ) ;
#10696=CARTESIAN_POINT ( 'NONE',  ( -80.90000000000000568, -32.55000000000000426, 102.5980762113533018 ) ) ;
#10697=CARTESIAN_POINT ( 'NONE',  ( 79.64356964375001269, -34.56562499938549138, 98.40857419181659793 ) ) ;
#10698=CARTESIAN_POINT ( 'NONE',  ( 83.77821517812500929, -32.87812499938548427, -102.3871387122750889 ) ) ;
#10700=CARTESIAN_POINT ( 'NONE',  ( -82.39999999999999147, -32.61562499938548854, 96.81714838363319586 ) ) ;
#10701=CARTESIAN_POINT ( 'NONE',  ( -82.39999999999999147, -32.61562499938548854, -103.1828516163667899 ) ) ;
#10704=CARTESIAN_POINT ( 'NONE',  ( 82.39999999999999147, -34.55624999877096570, 103.4641016151377499 ) ) ;
#10707=CARTESIAN_POINT ( 'NONE',  ( -79.64356964375001269, -31.79062499938548569, 98.40857419181659793 ) ) ;
#10708=CARTESIAN_POINT ( 'NONE',  ( 82.40000000000001990, -34.61250000000001137, -97.00000000000000000 ) ) ;
#10709=EDGE_LOOP ( 'NONE', ( #15102, #6629, #3235, #10392, #3311, #10760, #19268, #18007, #18117, #9709, #4269, #13420, #7514, #10733, #10229, #4180, #6054 ) ) ;
#10710=ADVANCED_FACE ( 'NONE', ( #13830 ), #4864, .F. ) ;
#10711=CARTESIAN_POINT ( 'NONE',  ( -83.90000000000000568, -30.97500000000000142, -102.5980762113533018 ) ) ;
#10712=( BOUNDED_CURVE ( )  B_SPLINE_CURVE ( 2, ( #13596, #14874, #12143, #18112, #8913, #4726, #10669, #6289, #16638 ),
 .UNSPECIFIED., .F., .F. ) 
 B_SPLINE_CURVE_WITH_KNOTS ( ( 3, 2, 2, 2, 3 ),
 ( 0.5625000000000000000, 0.5694444444444444198, 0.5833333333333333703, 0.5972222222222222099, 0.6041666666666666297 ),
 .UNSPECIFIED. ) 
 CURVE ( )  GEOMETRIC_REPRESENTATION_ITEM ( )  RATIONAL_B_SPLINE_CURVE ( ( 0.9330127018922194093, 0.9330127018922194093, 1.000000000000000000, 0.8660254037844387076, 1.000000000000000000, 0.8660254037844387076, 1.000000000000000000, 0.9330127018922198534, 0.9330127018922192983 ) ) 
 REPRESENTATION_ITEM ( '' )  );
#10713=CARTESIAN_POINT ( 'NONE',  ( 83.95700771753406855, -35.00000000000000000, 102.5724980549417324 ) ) ;
#10715=CARTESIAN_POINT ( 'NONE',  ( 82.40000000000001990, -34.16250000000000853, 103.0000000000000000 ) ) ;
#10719=EDGE_LOOP ( 'NONE', ( #17002, #1568, #7487, #16829 ) ) ;
#10721=CARTESIAN_POINT ( 'NONE',  ( 81.59615242270665192, -32.77634618820330559, -97.00000000000000000 ) ) ;
#10722=CARTESIAN_POINT ( 'NONE',  ( 79.64356964374999848, -34.41562499938548569, 99.99999999999998579 ) ) ;
#10725=CARTESIAN_POINT ( 'NONE',  ( 85.40000000000000568, -33.95624999877097139, -101.7320508075688679 ) ) ;
#10726=CARTESIAN_POINT ( 'NONE',  ( 82.39999999999999147, -34.83749999999999858, 97.00000000000000000 ) ) ;
#10733=ORIENTED_EDGE ( 'NONE', *, *, #14769, .T. ) ;
#10734=ORIENTED_EDGE ( 'NONE', *, *, #11528, .F. ) ;
#10735=CARTESIAN_POINT ( 'NONE',  ( -81.44903907897365514, -32.00000000000000711, 97.25957015486996227 ) ) ;
#10737=CARTESIAN_POINT ( 'NONE',  ( -82.39999999999999147, -34.83749999999999858, 103.0000000000000000 ) ) ;
#10741=CARTESIAN_POINT ( 'NONE',  ( -84.51155386534844638, -35.25364837475780888, 98.22820752270799005 ) ) ;
#10746=DIRECTION ( 'NONE',  ( -0.000000000000000000, 0.000000000000000000, -1.000000000000000000 ) ) ;
#10752=CARTESIAN_POINT ( 'NONE',  ( -81.02178482187500208, -33.59062499938548285, -97.61286128772489690 ) ) ;
#10760=ORIENTED_EDGE ( 'NONE', *, *, #11869, .T. ) ;
#10761=CARTESIAN_POINT ( 'NONE',  ( 82.40000000000000568, -33.43124999877096570, -102.9999999999999858 ) ) ;
#10762=CARTESIAN_POINT ( 'NONE',  ( 79.39999999999999147, -31.12500000000000355, -99.99999999999998579 ) ) ;
#10763=CARTESIAN_POINT ( 'NONE',  ( -80.90000000000000568, -34.59374999877096712, 97.40192378864668399 ) ) ;
#10764=CARTESIAN_POINT ( 'NONE',  ( 79.39999999999999147, -32.88750000000000284, 101.7320508075688821 ) ) ;
#10768=CARTESIAN_POINT ( 'NONE',  ( 81.02178482187500208, -32.35312499938548569, -102.3871387122750889 ) ) ;
#10772=CARTESIAN_POINT ( 'NONE',  ( 81.02178482187500208, -33.89062499938548711, -97.61286128772489690 ) ) ;
#10773=VERTEX_POINT ( 'NONE', #6421 ) ;
#10775=CARTESIAN_POINT ( 'NONE',  ( -80.90000000000000568, -34.35000000000000853, 102.5980762113533018 ) ) ;
#10776=ADVANCED_FACE ( 'NONE', ( #17064 ), #4964, .F. ) ;
#10777=EDGE_CURVE ( 'NONE', #2466, #10773, #9243, .T. ) ;
#10781=CARTESIAN_POINT ( 'NONE',  ( -80.90000000000000568, -31.05000000000000071, 97.40192378864668399 ) ) ;
#10782=VERTEX_POINT ( 'NONE', #13739 ) ;
#10783=CARTESIAN_POINT ( 'NONE',  ( -85.29357727954830182, -34.99999999999999289, 100.3154961327914805 ) ) ;
#10786=CARTESIAN_POINT ( 'NONE',  ( 82.39999999999999147, -30.47812499938548569, 96.81714838363319586 ) ) ;
#10788=EDGE_CURVE ( 'NONE', #12074, #14621, #5057, .T. ) ;
#10790=CARTESIAN_POINT ( 'NONE',  ( -84.44763168836719558, -32.00000000000001421, -98.15470523285542015 ) ) ;
#10791=CARTESIAN_POINT ( 'NONE',  ( 81.02178482187500208, -34.15312499938548285, 97.61286128772489690 ) ) ;
#10793=CARTESIAN_POINT ( 'NONE',  ( 79.64356964374999848, -32.27812499938548996, -99.99999999999998579 ) ) ;
#10795=CARTESIAN_POINT ( 'NONE',  ( -83.77821517812500929, -32.01562499938548001, 97.61286128772489690 ) ) ;
#10796=CARTESIAN_POINT ( 'NONE',  ( -82.39999999999999147, -32.84062499938548996, -96.81714838363319586 ) ) ;
#10798=CARTESIAN_POINT ( 'NONE',  ( 82.39999999999999147, -30.36562499938549209, 103.1828516163667899 ) ) ;
#10801=CARTESIAN_POINT ( 'NONE',  ( -81.02178482187500208, -33.70312499938548711, 102.3871387122750889 ) ) ;
#10804=CARTESIAN_POINT ( 'NONE',  ( -85.40000000000000568, -30.93750000000000355, -101.7320508075688679 ) ) ;
#10805=PRODUCT_DEFINITION_FORMATION_WITH_SPECIFIED_SOURCE ( 'ANY', '', #10904, .NOT_KNOWN. ) ;
#10806=CARTESIAN_POINT ( 'NONE',  ( 79.39999999999999147, -34.27499999999999858, -99.99999999999998579 ) ) ;
#10807=CARTESIAN_POINT ( 'NONE',  ( -96.99999999999998579, -5.200000000000000178, 150.0000000000000000 ) ) ;
#10815=CARTESIAN_POINT ( 'NONE',  ( 79.64356964374998427, -32.65312499938548285, 98.40857419181659793 ) ) ;
#10818=CARTESIAN_POINT ( 'NONE',  ( 85.40000000000000568, -34.89374999877097139, -99.99999999999998579 ) ) ;
#10826=CARTESIAN_POINT ( 'NONE',  ( -83.20384757729335945, -34.85759618943233562, 102.9999999999999716 ) ) ;
#10830=CARTESIAN_POINT ( 'NONE',  ( -80.07765479365644978, -32.00000000000000000, 98.15128725331825876 ) ) ;
#10831=CARTESIAN_POINT ( 'NONE',  ( -99.99999999999998579, 0.000000000000000000, 150.0000000000000000 ) ) ;
#10832=CARTESIAN_POINT ( 'NONE',  ( -85.40000000000000568, -34.08749999999999858, -101.7320508075688821 ) ) ;
#10833=VERTEX_POINT ( 'NONE', #10715 ) ;
#10835=AXIS2_PLACEMENT_3D ( 'NONE', #12344, #12531, #7943 ) ;
#10836=CARTESIAN_POINT ( 'NONE',  ( -80.90000000000000568, -33.39374999877097139, -97.40192378864668399 ) ) ;
#10846=EDGE_CURVE ( 'NONE', #2207, #17768, #9417, .T. ) ;
#10851=CARTESIAN_POINT ( 'NONE',  ( -81.59615242270662350, -33.46740381056766722, -96.99999999999998579 ) ) ;
#10853=CARTESIAN_POINT ( 'NONE',  ( 82.40000000000000568, -30.00000000000000355, 99.99999999999998579 ) ) ;
#10855=CARTESIAN_POINT ( 'NONE',  ( 82.40000000000001990, -33.26250000000000284, 103.0000000000000000 ) ) ;
#10857=VECTOR ( 'NONE', #1781, 1000.000000000000000 ) ;
#10858=ORIENTED_EDGE ( 'NONE', *, *, #11127, .F. ) ;
#10861=CARTESIAN_POINT ( 'NONE',  ( 83.90000000000000568, -30.07499999999999929, -97.40192378864668399 ) ) ;
#10863=CARTESIAN_POINT ( 'NONE',  ( -79.39999999999999147, -35.15624999877096712, 101.7320508075688537 ) ) ;
#10866=CARTESIAN_POINT ( 'NONE',  ( 85.15643035625001289, -33.36562499938548854, -101.5914258081833879 ) ) ;
#10868=CARTESIAN_POINT ( 'NONE',  ( 84.28136653320187577, -32.00000000000000000, -97.98546077809228905 ) ) ;
#10869=CARTESIAN_POINT ( 'NONE',  ( -83.77821517812500929, -33.36562499938548854, 97.61286128772489690 ) ) ;
#10870=CARTESIAN_POINT ( 'NONE',  ( 79.64356964375001269, -33.10312499938549280, -101.5914258081833879 ) ) ;
#10873=FACE_OUTER_BOUND ( 'NONE', #4434, .T. ) ;
#10878=CARTESIAN_POINT ( 'NONE',  ( -83.90000000000000568, -33.07500000000000284, 102.5980762113533018 ) ) ;
#10879=ORIENTED_EDGE ( 'NONE', *, *, #13997, .T. ) ;
#10880=CARTESIAN_POINT ( 'NONE',  ( -85.24876232368484352, -35.00000000000000000, 100.5466586069497623 ) ) ;
#10881=( BOUNDED_CURVE ( )  B_SPLINE_CURVE ( 2, ( #11100, #10721, #12288, #14126, #16685, #7791, #17068, #4870, #15409 ),
 .UNSPECIFIED., .F., .F. ) 
 B_SPLINE_CURVE_WITH_KNOTS ( ( 3, 2, 2, 2, 3 ),
 ( 0.4374999999999999445, 0.4444444444444444198, 0.4583333333333333148, 0.4722222222222222099, 0.4791666666666666297 ),
 .UNSPECIFIED. ) 
 CURVE ( )  GEOMETRIC_REPRESENTATION_ITEM ( )  RATIONAL_B_SPLINE_CURVE ( ( 0.9330127018922192983, 0.9330127018922187432, 1.000000000000000000, 0.8660254037844387076, 1.000000000000000000, 0.8660254037844387076, 1.000000000000000000, 0.9330127018922196314, 0.9330127018922194093 ) ) 
 REPRESENTATION_ITEM ( '' )  );
#10883=CARTESIAN_POINT ( 'NONE',  ( 79.90595866893272614, -34.99999999999998579, 98.81289630734771379 ) ) ;
#10884=CARTESIAN_POINT ( 'NONE',  ( 85.15643035624999868, -30.17812499938548498, 101.5914258081833879 ) ) ;
#10885=ADVANCED_FACE ( 'NONE', ( #1233 ), #15986, .F. ) ;
#10889=CARTESIAN_POINT ( 'NONE',  ( 79.64356964375001269, -30.40312499938548285, 98.40857419181659793 ) ) ;
#10890=CARTESIAN_POINT ( 'NONE',  ( 85.15643035624999868, -32.46562499938548996, -101.5914258081833879 ) ) ;
#10892=CARTESIAN_POINT ( 'NONE',  ( -83.77821517812500929, -33.92812499938548854, 97.61286128772489690 ) ) ;
#10893=CARTESIAN_POINT ( 'NONE',  ( -79.64356964375001269, -33.21562499938548996, -98.40857419181659793 ) ) ;
#10895=CARTESIAN_POINT ( 'NONE',  ( 85.15643035624999868, -33.36562499938548854, 98.40857419181659793 ) ) ;
#10897=CARTESIAN_POINT ( 'NONE',  ( -83.77821517812500929, -30.96562499938548640, 102.3871387122750889 ) ) ;
#10899=CARTESIAN_POINT ( 'NONE',  ( -85.15643035625001289, -32.95312499938548711, 99.99999999999998579 ) ) ;
#10901=DIRECTION ( 'NONE',  ( 0.000000000000000000, 0.000000000000000000, -1.000000000000000000 ) ) ;
#10903=CARTESIAN_POINT ( 'NONE',  ( -82.39999999999999147, -33.71249999999999858, -103.4641016151377499 ) ) ;
#10904=PRODUCT ( 'workbench', 'workbench', '', ( #9657 ) ) ;
#10908=EDGE_CURVE ( 'NONE', #2292, #7532, #10058, .T. ) ;
#10915=CARTESIAN_POINT ( 'NONE',  ( 81.59615242270665192, -34.18259618943233136, 103.0000000000000000 ) ) ;
#10916=CARTESIAN_POINT ( 'NONE',  ( -83.90000000000000568, -34.36874999877097281, 102.5980762113533018 ) ) ;
#10917=CARTESIAN_POINT ( 'NONE',  ( 85.15643035624999868, -32.46562499938548996, -101.5914258081833879 ) ) ;
#10920=CARTESIAN_POINT ( 'NONE',  ( 85.40000000000000568, -30.43124999877096926, 101.7320508075688679 ) ) ;
#10926=CARTESIAN_POINT ( 'NONE',  ( -82.39999999999999147, -32.81250000000000000, -103.0000000000000000 ) ) ;
#10928=VERTEX_POINT ( 'NONE', #14219 ) ;
#10929=CARTESIAN_POINT ( 'NONE',  ( -80.80006050682004570, -32.00000000000000711, 97.54622936382074272 ) ) ;
#10932=CARTESIAN_POINT ( 'NONE',  ( -83.90000000000000568, -33.67500000000000426, -102.5980762113533018 ) ) ;
#10935=CARTESIAN_POINT ( 'NONE',  ( -79.39999999999999147, -33.31874999877096855, -99.99999999999998579 ) ) ;
#10946=FACE_OUTER_BOUND ( 'NONE', #19085, .T. ) ;
#10951=CYLINDRICAL_SURFACE ( 'NONE', #11946, 3.000000000000002665 ) ;
#10954=CARTESIAN_POINT ( 'NONE',  ( -80.80636817121812498, -31.99999999999999289, 102.4696265554868688 ) ) ;
#10955=CARTESIAN_POINT ( 'NONE',  ( 85.15643035624999868, -34.60312499938548569, -101.5914258081833879 ) ) ;
#10958=CARTESIAN_POINT ( 'NONE',  ( -85.40000000000000568, -34.44374999877096855, 99.99999999999998579 ) ) ;
#10960=CARTESIAN_POINT ( 'NONE',  ( 80.90000000000000568, -33.39374999877097139, 97.40192378864668399 ) ) ;
#10961=CARTESIAN_POINT ( 'NONE',  ( 82.39999999999999147, -32.39062499938548711, -103.1828516163667899 ) ) ;
#10963=CARTESIAN_POINT ( 'NONE',  ( -79.64356964375001269, -32.65312499938548285, 101.5914258081833879 ) ) ;
#10964=CARTESIAN_POINT ( 'NONE',  ( 83.77821517812500929, -33.81562499938548427, -97.61286128772489690 ) ) ;
#10967=CARTESIAN_POINT ( 'NONE',  ( -85.40000000000000568, -34.53750000000000142, 98.26794919243111792 ) ) ;
#10971=CARTESIAN_POINT ( 'NONE',  ( -80.90000000000000568, -32.85000000000000142, 97.40192378864668399 ) ) ;
#10975=CARTESIAN_POINT ( 'NONE',  ( 79.64356964375001269, -31.75312499938548427, 98.40857419181659793 ) ) ;
#10976=VECTOR ( 'NONE', #5171, 1000.000000000000000 ) ;
#10980=CARTESIAN_POINT ( 'NONE',  ( -81.02178482187500208, -32.65312499938548996, -102.3871387122750889 ) ) ;
#10981=CARTESIAN_POINT ( 'NONE',  ( 81.02178482187500208, -30.44062499938548783, 97.61286128772489690 ) ) ;
#10982=CARTESIAN_POINT ( 'NONE',  ( 79.64356964375001269, -31.86562499938548143, -101.5914258081833879 ) ) ;
#10984=CARTESIAN_POINT ( 'NONE',  ( -83.77821517812500929, -33.32812499938548711, 102.3871387122750889 ) ) ;
#10985=CARTESIAN_POINT ( 'NONE',  ( -85.15643035624999868, -34.71562499938548285, -98.40857419181659793 ) ) ;
#10988=CARTESIAN_POINT ( 'NONE',  ( 85.15643035625001289, -32.50312499938548427, 99.99999999999998579 ) ) ;
#10992=CARTESIAN_POINT ( 'NONE',  ( -82.39999999999999147, -31.37812499938548427, 103.1828516163667899 ) ) ;
#10994=CARTESIAN_POINT ( 'NONE',  ( -79.64356964375001269, -34.49062499938548854, 98.40857419181659793 ) ) ;
#10997=CARTESIAN_POINT ( 'NONE',  ( -85.40000000000000568, -32.66250000000000142, -98.26794919243111792 ) ) ;
#11004=CARTESIAN_POINT ( 'NONE',  ( -85.40000000000000568, -33.50624999877096855, -98.26794919243111792 ) ) ;
#11005=LINE ( 'NONE', #16973, #5889 ) ;
#11008=CARTESIAN_POINT ( 'NONE',  ( 82.39999999999999147, -31.26562499938549067, -96.81714838363319586 ) ) ;
#11009=CARTESIAN_POINT ( 'NONE',  ( 94.79999999999995453, -32.00000000000000000, -150.0000000000000000 ) ) ;
#11011=ORIENTED_EDGE ( 'NONE', *, *, #17240, .T. ) ;
#11021=CARTESIAN_POINT ( 'NONE',  ( -85.15643035624999868, -30.62812499938548427, -101.5914258081833879 ) ) ;
#11026=CARTESIAN_POINT ( 'NONE',  ( 85.15643035625001289, -34.30312499938548854, 99.99999999999998579 ) ) ;
#11027=CARTESIAN_POINT ( 'NONE',  ( -79.39999999999999147, -32.83124999877097139, -101.7320508075688821 ) ) ;
#11033=EDGE_CURVE ( 'NONE', #13093, #18033, #14665, .T. ) ;
#11038=VERTEX_POINT ( 'NONE', #4750 ) ;
#11039=CARTESIAN_POINT ( 'NONE',  ( 81.02178482187500208, -32.69062499938548427, -102.3871387122750889 ) ) ;
#11042=ORIENTED_EDGE ( 'NONE', *, *, #17017, .F. ) ;
#11043=PLANE ( 'NONE',  #19269 ) ;
#11045=DIRECTION ( 'NONE',  ( -0.000000000000000000, 0.000000000000000000, -1.000000000000000000 ) ) ;
#11046=ORIENTED_EDGE ( 'NONE', *, *, #4026, .F. ) ;
#11049=ORIENTED_EDGE ( 'NONE', *, *, #11373, .T. ) ;
#11051=CARTESIAN_POINT ( 'NONE',  ( 85.40000000000000568, -31.35000000000000142, -99.99999999999998579 ) ) ;
#11052=CARTESIAN_POINT ( 'NONE',  ( -82.39999999999999147, -34.10624999877096997, 96.53589838486223584 ) ) ;
#11054=CARTESIAN_POINT ( 'NONE',  ( -80.90000000000000568, -33.24374999877097281, 97.40192378864668399 ) ) ;
#11056=CARTESIAN_POINT ( 'NONE',  ( 81.02178482187500208, -32.20312499938548711, -97.61286128772489690 ) ) ;
#11057=CARTESIAN_POINT ( 'NONE',  ( 82.40000000000000568, -30.00000000000000355, -103.0000000000000000 ) ) ;
#11058=CARTESIAN_POINT ( 'NONE',  ( -83.77821517812500929, -32.46562499938548285, 97.61286128772489690 ) ) ;
#11059=CARTESIAN_POINT ( 'NONE',  ( 83.77821517812500929, -33.66562499938548569, -102.3871387122750889 ) ) ;
#11060=VERTEX_POINT ( 'NONE', #13525 ) ;
#11065=CARTESIAN_POINT ( 'NONE',  ( 82.40000000000000568, -33.03750000000000142, -102.9999999999999858 ) ) ;
#11069=CARTESIAN_POINT ( 'NONE',  ( -79.39999999999999147, -32.43750000000000000, 98.26794919243110371 ) ) ;
#11074=CARTESIAN_POINT ( 'NONE',  ( 85.15643035624999868, -31.97812499938548925, 101.5914258081833879 ) ) ;
#11076=CARTESIAN_POINT ( 'NONE',  ( 81.59615242270663771, -32.11740381056766580, -103.0000000000000000 ) ) ;
#11079=CARTESIAN_POINT ( 'NONE',  ( 81.02178482187500208, -31.64062499938548356, 102.3871387122750889 ) ) ;
#11080=CARTESIAN_POINT ( 'NONE',  ( 79.64356964375001269, -31.34062499938548640, -98.40857419181659793 ) ) ;
#11082=CARTESIAN_POINT ( 'NONE',  ( -81.02178482187500208, -33.70312499938548711, 102.3871387122750889 ) ) ;
#11083=CARTESIAN_POINT ( 'NONE',  ( -85.15643035624999868, -32.54062499938548569, -101.5914258081833879 ) ) ;
#11084=VERTEX_POINT ( 'NONE', #7282 ) ;
#11085=CARTESIAN_POINT ( 'NONE',  ( 83.77821517812500929, -32.12812499938548427, 102.3871387122750889 ) ) ;
#11088=CARTESIAN_POINT ( 'NONE',  ( -81.02178482187500208, -31.19062499938548427, 97.61286128772489690 ) ) ;
#11089=CARTESIAN_POINT ( 'NONE',  ( -83.77821517812500929, -34.22812499938549280, 102.3871387122750889 ) ) ;
#11090=DIRECTION ( 'NONE',  ( -0.000000000000000000, -1.000000000000000000, -0.000000000000000000 ) ) ;
#11092=CARTESIAN_POINT ( 'NONE',  ( -83.90000000000000568, -33.52499999999999858, -97.40192378864668399 ) ) ;
#11093=CARTESIAN_POINT ( 'NONE',  ( -99.99999999999998579, -29.80000000000000426, 150.0000000000000000 ) ) ;
#11098=VERTEX_POINT ( 'NONE', #13434 ) ;
#11100=CARTESIAN_POINT ( 'NONE',  ( 82.40000000000001990, -32.75624999877096855, -97.00000000000000000 ) ) ;
#11101=CARTESIAN_POINT ( 'NONE',  ( -83.20384757729335945, -33.24240381056766580, 96.99999999999998579 ) ) ;
#11102=CARTESIAN_POINT ( 'NONE',  ( 82.39999999999999147, -30.81562499938548427, 103.1828516163667899 ) ) ;
#11103=AXIS2_PLACEMENT_3D ( 'NONE', #2355, #15357, #9787 ) ;
#11105=CARTESIAN_POINT ( 'NONE',  ( 85.15643035625001289, -30.25312499938548783, -99.99999999999998579 ) ) ;
#11107=ORIENTED_EDGE ( 'NONE', *, *, #2958, .T. ) ;
#11108=CARTESIAN_POINT ( 'NONE',  ( 83.90000000000000568, -31.81874999877096855, 102.5980762113533018 ) ) ;
#11115=EDGE_LOOP ( 'NONE', ( #17116, #1939, #11107, #17498 ) ) ;
#11117=CARTESIAN_POINT ( 'NONE',  ( -79.64356964375001269, -31.22812499938548925, -101.5914258081833879 ) ) ;
#11120=CARTESIAN_POINT ( 'NONE',  ( 79.64356964374998427, -33.21562499938548996, 98.40857419181659793 ) ) ;
#11121=CARTESIAN_POINT ( 'NONE',  ( -82.39999999999999147, -32.75624999877096855, -103.4641016151377499 ) ) ;
#11122=CARTESIAN_POINT ( 'NONE',  ( 94.79999999999995453, -29.80000000000000071, -150.0000000000000000 ) ) ;
#11123=CARTESIAN_POINT ( 'NONE',  ( -82.40000000000000568, -30.00000000000000355, 103.0000000000000000 ) ) ;
#11126=DIRECTION ( 'NONE',  ( 1.000000000000000000, -1.445602896647337931E-15, 0.000000000000000000 ) ) ;
#11127=EDGE_CURVE ( 'NONE', #19014, #5107, #10164, .T. ) ;
#11128=EDGE_CURVE ( 'NONE', #5078, #6543, #65, .T. ) ;
#11133=CARTESIAN_POINT ( 'NONE',  ( 82.39999999999999147, -33.40312499938548285, -96.81714838363319586 ) ) ;
#11141=VERTEX_POINT ( 'NONE', #4356 ) ;
#11145=EDGE_CURVE ( 'NONE', #15108, #6865, #2886, .T. ) ;
#11146=VERTEX_POINT ( 'NONE', #1425 ) ;
#11148=CARTESIAN_POINT ( 'NONE',  ( 83.77821517812500929, -34.56562499938548427, -102.3871387122750889 ) ) ;
#11150=VECTOR ( 'NONE', #11972, 1000.000000000000000 ) ;
#11151=( GEOMETRIC_REPRESENTATION_CONTEXT ( 3 ) GLOBAL_UNCERTAINTY_ASSIGNED_CONTEXT ( ( #3353 ) ) GLOBAL_UNIT_ASSIGNED_CONTEXT ( ( #9798, #14090, #2850 ) ) REPRESENTATION_CONTEXT ( 'NONE', 'WORKASPACE' ) );
#11152=CARTESIAN_POINT ( 'NONE',  ( -83.90000000000000568, -34.81874999877096855, 102.5980762113533018 ) ) ;
#11157=CARTESIAN_POINT ( 'NONE',  ( 79.64356964374998427, -32.20312499938548711, 98.40857419181659793 ) ) ;
#11158=CARTESIAN_POINT ( 'NONE',  ( -79.39999999999999147, -33.80624999877097281, 101.7320508075688537 ) ) ;
#11159=CARTESIAN_POINT ( 'NONE',  ( -79.64356964374999848, -33.51562499938548711, 99.99999999999998579 ) ) ;
#11161=ORIENTED_EDGE ( 'NONE', *, *, #6147, .T. ) ;
#11164=CARTESIAN_POINT ( 'NONE',  ( -83.90000000000000568, -33.52499999999999858, 102.5980762113533018 ) ) ;
#11171=ORIENTED_EDGE ( 'NONE', *, *, #7224, .T. ) ;
#11174=CARTESIAN_POINT ( 'NONE',  ( 81.96801452314024061, -34.99999999999999289, 97.27181766474434710 ) ) ;
#11175=CARTESIAN_POINT ( 'NONE',  ( 79.64356964375001269, -32.57812499938548001, 101.5914258081833879 ) ) ;
#11177=AXIS2_PLACEMENT_3D ( 'NONE', #9544, #7694, #6623 ) ;
#11179=CARTESIAN_POINT ( 'NONE',  ( 82.39999999999999147, -32.58749999999999858, 96.99999999999998579 ) ) ;
#11182=CARTESIAN_POINT ( 'NONE',  ( 79.64356964375001269, -31.67812499938548143, 101.5914258081833879 ) ) ;
#11183=CARTESIAN_POINT ( 'NONE',  ( 82.39999999999999147, -34.41562499938547859, -96.81714838363319586 ) ) ;
#11184=EDGE_CURVE ( 'NONE', #592, #11539, #11967, .T. ) ;
#11186=CARTESIAN_POINT ( 'NONE',  ( -79.64356964374998427, -33.59062499938548285, 98.40857419181659793 ) ) ;
#11187=CARTESIAN_POINT ( 'NONE',  ( -85.15643035624999868, -31.52812499938547930, -101.5914258081833879 ) ) ;
#11189=CARTESIAN_POINT ( 'NONE',  ( 81.02178482187500208, -33.55312499938548854, 102.3871387122750889 ) ) ;
#11192=CARTESIAN_POINT ( 'NONE',  ( -85.15643035625001289, -31.94062499938548427, 99.99999999999998579 ) ) ;
#11193=CARTESIAN_POINT ( 'NONE',  ( -82.39999999999999147, -34.64062499938548711, 103.1828516163667899 ) ) ;
#11194=CARTESIAN_POINT ( 'NONE',  ( 82.40000000000001990, -32.75624999877096855, -97.00000000000000000 ) ) ;
#11195=ORIENTED_EDGE ( 'NONE', *, *, #3753, .T. ) ;
#11196=CARTESIAN_POINT ( 'NONE',  ( -82.39999999999999147, -34.61250000000000426, -103.4641016151377499 ) ) ;
#11197=CARTESIAN_POINT ( 'NONE',  ( 81.59615242270662350, -33.01740381056767148, -102.9999999999999858 ) ) ;
#11202=EDGE_CURVE ( 'NONE', #1356, #10773, #10503, .T. ) ;
#11203=APPLICATION_CONTEXT ( 'automotive_design' ) ;
#11204=CARTESIAN_POINT ( 'NONE',  ( -82.65333140691201663, -34.99995246259153703, 97.01071553687880566 ) ) ;
#11207=CARTESIAN_POINT ( 'NONE',  ( 82.39999999999999147, -30.59062499938548640, 96.81714838363319586 ) ) ;
#11209=PLANE ( 'NONE',  #2769 ) ;
#11210=CARTESIAN_POINT ( 'NONE',  ( 85.15643035625001289, -31.60312499938548569, -99.99999999999998579 ) ) ;
#11212=VERTEX_POINT ( 'NONE', #4547 ) ;
#11213=CARTESIAN_POINT ( 'NONE',  ( 79.39999999999999147, -31.93124999877096926, 101.7320508075688821 ) ) ;
#11218=CARTESIAN_POINT ( 'NONE',  ( 83.20384757729338787, -33.95759618943233704, 97.00000000000000000 ) ) ;
#11220=CARTESIAN_POINT ( 'NONE',  ( -82.39999999999999147, -31.60312499938548569, -103.1828516163667899 ) ) ;
#11223=CARTESIAN_POINT ( 'NONE',  ( 81.02178482187500208, -34.00312499938548427, 102.3871387122750889 ) ) ;
#11224=CARTESIAN_POINT ( 'NONE',  ( -83.90000000000000568, -32.71874999877096712, -102.5980762113533018 ) ) ;
#11225=CARTESIAN_POINT ( 'NONE',  ( 80.90000000000000568, -34.20000000000000284, 102.5980762113533018 ) ) ;
#11226=CARTESIAN_POINT ( 'NONE',  ( -79.91954014136210560, -34.99999999999999289, 98.55723758691019043 ) ) ;
#11229=CARTESIAN_POINT ( 'NONE',  ( 84.85538848573307291, -35.00000000000139977, -98.27756861396950683 ) ) ;
#11235=ORIENTED_EDGE ( 'NONE', *, *, #5596, .F. ) ;
#11236=CARTESIAN_POINT ( 'NONE',  ( 85.15643035625001289, -32.35312499938548569, -101.5914258081833879 ) ) ;
#11244=CARTESIAN_POINT ( 'NONE',  ( -83.90000000000000568, -33.91874999877096997, -97.40192378864668399 ) ) ;
#11248=CARTESIAN_POINT ( 'NONE',  ( 79.39999999999999147, -31.61250000000000071, -101.7320508075688537 ) ) ;
#11250=CARTESIAN_POINT ( 'NONE',  ( -81.02178482187500208, -31.90312499938548996, 102.3871387122750889 ) ) ;
#11254=CARTESIAN_POINT ( 'NONE',  ( 79.64356964374998427, -34.94062499938548427, -98.40857419181659793 ) ) ;
#11256=CARTESIAN_POINT ( 'NONE',  ( -82.39999999999999147, -32.95312499938548711, 96.81714838363319586 ) ) ;
#11257=DIRECTION ( 'NONE',  ( 0.000000000000000000, 1.000000000000000000, 0.000000000000000000 ) ) ;
#11259=( NAMED_UNIT ( * ) SI_UNIT ( $, .STERADIAN. ) SOLID_ANGLE_UNIT ( ) );
#11260=DIRECTION ( 'NONE',  ( 0.000000000000000000, -1.000000000000000000, 0.000000000000000000 ) ) ;
#11264=EDGE_CURVE ( 'NONE', #13128, #18799, #16047, .T. ) ;
#11265=ORIENTED_EDGE ( 'NONE', *, *, #11558, .T. ) ;
#11266=CARTESIAN_POINT ( 'NONE',  ( -81.28488860390726245, -34.99999999999999289, -97.47285052570516939 ) ) ;
#11268=CARTESIAN_POINT ( 'NONE',  ( 79.64356964375001269, -31.67812499938548143, 101.5914258081833879 ) ) ;
#11271=( BOUNDED_CURVE ( )  B_SPLINE_CURVE ( 2, ( #10470, #11557, #16247, #17520, #7162, #10093, #16051, #2654, #19081 ),
 .UNSPECIFIED., .F., .F. ) 
 B_SPLINE_CURVE_WITH_KNOTS ( ( 3, 2, 2, 2, 3 ),
 ( 0.4375000000000000555, 0.4444444444444444198, 0.4583333333333333148, 0.4722222222222222099, 0.4791666666666666297 ),
 .UNSPECIFIED. ) 
 CURVE ( )  GEOMETRIC_REPRESENTATION_ITEM ( )  RATIONAL_B_SPLINE_CURVE ( ( 0.9330127018922192983, 0.9330127018922198534, 1.000000000000000000, 0.8660254037844387076, 1.000000000000000000, 0.8660254037844387076, 1.000000000000000000, 0.9330127018922196314, 0.9330127018922194093 ) ) 
 REPRESENTATION_ITEM ( '' )  );
#11274=CARTESIAN_POINT ( 'NONE',  ( -81.02178482187500208, -34.15312499938548285, -97.61286128772489690 ) ) ;
#11275=CARTESIAN_POINT ( 'NONE',  ( 83.77821517812500929, -33.21562499938548285, 97.61286128772489690 ) ) ;
#11276=EDGE_CURVE ( 'NONE', #3690, #867, #17633, .T. ) ;
#11277=CARTESIAN_POINT ( 'NONE',  ( 85.15643035624999868, -32.99062499938548854, -98.40857419181659793 ) ) ;
#11279=CARTESIAN_POINT ( 'NONE',  ( -85.15643035625001289, -32.80312499938548854, 101.5914258081833879 ) ) ;
#11280=CARTESIAN_POINT ( 'NONE',  ( 82.39999999999999147, -30.70312499938548711, -96.81714838363319586 ) ) ;
#11281=EDGE_CURVE ( 'NONE', #4201, #779, #18056, .T. ) ;
#11282=VERTEX_POINT ( 'NONE', #11179 ) ;
#11283=CARTESIAN_POINT ( 'NONE',  ( 79.64356964374999848, -32.72812499938548569, 99.99999999999998579 ) ) ;
#11286=CARTESIAN_POINT ( 'NONE',  ( -81.02178482187500208, -30.74062499938548498, 97.61286128772489690 ) ) ;
#11287=CARTESIAN_POINT ( 'NONE',  ( -79.64356964375001269, -30.32812499938548711, 98.40857419181659793 ) ) ;
#11290=CARTESIAN_POINT ( 'NONE',  ( -82.39999999999999147, -32.36250000000000426, -103.4641016151377499 ) ) ;
#11296=CARTESIAN_POINT ( 'NONE',  ( 83.90000000000000568, -33.52499999999999858, -102.5980762113533018 ) ) ;
#11298=CARTESIAN_POINT ( 'NONE',  ( 85.40000000000000568, -34.03124999877096712, -98.26794919243111792 ) ) ;
#11301=CARTESIAN_POINT ( 'NONE',  ( 79.64356964375001269, -31.34062499938548640, 101.5914258081833879 ) ) ;
#11303=CARTESIAN_POINT ( 'NONE',  ( -83.90000000000000568, -32.62500000000000000, -97.40192378864668399 ) ) ;
#11304=CARTESIAN_POINT ( 'NONE',  ( 79.64356964375001269, -32.24062499938548854, -98.40857419181659793 ) ) ;
#11308=( BOUNDED_CURVE ( )  B_SPLINE_CURVE ( 2, ( #8151, #14103, #3458, #739, #13719, #15383, #2478, #14481, #3845 ),
 .UNSPECIFIED., .F., .F. ) 
 B_SPLINE_CURVE_WITH_KNOTS ( ( 3, 2, 2, 2, 3 ),
 ( 0.3958333333333334259, 0.4027777777777777901, 0.4166666666666666852, 0.4305555555555555802, 0.4374999999999999445 ),
 .UNSPECIFIED. ) 
 CURVE ( )  GEOMETRIC_REPRESENTATION_ITEM ( )  RATIONAL_B_SPLINE_CURVE ( ( 0.9330127018922192983, 0.9330127018922200755, 1.000000000000000000, 0.8660254037844387076, 1.000000000000000000, 0.8660254037844387076, 1.000000000000000000, 0.9330127018922198534, 0.9330127018922192983 ) ) 
 REPRESENTATION_ITEM ( '' )  );
#11309=ORIENTED_EDGE ( 'NONE', *, *, #14586, .F. ) ;
#11310=CARTESIAN_POINT ( 'NONE',  ( 82.39999999999999147, -30.95624999877097139, 103.4641016151377499 ) ) ;
#11315=CARTESIAN_POINT ( 'NONE',  ( -85.15643035624999868, -30.29062499938548925, 98.40857419181659793 ) ) ;
#11317=ORIENTED_EDGE ( 'NONE', *, *, #1293, .T. ) ;
#11318=CARTESIAN_POINT ( 'NONE',  ( -85.15643035624999868, -32.80312499938548854, -98.40857419181659793 ) ) ;
#11319=CARTESIAN_POINT ( 'NONE',  ( 83.20384757729335945, -33.24240381056766580, 102.9999999999999716 ) ) ;
#11321=CARTESIAN_POINT ( 'NONE',  ( 83.77821517812500929, -34.67812499938548854, 97.61286128772489690 ) ) ;
#11323=CARTESIAN_POINT ( 'NONE',  ( -79.64356964375001269, -30.89062499938548711, -101.5914258081833879 ) ) ;
#11324=CARTESIAN_POINT ( 'NONE',  ( 85.40000000000000568, -34.95000000000000284, 99.99999999999998579 ) ) ;
#11325=CARTESIAN_POINT ( 'NONE',  ( -80.32125193361312654, -35.00000000000000711, 97.97655282300750912 ) ) ;
#11332=EDGE_LOOP ( 'NONE', ( #11340, #7114, #3468, #942 ) ) ;
#11333=CARTESIAN_POINT ( 'NONE',  ( 79.64356964374998427, -33.10312499938548569, -101.5914258081833879 ) ) ;
#11337=CARTESIAN_POINT ( 'NONE',  ( 83.20384757729335945, -32.60759618943233562, 96.99999999999997158 ) ) ;
#11340=ORIENTED_EDGE ( 'NONE', *, *, #11202, .F. ) ;
#11343=ORIENTED_EDGE ( 'NONE', *, *, #9244, .T. ) ;
#11344=CARTESIAN_POINT ( 'NONE',  ( -79.39999999999999147, -32.06250000000000000, -98.26794919243113213 ) ) ;
#11345=CARTESIAN_POINT ( 'NONE',  ( 79.39999999999999147, -33.33749999999999858, -98.26794919243110371 ) ) ;
#11348=CARTESIAN_POINT ( 'NONE',  ( -82.39999999999999147, -32.61562499938548854, 96.81714838363319586 ) ) ;
#11350=LINE ( 'NONE', #13194, #4940 ) ;
#11352=CARTESIAN_POINT ( 'NONE',  ( 85.15643035625001289, -34.34062499938548285, -98.40857419181659793 ) ) ;
#11353=CARTESIAN_POINT ( 'NONE',  ( -81.59615242270665192, -33.86115380933864571, 103.0000000000000000 ) ) ;
#11354=CARTESIAN_POINT ( 'NONE',  ( 85.31192385480825635, -35.00000000000000711, 100.3932545473399642 ) ) ;
#11359=CARTESIAN_POINT ( 'NONE',  ( -84.70388354820684640, -35.00002705695768412, -101.9214814096701076 ) ) ;
#11363=VERTEX_POINT ( 'NONE', #3656 ) ;
#11364=CARTESIAN_POINT ( 'NONE',  ( -80.17984880387896851, -35.00000000000000000, -98.35655086105390410 ) ) ;
#11367=CARTESIAN_POINT ( 'NONE',  ( 82.39999999999999147, -33.85312499938547859, 103.1828516163667899 ) ) ;
#11368=CARTESIAN_POINT ( 'NONE',  ( 83.20384757729338787, -33.95759618943233704, -102.9999999999999858 ) ) ;
#11369=CARTESIAN_POINT ( 'NONE',  ( -82.40000000000000568, -30.00000000000000355, -99.99999999999998579 ) ) ;
#11371=CARTESIAN_POINT ( 'NONE',  ( -79.64356964374999848, -34.52812499938548285, -99.99999999999998579 ) ) ;
#11372=CARTESIAN_POINT ( 'NONE',  ( 85.15643035624999868, -32.87812499938549138, 101.5914258081833879 ) ) ;
#11373=EDGE_CURVE ( 'NONE', #10346, #5045, #11308, .T. ) ;
#11375=CARTESIAN_POINT ( 'NONE',  ( 83.77821517812500929, -34.82812499938548711, -97.61286128772489690 ) ) ;
#11377=CARTESIAN_POINT ( 'NONE',  ( -83.77821517812500929, -34.26562499938548711, 97.61286128772489690 ) ) ;
#11378=CARTESIAN_POINT ( 'NONE',  ( 85.15643035625001289, -30.14062499938548711, -99.99999999999998579 ) ) ;
#11383=CARTESIAN_POINT ( 'NONE',  ( -79.64356964375001269, -33.92812499938548854, 98.40857419181659793 ) ) ;
#11384=CARTESIAN_POINT ( 'NONE',  ( -82.39999999999999147, -31.60312499938548569, 96.81714838363319586 ) ) ;
#11386=CARTESIAN_POINT ( 'NONE',  ( -84.82992844608097016, -31.99999999999998579, 98.68659295968647882 ) ) ;
#11389=EDGE_CURVE ( 'NONE', #13275, #5463, #12839, .T. ) ;
#11390=CARTESIAN_POINT ( 'NONE',  ( 82.40000000000000568, -33.03750000000000142, -102.9999999999999858 ) ) ;
#11391=CARTESIAN_POINT ( 'NONE',  ( 84.12112955302457351, -35.00000000000000000, -97.53419980903892395 ) ) ;
#11396=CARTESIAN_POINT ( 'NONE',  ( 83.20384757729335945, -34.08615380933863293, -96.99999999999998579 ) ) ;
#11400=( BOUNDED_CURVE ( )  B_SPLINE_CURVE ( 2, ( #3599, #9561, #12877, #17285, #19035, #14429, #9955, #11319, #5659 ),
 .UNSPECIFIED., .F., .F. ) 
 B_SPLINE_CURVE_WITH_KNOTS ( ( 3, 2, 2, 2, 3 ),
 ( 0.5625000000000000000, 0.5694444444444444198, 0.5833333333333333703, 0.5972222222222222099, 0.6041666666666666297 ),
 .UNSPECIFIED. ) 
 CURVE ( )  GEOMETRIC_REPRESENTATION_ITEM ( )  RATIONAL_B_SPLINE_CURVE ( ( 0.9330127018922194093, 0.9330127018922194093, 1.000000000000000000, 0.8660254037844387076, 1.000000000000000000, 0.8660254037844387076, 1.000000000000000000, 0.9330127018922198534, 0.9330127018922192983 ) ) 
 REPRESENTATION_ITEM ( '' )  );
#11403=CARTESIAN_POINT ( 'NONE',  ( 82.39999999999999147, -34.86562499938548854, -96.81714838363319586 ) ) ;
#11407=CARTESIAN_POINT ( 'NONE',  ( 85.40000000000000568, -34.03124999877096712, 101.7320508075688679 ) ) ;
#11412=B_SPLINE_CURVE_WITH_KNOTS ( 'NONE', 3,
 ( #17701, #17319, #19170, #4317, #18981, #10278, #10175, #7242, #16240, #2847, #8803, #5411, #11354, #4122, #9894, #2464, #8419, #14373 ),
 .UNSPECIFIED., .F., .F.,
 ( 4, 2, 2, 2, 2, 2, 2, 2, 4 ),
 ( 0.000000000000000000, 0.0007089252359835979036, 0.001417850471967195807, 0.002126775707950793494, 0.002835700943934391614, 0.003544626179917989735, 0.004253551415901586988, 0.004962476651885185108, 0.005671401887868783229 ),
 .UNSPECIFIED. ) ;
#11415=CARTESIAN_POINT ( 'NONE',  ( -79.64356964375001269, -32.20312499938548001, -98.40857419181659793 ) ) ;
#11416=FACE_OUTER_BOUND ( 'NONE', #5673, .T. ) ;
#11417=ORIENTED_EDGE ( 'NONE', *, *, #18544, .T. ) ;
#11418=CARTESIAN_POINT ( 'NONE',  ( 82.39999999999999147, -33.06562499938548427, 103.1828516163667899 ) ) ;
#11419=CARTESIAN_POINT ( 'NONE',  ( -81.02178482187500208, -31.30312499938548498, -102.3871387122750889 ) ) ;
#11420=AXIS2_PLACEMENT_3D ( 'NONE', #15303, #472, #8077 ) ;
#11421=CARTESIAN_POINT ( 'NONE',  ( 82.39999999999999147, -34.16250000000000142, 103.4641016151377499 ) ) ;
#11422=CARTESIAN_POINT ( 'NONE',  ( 80.90000000000000568, -34.59374999877096712, -97.40192378864668399 ) ) ;
#11425=CARTESIAN_POINT ( 'NONE',  ( -85.15643035625001289, -33.29062499938547859, -99.99999999999998579 ) ) ;
#11426=( BOUNDED_CURVE ( )  B_SPLINE_CURVE ( 2, ( #10790, #15386, #7956, #1999, #15681, #455, #14201, #6404, #12357, #14012, #13910, #548, #648, #6506, #12451, #6597, #5038, #9624, #10980, #9520, #12545, #18516, #17047, #3659, #8534, #13031, #5337, #10106, #18809, #14483, #15775, #17531, #2666, #12747, #8345, #15876, #9813, #4146, #1115, #14300, #15965, #16062, #13122, #2572, #14581, #7072, #19002, #5622, #2383, #10009, #18714, #18903, #936, #8627, #11568, #1216, #7172, #6800, #11274, #6891, #17243, #8438, #14390, #3847, #12841, #4050, #2480, #5434, #11371, #1029, #17338, #5524, #3948, #11472, #9913, #17439, #6981, #12933, #14176, #2067, #18396, #6673, #12615 ),
 .UNSPECIFIED., .F., .F. ) 
 B_SPLINE_CURVE_WITH_KNOTS ( ( 3, 2, 2, 2, 2, 2, 2, 2, 2, 2, 2, 2, 2, 2, 2, 2, 2, 2, 2, 2, 2, 2, 2, 2, 2, 2, 2, 2, 2, 2, 2, 2, 2, 2, 2, 2, 2, 2, 2, 2, 2, 3 ),
 ( 0.3495698921800971526, 0.3600184345287979482, 0.3750192026341645501, 0.3900199707395311521, 0.4050207388448977541, 0.4200215069502643561, 0.4350222750556309581, 0.4500230431609975046, 0.4650238112663641066, 0.4800245793717306531, 0.4950253474770972550, 0.5100261155824639125, 0.5250268836878304590, 0.5400276517931970055, 0.5550284198985635520, 0.5700291880039302095, 0.5850299561092967560, 0.6000307242146634135, 0.6150314923200299599, 0.6300322604253966174, 0.6450330285307630529, 0.6600337966361298214, 0.6750345647414963679, 0.6900353328468629144, 0.7050361009522294609, 0.7200368690575960073, 0.7350376371629626648, 0.7500384052683292113, 0.7650391733736958688, 0.7800399414790624153, 0.7950407095844290728, 0.8100414776897955083, 0.8250422457951621658, 0.8400430139005288233, 0.8550437820058952587, 0.8700445501112620272, 0.8850453182166284627, 0.9000460863219952312, 0.9150468544273616667, 0.9300476225327284352, 0.9450483906380948707, 0.9496006163947589007 ),
 .UNSPECIFIED. ) 
 CURVE ( )  GEOMETRIC_REPRESENTATION_ITEM ( )  RATIONAL_B_SPLINE_CURVE ( ( 0.9433623850486676510, 0.9066821623815660702, 1.000000000000000000, 0.8660254037844387076, 1.000000000000000000, 0.8660254037844387076, 1.000000000000000000, 0.8660254037844387076, 1.000000000000000000, 0.8660254037844387076, 1.000000000000000000, 0.8660254037844387076, 1.000000000000000000, 0.8660254037844387076, 1.000000000000000000, 0.8660254037844387076, 1.000000000000000000, 0.8660254037844387076, 1.000000000000000000, 0.8660254037844387076, 1.000000000000000000, 0.8660254037844387076, 1.000000000000000000, 0.8660254037844387076, 1.000000000000000000, 0.8660254037844387076, 1.000000000000000000, 0.8660254037844387076, 1.000000000000000000, 0.8660254037844387076, 1.000000000000000000, 0.8660254037844387076, 1.000000000000000000, 0.8660254037844387076, 1.000000000000000000, 0.8660254037844387076, 1.000000000000000000, 0.8660254037844387076, 1.000000000000000000, 0.8660254037844387076, 1.000000000000000000, 0.8660254037844387076, 1.000000000000000000, 0.8660254037844387076, 1.000000000000000000, 0.8660254037844387076, 1.000000000000000000, 0.8660254037844387076, 1.000000000000000000, 0.8660254037844387076, 1.000000000000000000, 0.8660254037844387076, 1.000000000000000000, 0.8660254037844387076, 1.000000000000000000, 0.8660254037844387076, 1.000000000000000000, 0.8660254037844387076, 1.000000000000000000, 0.8660254037844387076, 1.000000000000000000, 0.8660254037844387076, 1.000000000000000000, 0.8660254037844387076, 1.000000000000000000, 0.8660254037844387076, 1.000000000000000000, 0.8660254037844387076, 1.000000000000000000, 0.8660254037844387076, 1.000000000000000000, 0.8660254037844387076, 1.000000000000000000, 0.8660254037844387076, 1.000000000000000000, 0.8660254037844387076, 1.000000000000000000, 0.8660254037844387076, 1.000000000000000000, 0.8660254037844387076, 1.000000000000000000, 0.9593432414028885136, 0.9433623850486800855 ) ) 
 REPRESENTATION_ITEM ( '' )  );
#11428=CARTESIAN_POINT ( 'NONE',  ( 85.40000000000000568, -31.70624999877096784, -101.7320508075688679 ) ) ;
#11432=CARTESIAN_POINT ( 'NONE',  ( 85.15643035625001289, -33.74062499938548854, -99.99999999999998579 ) ) ;
#11433=ADVANCED_FACE ( 'NONE', ( #7070 ), #19000, .F. ) ;
#11440=CARTESIAN_POINT ( 'NONE',  ( -83.20384757729335945, -33.90134618820329848, -96.99999999999998579 ) ) ;
#11444=CARTESIAN_POINT ( 'NONE',  ( 83.90000000000000568, -32.17500000000000426, -102.5980762113533018 ) ) ;
#11445=CYLINDRICAL_SURFACE ( 'NONE', #5518, 3.000000000000002665 ) ;
#11446=B_SPLINE_CURVE_WITH_KNOTS ( 'NONE', 3,
 ( #15989, #8554, #14506, #1140, #19021, #11873, #11970, #4752, #263, #1531, #14801, #3266, #12068, #1428, #8937, #5927 ),
 .UNSPECIFIED., .F., .F.,
 ( 4, 2, 2, 2, 2, 2, 2, 4 ),
 ( 0.000000000000000000, 0.0005391024520904015354, 0.001078204904180803071, 0.002156409808361606142, 0.002695512260452029903, 0.003234614712542453665, 0.003773717164632876993, 0.004312819616723300754 ),
 .UNSPECIFIED. ) ;
#11447=CARTESIAN_POINT ( 'NONE',  ( -83.77821517812500929, -32.42812499938548854, 102.3871387122750889 ) ) ;
#11451=CARTESIAN_POINT ( 'NONE',  ( 79.64356964374998427, -32.12812499938548427, 101.5914258081833879 ) ) ;
#11453=CARTESIAN_POINT ( 'NONE',  ( -85.15643035624999868, -35.11426555956768425, 98.99674139749697588 ) ) ;
#11454=FACE_OUTER_BOUND ( 'NONE', #10177, .T. ) ;
#11463=( BOUNDED_CURVE ( )  B_SPLINE_CURVE ( 2, ( #9654, #18161, #2219, #4784, #3588, #6435, #4876, #6626, #10726 ),
 .UNSPECIFIED., .F., .F. ) 
 B_SPLINE_CURVE_WITH_KNOTS ( ( 3, 2, 2, 2, 3 ),
 ( 0.8541666666666665186, 0.8611111111111111605, 0.8750000000000000000, 0.8888888888888888395, 0.8958333333333333703 ),
 .UNSPECIFIED. ) 
 CURVE ( )  GEOMETRIC_REPRESENTATION_ITEM ( )  RATIONAL_B_SPLINE_CURVE ( ( 0.9330127018922194093, 0.9330127018922177440, 1.000000000000000000, 0.8660254037844387076, 1.000000000000000000, 0.8660254037844387076, 1.000000000000000000, 0.9330127018922187432, 0.9330127018922192983 ) ) 
 REPRESENTATION_ITEM ( '' )  );
#11466=CARTESIAN_POINT ( 'NONE',  ( 82.40000000000001990, -34.55624999877097281, 103.0000000000000000 ) ) ;
#11467=CARTESIAN_POINT ( 'NONE',  ( 81.02178482187500208, -34.94062499938548427, 97.61286128772489690 ) ) ;
#11469=DIRECTION ( 'NONE',  ( -0.000000000000000000, -0.000000000000000000, -1.000000000000000000 ) ) ;
#11472=CARTESIAN_POINT ( 'NONE',  ( -85.15643035625001289, -34.71562499938548285, -98.40857419181659793 ) ) ;
#11473=CARTESIAN_POINT ( 'NONE',  ( 85.15643035624999868, -32.35312499938549280, 98.40857419181659793 ) ) ;
#11474=CARTESIAN_POINT ( 'NONE',  ( 81.02178482187500208, -34.00312499938548427, -97.61286128772489690 ) ) ;
#11476=CARTESIAN_POINT ( 'NONE',  ( -79.64356964374999848, -32.16562499938548569, 99.99999999999998579 ) ) ;
#11477=CARTESIAN_POINT ( 'NONE',  ( 85.15643035624999868, -31.90312499938548285, -101.5914258081833879 ) ) ;
#11478=ORIENTED_EDGE ( 'NONE', *, *, #8247, .T. ) ;
#11479=FACE_OUTER_BOUND ( 'NONE', #5342, .T. ) ;
#11481=PLANE ( 'NONE',  #6185 ) ;
#11483=CARTESIAN_POINT ( 'NONE',  ( -82.39999999999999147, -33.85312499938547859, 96.81714838363319586 ) ) ;
#11484=CARTESIAN_POINT ( 'NONE',  ( -83.77821517812500929, -30.66562499938548569, 97.61286128772489690 ) ) ;
#11488=VECTOR ( 'NONE', #14554, 1000.000000000000000 ) ;
#11490=CARTESIAN_POINT ( 'NONE',  ( 82.41196654184807358, -34.99999999999999289, -97.00083539721711645 ) ) ;
#11494=CARTESIAN_POINT ( 'NONE',  ( -85.40000000000000568, -34.89374999877097139, 99.99999999999998579 ) ) ;
#11495=CARTESIAN_POINT ( 'NONE',  ( -79.39999999999999147, -33.31874999877096855, -99.99999999999998579 ) ) ;
#11497=CARTESIAN_POINT ( 'NONE',  ( -85.40000000000000568, -33.13124999877096855, -101.7320508075688821 ) ) ;
#11499=CARTESIAN_POINT ( 'NONE',  ( 99.99999999999994316, -21.80000000000003268, -139.9999999999999716 ) ) ;
#11500=CARTESIAN_POINT ( 'NONE',  ( 79.64356964375001269, -34.04062499938549280, -98.40857419181659793 ) ) ;
#11502=CARTESIAN_POINT ( 'NONE',  ( -83.90000000000000568, -33.01874999877097139, 102.5980762113533018 ) ) ;
#11505=CARTESIAN_POINT ( 'NONE',  ( 82.39999999999999147, -33.88124999877096855, 96.53589838486223584 ) ) ;
#11511=ORIENTED_EDGE ( 'NONE', *, *, #13311, .T. ) ;
#11512=CARTESIAN_POINT ( 'NONE',  ( -82.39999999999999147, -33.17812499938548854, -96.81714838363319586 ) ) ;
#11514=EDGE_CURVE ( 'NONE', #5649, #8302, #16060, .T. ) ;
#11517=CARTESIAN_POINT ( 'NONE',  ( -83.77821517812500929, -30.32812499938548711, -102.3871387122750889 ) ) ;
#11518=( BOUNDED_CURVE ( )  B_SPLINE_CURVE ( 2, ( #15309, #1922, #6621, #12570, #7885, #13836, #478, #12475, #6429 ),
 .UNSPECIFIED., .F., .F. ) 
 B_SPLINE_CURVE_WITH_KNOTS ( ( 3, 2, 2, 2, 3 ),
 ( 0.8125000000000000000, 0.8194444444444444198, 0.8333333333333333703, 0.8472222222222222099, 0.8541666666666665186 ),
 .UNSPECIFIED. ) 
 CURVE ( )  GEOMETRIC_REPRESENTATION_ITEM ( )  RATIONAL_B_SPLINE_CURVE ( ( 0.9330127018922194093, 0.9330127018922194093, 1.000000000000000000, 0.8660254037844387076, 1.000000000000000000, 0.8660254037844387076, 1.000000000000000000, 0.9330127018922209636, 0.9330127018922194093 ) ) 
 REPRESENTATION_ITEM ( '' )  );
#11519=CARTESIAN_POINT ( 'NONE',  ( 85.39999999999999147, -34.97364041986484295, 101.0919042218176287 ) ) ;
#11520=CARTESIAN_POINT ( 'NONE',  ( -81.70916641599835373, -34.99999999999998579, 97.11314983874014217 ) ) ;
#11523=CARTESIAN_POINT ( 'NONE',  ( -79.64356964374998427, -33.10312499938548569, -98.40857419181659793 ) ) ;
#11526=CARTESIAN_POINT ( 'NONE',  ( 83.90000000000000568, -32.56874999877096855, -102.5980762113533018 ) ) ;
#11528=EDGE_CURVE ( 'NONE', #7316, #13275, #2684, .T. ) ;
#11532=EDGE_CURVE ( 'NONE', #3690, #6638, #2570, .T. ) ;
#11539=VERTEX_POINT ( 'NONE', #12724 ) ;
#11541=CARTESIAN_POINT ( 'NONE',  ( 83.90000000000000568, -31.72500000000000142, -102.5980762113533018 ) ) ;
#11543=CARTESIAN_POINT ( 'NONE',  ( -83.77821517812500929, -30.77812499938548640, 97.61286128772489690 ) ) ;
#11546=DIRECTION ( 'NONE',  ( -0.000000000000000000, -1.000000000000000000, -0.000000000000000000 ) ) ;
#11547=CARTESIAN_POINT ( 'NONE',  ( -82.40000000000001990, -32.75624999877096855, 97.00000000000000000 ) ) ;
#11548=DIRECTION ( 'NONE',  ( -0.000000000000000000, -1.000000000000000000, -0.000000000000000000 ) ) ;
#11551=EDGE_LOOP ( 'NONE', ( #6459, #16410, #397, #7736 ) ) ;
#11552=CARTESIAN_POINT ( 'NONE',  ( -83.77821517812500929, -31.41562499938548569, -97.61286128772489690 ) ) ;
#11557=CARTESIAN_POINT ( 'NONE',  ( 81.59615242270662350, -32.38259618943233420, 102.9999999999999716 ) ) ;
#11558=EDGE_CURVE ( 'NONE', #16799, #4468, #3316, .T. ) ;
#11560=VERTEX_POINT ( 'NONE', #11547 ) ;
#11562=CARTESIAN_POINT ( 'NONE',  ( -82.40000000000000568, -33.93750000000000711, -97.00000000000000000 ) ) ;
#11563=CARTESIAN_POINT ( 'NONE',  ( 79.39999999999999147, -30.18750000000000355, 101.7320508075688821 ) ) ;
#11564=CARTESIAN_POINT ( 'NONE',  ( -82.40000000000000568, -34.38749999999999574, 102.9999999999999858 ) ) ;
#11566=CARTESIAN_POINT ( 'NONE',  ( 99.99999999999997158, -5.200000000000008171, 150.0000000000000000 ) ) ;
#11568=CARTESIAN_POINT ( 'NONE',  ( -81.02178482187500208, -34.00312499938548427, -102.3871387122750889 ) ) ;
#11569=CARTESIAN_POINT ( 'NONE',  ( 81.02178482187500208, -33.44062499938548427, 102.3871387122750889 ) ) ;
#11570=CARTESIAN_POINT ( 'NONE',  ( 85.15643035624999868, -34.79062499938548569, -98.40857419181659793 ) ) ;
#11572=CARTESIAN_POINT ( 'NONE',  ( -82.39999999999999147, -34.07812499938548711, 103.1828516163667899 ) ) ;
#11573=CARTESIAN_POINT ( 'NONE',  ( 85.15643035624999868, -31.07812499938548356, -98.40857419181659793 ) ) ;
#11574=ORIENTED_EDGE ( 'NONE', *, *, #323, .F. ) ;
#11575=CARTESIAN_POINT ( 'NONE',  ( 83.77821517812500929, -34.67812499938548854, 97.61286128772489690 ) ) ;
#11578=CARTESIAN_POINT ( 'NONE',  ( -81.02178482187500208, -33.44062499938548427, 97.61286128772489690 ) ) ;
#11579=CARTESIAN_POINT ( 'NONE',  ( -79.64356964375001269, -31.75312499938548427, 101.5914258081833879 ) ) ;
#11580=ORIENTED_EDGE ( 'NONE', *, *, #10348, .T. ) ;
#11583=CARTESIAN_POINT ( 'NONE',  ( 80.03686793005721256, -35.00000000000000711, -98.35371953419867452 ) ) ;
#11586=CARTESIAN_POINT ( 'NONE',  ( 83.90000000000000568, -33.91874999877096997, -102.5980762113533018 ) ) ;
#11589=CARTESIAN_POINT ( 'NONE',  ( 81.02178482187500208, -33.25312499938548427, 97.61286128772489690 ) ) ;
#11591=CARTESIAN_POINT ( 'NONE',  ( -82.40000000000001990, -32.75624999877096855, -103.0000000000000000 ) ) ;
#11592=CARTESIAN_POINT ( 'NONE',  ( 81.02178482187500208, -34.00312499938548427, -97.61286128772489690 ) ) ;
#11594=ORIENTED_EDGE ( 'NONE', *, *, #12830, .F. ) ;
#11595=CARTESIAN_POINT ( 'NONE',  ( 79.39999999999999147, -33.35624999877097707, 98.26794919243113213 ) ) ;
#11597=CARTESIAN_POINT ( 'NONE',  ( 83.90000000000000568, -32.71874999877096712, 102.5980762113533018 ) ) ;
#11601=CARTESIAN_POINT ( 'NONE',  ( -79.64356964375001269, -34.45312499938548711, -98.40857419181659793 ) ) ;
#11603=EDGE_LOOP ( 'NONE', ( #7963, #5245, #6444, #2156 ) ) ;
#11604=DIRECTION ( 'NONE',  ( 0.000000000000000000, 0.000000000000000000, -1.000000000000000000 ) ) ;
#11605=CARTESIAN_POINT ( 'NONE',  ( -83.77821517812500929, -30.77812499938548640, -102.3871387122750889 ) ) ;
#11606=CARTESIAN_POINT ( 'NONE',  ( -85.40000000000000568, -31.29374999877096997, -99.99999999999998579 ) ) ;
#11607=CARTESIAN_POINT ( 'NONE',  ( 79.39999999999999147, -34.66874999877096997, -99.99999999999998579 ) ) ;
#11612=VECTOR ( 'NONE', #7233, 1000.000000000000000 ) ;
#11614=CARTESIAN_POINT ( 'NONE',  ( 85.40000000000000568, -32.68124999877097281, -98.26794919243111792 ) ) ;
#11617=ADVANCED_FACE ( 'NONE', ( #10082 ), #17125, .T. ) ;
#11618=ORIENTED_EDGE ( 'NONE', *, *, #18431, .T. ) ;
#11628=( BOUNDED_CURVE ( )  B_SPLINE_CURVE ( 2, ( #781, #7807, #16898, #13761, #13852, #2143, #15325, #399, #12490 ),
 .UNSPECIFIED., .F., .F. ) 
 B_SPLINE_CURVE_WITH_KNOTS ( ( 3, 2, 2, 2, 3 ),
 ( 0.6041666666666666297, 0.6111111111111111605, 0.6250000000000000000, 0.6388888888888888395, 0.6458333333333333703 ),
 .UNSPECIFIED. ) 
 CURVE ( )  GEOMETRIC_REPRESENTATION_ITEM ( )  RATIONAL_B_SPLINE_CURVE ( ( 0.9330127018922192983, 0.9330127018922187432, 1.000000000000000000, 0.8660254037844387076, 1.000000000000000000, 0.8660254037844387076, 1.000000000000000000, 0.9330127018922187432, 0.9330127018922192983 ) ) 
 REPRESENTATION_ITEM ( '' )  );
#11633=CARTESIAN_POINT ( 'NONE',  ( 85.40000000000000568, -31.80000000000000071, -99.99999999999998579 ) ) ;
#11634=CARTESIAN_POINT ( 'NONE',  ( 82.39076102795760903, -31.99999999999999289, -102.8695224571928719 ) ) ;
#11635=EDGE_CURVE ( 'NONE', #6898, #10655, #18685, .T. ) ;
#11636=CARTESIAN_POINT ( 'NONE',  ( -79.64356964375001269, -32.24062499938548854, 98.40857419181659793 ) ) ;
#11638=EDGE_CURVE ( 'NONE', #4516, #5783, #14783, .T. ) ;
#11640=EDGE_CURVE ( 'NONE', #5588, #12381, #16789, .T. ) ;
#11642=DIRECTION ( 'NONE',  ( -0.000000000000000000, -0.000000000000000000, -1.000000000000000000 ) ) ;
#11645=ORIENTED_EDGE ( 'NONE', *, *, #11202, .T. ) ;
#11646=SURFACE_STYLE_USAGE ( .BOTH. , #4320 ) ;
#11647=CARTESIAN_POINT ( 'NONE',  ( -79.64356964375001269, -30.85312499938548569, -98.40857419181659793 ) ) ;
#11655=VERTEX_POINT ( 'NONE', #3684 ) ;
#11657=CARTESIAN_POINT ( 'NONE',  ( 79.39999999999999147, -30.63750000000000284, 101.7320508075688821 ) ) ;
#11658=CARTESIAN_POINT ( 'NONE',  ( -69.99999999999998579, -32.00000000000000000, 150.0000000000000000 ) ) ;
#11660=CARTESIAN_POINT ( 'NONE',  ( 82.40000000000000568, -32.30624999877097281, 102.9999999999999858 ) ) ;
#11664=CARTESIAN_POINT ( 'NONE',  ( 81.02178482187500208, -33.59062499938548285, 97.61286128772489690 ) ) ;
#11665=CARTESIAN_POINT ( 'NONE',  ( 79.64356964375001269, -30.77812499938548285, -98.40857419181659793 ) ) ;
#11667=CARTESIAN_POINT ( 'NONE',  ( -81.02178482187500208, -34.34062499938548285, 97.61286128772489690 ) ) ;
#11668=CARTESIAN_POINT ( 'NONE',  ( 82.39999999999999147, -31.60312499938548569, -96.81714838363319586 ) ) ;
#11669=EDGE_LOOP ( 'NONE', ( #3236, #5010, #17084, #17900, #14839, #13874, #3326, #5301, #10473, #16480, #13253, #15367, #17207, #14833, #8198, #3069, #7711 ) ) ;
#11670=CARTESIAN_POINT ( 'NONE',  ( 81.02178482187500208, -34.00312499938548427, 102.3871387122750889 ) ) ;
#11674=CARTESIAN_POINT ( 'NONE',  ( -79.64356964375001269, -34.00312499938549138, 101.5914258081833879 ) ) ;
#11684=CARTESIAN_POINT ( 'NONE',  ( 85.15643035624999868, -32.01562499938548711, 98.40857419181659793 ) ) ;
#11686=CARTESIAN_POINT ( 'NONE',  ( 83.77821517812500929, -32.87812499938548427, -102.3871387122750889 ) ) ;
#11687=CARTESIAN_POINT ( 'NONE',  ( -83.77821517812500929, -32.42812499938548854, -97.61286128772489690 ) ) ;
#11689=CARTESIAN_POINT ( 'NONE',  ( 79.39999999999999147, -33.80624999877097281, 98.26794919243113213 ) ) ;
#11692=CARTESIAN_POINT ( 'NONE',  ( -85.15643035625001289, -30.25312499938548783, 99.99999999999998579 ) ) ;
#11695=CARTESIAN_POINT ( 'NONE',  ( -79.64356964375001269, -34.37812499938548427, -101.5914258081833879 ) ) ;
#11699=CARTESIAN_POINT ( 'NONE',  ( -82.39999999999999147, -30.81562499938548427, -103.1828516163667899 ) ) ;
#11700=CARTESIAN_POINT ( 'NONE',  ( -80.07765479359939320, -32.00000000000000711, -101.8487127466165845 ) ) ;
#11701=CARTESIAN_POINT ( 'NONE',  ( -82.39999999999999147, -31.63124999877097210, -96.53589838486223584 ) ) ;
#11706=CARTESIAN_POINT ( 'NONE',  ( -83.77821517812500929, -34.56562499938548427, -97.61286128772489690 ) ) ;
#11708=AXIS2_PLACEMENT_3D ( 'NONE', #4280, #5942, #17478 ) ;
#11710=CARTESIAN_POINT ( 'NONE',  ( 79.39999999999999147, -32.86874999877097281, -99.99999999999998579 ) ) ;
#11718=EDGE_LOOP ( 'NONE', ( #7322, #11645, #5390, #583 ) ) ;
#11720=VECTOR ( 'NONE', #8842, 1000.000000000000000 ) ;
#11722=CARTESIAN_POINT ( 'NONE',  ( -82.40000000000000568, -32.08124999877097139, 102.9999999999999858 ) ) ;
#11723=ORIENTED_EDGE ( 'NONE', *, *, #19273, .T. ) ;
#11724=CARTESIAN_POINT ( 'NONE',  ( 80.90000000000000568, -32.49374999877097281, -102.5980762113533018 ) ) ;
#11725=CARTESIAN_POINT ( 'NONE',  ( 79.39999999999999147, -34.23750000000000426, -98.26794919243110371 ) ) ;
#11728=CARTESIAN_POINT ( 'NONE',  ( -85.15643035624999868, -33.81562499938549138, 101.5914258081833879 ) ) ;
#11731=CARTESIAN_POINT ( 'NONE',  ( 99.99999999999998579, 0.000000000000000000, -150.0000000000000000 ) ) ;
#11735=AXIS2_PLACEMENT_3D ( 'NONE', #5970, #8985, #16418 ) ;
#11736=CARTESIAN_POINT ( 'NONE',  ( -82.40000000000000568, -34.38749999999999574, -96.99999999999998579 ) ) ;
#11738=DIRECTION ( 'NONE',  ( 1.000000000000000000, 0.000000000000000000, 0.000000000000000000 ) ) ;
#11739=CARTESIAN_POINT ( 'NONE',  ( -83.77821517812500929, -35.12812499938548427, -97.61286128772489690 ) ) ;
#11745=CARTESIAN_POINT ( 'NONE',  ( 81.59615242270665192, -33.28259618943233278, 103.0000000000000000 ) ) ;
#11747=ORIENTED_EDGE ( 'NONE', *, *, #12505, .F. ) ;
#11748=ORIENTED_EDGE ( 'NONE', *, *, #4504, .F. ) ;
#11749=FACE_OUTER_BOUND ( 'NONE', #10352, .T. ) ;
#11752=CARTESIAN_POINT ( 'NONE',  ( -81.59615242270662350, -33.91740381056766296, -96.99999999999997158 ) ) ;
#11753=CARTESIAN_POINT ( 'NONE',  ( 83.77821517812500929, -34.26562499938548711, 102.3871387122750889 ) ) ;
#11757=CARTESIAN_POINT ( 'NONE',  ( -81.59615242270662350, -33.73259618943233562, 96.99999999999998579 ) ) ;
#11758=CARTESIAN_POINT ( 'NONE',  ( 79.64356964375001269, -34.90312499938548285, 98.40857419181659793 ) ) ;
#11759=CARTESIAN_POINT ( 'NONE',  ( 82.39999999999999147, -31.15312499938548640, -96.81714838363319586 ) ) ;
#11761=CARTESIAN_POINT ( 'NONE',  ( 83.77821517812500929, -32.46562499938548285, -97.61286128772489690 ) ) ;
#11764=CARTESIAN_POINT ( 'NONE',  ( 82.39999999999999147, -34.86562499938548854, 103.1828516163667899 ) ) ;
#11767=CARTESIAN_POINT ( 'NONE',  ( -81.02178482187500208, -32.99062499938548854, 97.61286128772489690 ) ) ;
#11769=CARTESIAN_POINT ( 'NONE',  ( -84.75088379146899342, -35.00000000000000711, 101.6079878054202652 ) ) ;
#11774=VECTOR ( 'NONE', #8512, 1000.000000000000000 ) ;
#11781=CARTESIAN_POINT ( 'NONE',  ( 82.39999999999999147, -31.49062499938548854, 96.81714838363319586 ) ) ;
#11785=CARTESIAN_POINT ( 'NONE',  ( -85.15643035625001289, -32.09062499938548996, 98.40857419181659793 ) ) ;
#11786=CARTESIAN_POINT ( 'NONE',  ( -83.77821517812500929, -31.52812499938548996, -97.61286128772489690 ) ) ;
#11788=CARTESIAN_POINT ( 'NONE',  ( 80.90000000000000568, -34.29374999877096997, 97.40192378864668399 ) ) ;
#11793=CARTESIAN_POINT ( 'NONE',  ( -81.02178482187500208, -31.00312499938548783, 102.3871387122750889 ) ) ;
#11794=CARTESIAN_POINT ( 'NONE',  ( 80.07765479365677663, -31.99999999999999289, 101.8487127466820965 ) ) ;
#11795=ORIENTED_EDGE ( 'NONE', *, *, #18843, .T. ) ;
#11796=CARTESIAN_POINT ( 'NONE',  ( -85.15643035624999868, -34.60312499938548569, -98.40857419181659793 ) ) ;
#11802=CARTESIAN_POINT ( 'NONE',  ( -81.02178482187500208, -32.65312499938548996, -102.3871387122750889 ) ) ;
#11803=CARTESIAN_POINT ( 'NONE',  ( -94.79999999999999716, -5.200000000000000178, -150.0000000000000000 ) ) ;
#11804=CARTESIAN_POINT ( 'NONE',  ( -85.40000000000000568, -32.23124999877096997, -101.7320508075688679 ) ) ;
#11809=CARTESIAN_POINT ( 'NONE',  ( -83.90000000000000568, -33.61874999877097281, 97.40192378864668399 ) ) ;
#11812=CARTESIAN_POINT ( 'NONE',  ( 80.90000000000000568, -32.34374999877096712, -97.40192378864668399 ) ) ;
#11814=EDGE_LOOP ( 'NONE', ( #8046, #11011, #2161, #17738, #6352, #3307, #13308, #1873, #1399, #14071, #7969, #15132, #2122, #3930, #3426, #14548, #13182 ) ) ;
#11821=CARTESIAN_POINT ( 'NONE',  ( -82.61711639273519836, -31.99999999999998579, 97.16008101253264329 ) ) ;
#11823=CARTESIAN_POINT ( 'NONE',  ( -83.20384757729335945, -32.28615380933863577, 97.00000000000000000 ) ) ;
#11825=CARTESIAN_POINT ( 'NONE',  ( -80.17984880387896851, -35.00000000000000000, 101.6434491389460959 ) ) ;
#11828=CARTESIAN_POINT ( 'NONE',  ( -82.39999999999999147, -33.51562499938548001, 96.81714838363319586 ) ) ;
#11833=CARTESIAN_POINT ( 'NONE',  ( -81.48596794228828344, -35.00000000000000711, -102.8136019330778339 ) ) ;
#11834=CARTESIAN_POINT ( 'NONE',  ( -83.90000000000000568, -34.57500000000000284, -102.5980762113533018 ) ) ;
#11836=CARTESIAN_POINT ( 'NONE',  ( -85.15643035625001289, -31.04062499938548569, -99.99999999999998579 ) ) ;
#11838=LINE ( 'NONE', #4416, #14878 ) ;
#11839=DIRECTION ( 'NONE',  ( -0.000000000000000000, -0.000000000000000000, -1.000000000000000000 ) ) ;
#11843=ORIENTED_EDGE ( 'NONE', *, *, #8093, .F. ) ;
#11847=CARTESIAN_POINT ( 'NONE',  ( -80.90000000000000568, -31.14374999877097139, 102.5980762113533018 ) ) ;
#11848=CARTESIAN_POINT ( 'NONE',  ( 79.39999999999999147, -32.47500000000000142, 99.99999999999998579 ) ) ;
#11852=CARTESIAN_POINT ( 'NONE',  ( 84.51154815724953551, -35.14114861271051637, 101.7717992799616553 ) ) ;
#11853=( BOUNDED_CURVE ( )  B_SPLINE_CURVE ( 2, ( #8728, #5997, #11949, #19093, #5714, #4242, #15966, #8535, #14484 ),
 .UNSPECIFIED., .F., .F. ) 
 B_SPLINE_CURVE_WITH_KNOTS ( ( 3, 2, 2, 2, 3 ),
 ( 0.4791666666666666297, 0.4861111111111111049, 0.5000000000000000000, 0.5138888888888888395, 0.5208333333333334814 ),
 .UNSPECIFIED. ) 
 CURVE ( )  GEOMETRIC_REPRESENTATION_ITEM ( )  RATIONAL_B_SPLINE_CURVE ( ( 0.9330127018922194093, 0.9330127018922190762, 1.000000000000000000, 0.8660254037844387076, 1.000000000000000000, 0.8660254037844387076, 1.000000000000000000, 0.9330127018922177440, 0.9330127018922194093 ) ) 
 REPRESENTATION_ITEM ( '' )  );
#11854=CARTESIAN_POINT ( 'NONE',  ( 85.15643035624999868, -32.42812499938548854, -98.40857419181659793 ) ) ;
#11856=CARTESIAN_POINT ( 'NONE',  ( 82.40000000000000568, -30.00000000000000355, -99.99999999999998579 ) ) ;
#11857=CARTESIAN_POINT ( 'NONE',  ( 79.64356964375001269, -33.92812499938548854, -98.40857419181659793 ) ) ;
#11860=CARTESIAN_POINT ( 'NONE',  ( 82.40000000000000568, -30.00000000000000355, 99.99999999999998579 ) ) ;
#11863=CARTESIAN_POINT ( 'NONE',  ( -85.40000000000000568, -31.38749999999999574, 98.26794919243111792 ) ) ;
#11864=VERTEX_POINT ( 'NONE', #13140 ) ;
#11865=CARTESIAN_POINT ( 'NONE',  ( -80.90000000000000568, -33.00000000000000000, 102.5980762113533018 ) ) ;
#11869=EDGE_CURVE ( 'NONE', #4397, #3695, #18793, .T. ) ;
#11873=CARTESIAN_POINT ( 'NONE',  ( 85.11512745526613344, -31.99999999999998579, 99.40473233008030718 ) ) ;
#11874=CARTESIAN_POINT ( 'NONE',  ( 83.77821517812500929, -32.12812499938548427, 102.3871387122750889 ) ) ;
#11878=CARTESIAN_POINT ( 'NONE',  ( -85.15643035625001289, -32.91562499938548569, 101.5914258081833879 ) ) ;
#11879=CARTESIAN_POINT ( 'NONE',  ( -82.39999999999999147, -31.71562499938548640, -103.1828516163667899 ) ) ;
#11881=CARTESIAN_POINT ( 'NONE',  ( 85.40000000000000568, -35.36739044046696279, 101.0919052301551204 ) ) ;
#11882=CARTESIAN_POINT ( 'NONE',  ( 82.39999999999999147, -34.33124999877097139, 97.00000000000000000 ) ) ;
#11883=LINE ( 'NONE', #79, #14278 ) ;
#11884=CARTESIAN_POINT ( 'NONE',  ( -85.15643035624999868, -31.64062499938548356, 98.40857419181659793 ) ) ;
#11885=CARTESIAN_POINT ( 'NONE',  ( -85.32499745258149915, -35.00000000000000711, -100.1587029275224978 ) ) ;
#11886=ORIENTED_EDGE ( 'NONE', *, *, #18798, .F. ) ;
#11888=CARTESIAN_POINT ( 'NONE',  ( -82.39999999999999147, -33.62812499938549138, -96.81714838363319586 ) ) ;
#11891=CARTESIAN_POINT ( 'NONE',  ( -85.15643035624999868, -32.54062499938548569, -101.5914258081833879 ) ) ;
#11893=CARTESIAN_POINT ( 'NONE',  ( -82.39999999999999147, -30.95624999877097139, -103.4641016151377499 ) ) ;
#11897=CARTESIAN_POINT ( 'NONE',  ( -79.64356964374999848, -34.41562499938548569, -99.99999999999998579 ) ) ;
#11898=CARTESIAN_POINT ( 'NONE',  ( 79.64356964374998427, -34.00312499938548427, 98.40857419181659793 ) ) ;
#11899=CARTESIAN_POINT ( 'NONE',  ( 81.59615242270662350, -32.38259618943233420, -96.99999999999998579 ) ) ;
#11900=( BOUNDED_CURVE ( )  B_SPLINE_CURVE ( 2, ( #151, #17736, #10490, #4436, #10394, #2966, #16454, #17923, #3063 ),
 .UNSPECIFIED., .F., .F. ) 
 B_SPLINE_CURVE_WITH_KNOTS ( ( 3, 2, 2, 2, 3 ),
 ( 0.6875000000000000000, 0.6944444444444444198, 0.7083333333333333703, 0.7222222222222222099, 0.7291666666666666297 ),
 .UNSPECIFIED. ) 
 CURVE ( )  GEOMETRIC_REPRESENTATION_ITEM ( )  RATIONAL_B_SPLINE_CURVE ( ( 0.9330127018922194093, 0.9330127018922194093, 1.000000000000000000, 0.8660254037844387076, 1.000000000000000000, 0.8660254037844387076, 1.000000000000000000, 0.9330127018922198534, 0.9330127018922192983 ) ) 
 REPRESENTATION_ITEM ( '' )  );
#11902=EDGE_CURVE ( 'NONE', #2874, #6898, #11446, .T. ) ;
#11903=CARTESIAN_POINT ( 'NONE',  ( 82.39999999999999147, -34.78124999877096712, -103.4641016151377499 ) ) ;
#11906=CARTESIAN_POINT ( 'NONE',  ( 85.15643035625001289, -34.60312499938548569, -101.5914258081833879 ) ) ;
#11912=EDGE_LOOP ( 'NONE', ( #4768, #12001, #13449, #11171 ) ) ;
#11915=CARTESIAN_POINT ( 'NONE',  ( -82.40000000000000568, -30.00000000000000355, -96.99999999999998579 ) ) ;
#11918=CARTESIAN_POINT ( 'NONE',  ( 82.40000000000000568, -31.99999999999999289, -99.99999999999998579 ) ) ;
#11921=CARTESIAN_POINT ( 'NONE',  ( -79.64356964375001269, -35.01562499938548711, 101.5914258081833879 ) ) ;
#11925=DIRECTION ( 'NONE',  ( 0.000000000000000000, 0.000000000000000000, 1.000000000000000000 ) ) ;
#11926=CARTESIAN_POINT ( 'NONE',  ( -82.40000000000001990, -33.26250000000000284, -103.0000000000000000 ) ) ;
#11927=CARTESIAN_POINT ( 'NONE',  ( -80.48808202378404530, -35.00000000000000000, -102.1951992292040075 ) ) ;
#11930=CARTESIAN_POINT ( 'NONE',  ( -83.77821517812500929, -34.26562499938548711, -102.3871387122750889 ) ) ;
#11932=AXIS2_PLACEMENT_3D ( 'NONE', #14252, #2338, #8209 ) ;
#11939=ORIENTED_EDGE ( 'NONE', *, *, #13637, .T. ) ;
#11941=CARTESIAN_POINT ( 'NONE',  ( -85.14613134194615895, -32.00000000000000000, 99.70214005991836359 ) ) ;
#11943=CARTESIAN_POINT ( 'NONE',  ( -82.39999999999999147, -32.75624999877096855, 96.53589838486223584 ) ) ;
#11944=CARTESIAN_POINT ( 'NONE',  ( 80.90000000000000568, -31.94999999999999929, 102.5980762113533018 ) ) ;
#11945=CARTESIAN_POINT ( 'NONE',  ( -84.12306224665893239, -32.00000000000001421, -97.80849716182723341 ) ) ;
#11946=AXIS2_PLACEMENT_3D ( 'NONE', #7733, #1969, #6374 ) ;
#11949=CARTESIAN_POINT ( 'NONE',  ( 83.90000000000000568, -33.01874999877097139, -102.5980762113533018 ) ) ;
#11950=CARTESIAN_POINT ( 'NONE',  ( 81.02178482187500208, -32.09062499938548285, -97.61286128772489690 ) ) ;
#11951=EDGE_LOOP ( 'NONE', ( #10208, #4820 ) ) ;
#11954=CARTESIAN_POINT ( 'NONE',  ( 82.39999999999999147, -34.30312499938548143, -96.81714838363319586 ) ) ;
#11955=CYLINDRICAL_SURFACE ( 'NONE', #423, 5.199999999999996625 ) ;
#11956=CARTESIAN_POINT ( 'NONE',  ( -82.39999999999999147, -33.20624999877097849, 97.00000000000000000 ) ) ;
#11958=CARTESIAN_POINT ( 'NONE',  ( -82.39999999999999147, -30.78750000000000497, 103.4641016151377499 ) ) ;
#11960=CARTESIAN_POINT ( 'NONE',  ( 82.40000000000000568, -33.43124999877096570, -102.9999999999999858 ) ) ;
#11964=EDGE_CURVE ( 'NONE', #16006, #16850, #17309, .T. ) ;
#11965=( BOUNDED_CURVE ( )  B_SPLINE_CURVE ( 2, ( #6531, #10915, #9252, #9445, #9348, #293, #480, #18255, #12477 ),
 .UNSPECIFIED., .F., .F. ) 
 B_SPLINE_CURVE_WITH_KNOTS ( ( 3, 2, 2, 2, 3 ),
 ( 0.7708333333333332593, 0.7777777777777777901, 0.7916666666666666297, 0.8055555555555555802, 0.8125000000000000000 ),
 .UNSPECIFIED. ) 
 CURVE ( )  GEOMETRIC_REPRESENTATION_ITEM ( )  RATIONAL_B_SPLINE_CURVE ( ( 0.9330127018922192983, 0.9330127018922187432, 1.000000000000000000, 0.8660254037844387076, 1.000000000000000000, 0.8660254037844387076, 1.000000000000000000, 0.9330127018922194093, 0.9330127018922194093 ) ) 
 REPRESENTATION_ITEM ( '' )  );
#11967=LINE ( 'NONE', #8934, #14841 ) ;
#11968=CARTESIAN_POINT ( 'NONE',  ( -80.90000000000000568, -32.04374999877096997, 102.5980762113533018 ) ) ;
#11970=CARTESIAN_POINT ( 'NONE',  ( 85.16931825408417467, -32.00000000000000000, 99.76128878215590134 ) ) ;
#11971=CARTESIAN_POINT ( 'NONE',  ( 83.77821517812500929, -33.02812499938548285, 102.3871387122750889 ) ) ;
#11972=DIRECTION ( 'NONE',  ( 0.000000000000000000, -1.000000000000000000, 0.000000000000000000 ) ) ;
#11973=CARTESIAN_POINT ( 'NONE',  ( -81.59615242270662350, -32.38259618943233420, -102.9999999999999716 ) ) ;
#11974=CARTESIAN_POINT ( 'NONE',  ( 79.64356964375001269, -35.01562499938548711, -101.5914258081833879 ) ) ;
#11975=CARTESIAN_POINT ( 'NONE',  ( -81.02178482187500208, -31.00312499938548783, -97.61286128772489690 ) ) ;
#11977=CARTESIAN_POINT ( 'NONE',  ( 85.15643035624999868, -30.66562499938548569, 98.40857419181659793 ) ) ;
#11983=CARTESIAN_POINT ( 'NONE',  ( -82.39999999999999147, -31.26562499938549067, 96.81714838363319586 ) ) ;
#11987=CARTESIAN_POINT ( 'NONE',  ( -80.90000000000000568, -31.65000000000000568, -97.40192378864668399 ) ) ;
#11988=DIRECTION ( 'NONE',  ( 1.000000000000000000, 0.000000000000000000, 0.000000000000000000 ) ) ;
#11990=CARTESIAN_POINT ( 'NONE',  ( -83.77821517812500929, -32.87812499938548427, -97.61286128772489690 ) ) ;
#11991=CARTESIAN_POINT ( 'NONE',  ( -80.80006050676047380, -32.00000000000000000, -102.4537706361438438 ) ) ;
#11996=CARTESIAN_POINT ( 'NONE',  ( 85.15643035625001289, -32.35312499938548569, 98.40857419181659793 ) ) ;
#11998=FACE_OUTER_BOUND ( 'NONE', #4033, .T. ) ;
#11999=CARTESIAN_POINT ( 'NONE',  ( 85.40000000000000568, -33.54374999877096286, -99.99999999999998579 ) ) ;
#12001=ORIENTED_EDGE ( 'NONE', *, *, #17238, .F. ) ;
#12008=ORIENTED_EDGE ( 'NONE', *, *, #18216, .F. ) ;
#12010=DIRECTION ( 'NONE',  ( 0.000000000000000000, 0.000000000000000000, -1.000000000000000000 ) ) ;
#12011=CARTESIAN_POINT ( 'NONE',  ( -85.40000000000000568, -33.56250000000000000, -98.26794919243111792 ) ) ;
#12013=DIRECTION ( 'NONE',  ( 0.000000000000000000, -1.000000000000000000, 0.000000000000000000 ) ) ;
#12015=CARTESIAN_POINT ( 'NONE',  ( -85.15643035624999868, -34.34062499938548285, 98.40857419181659793 ) ) ;
#12020=EDGE_CURVE ( 'NONE', #10773, #15647, #13598, .T. ) ;
#12022=LINE ( 'NONE', #4807, #16498 ) ;
#12023=LINE ( 'NONE', #7437, #4939 ) ;
#12027=CARTESIAN_POINT ( 'NONE',  ( -83.77821517812500929, -32.31562499938548427, -97.61286128772489690 ) ) ;
#12031=CARTESIAN_POINT ( 'NONE',  ( 69.99999999999998579, -34.99999999999999289, 150.0000000000000000 ) ) ;
#12033=CARTESIAN_POINT ( 'NONE',  ( 82.39999999999999147, -33.48750000000000426, 97.00000000000000000 ) ) ;
#12039=CARTESIAN_POINT ( 'NONE',  ( -80.90000000000000568, -32.34374999877096712, 97.40192378864668399 ) ) ;
#12040=CARTESIAN_POINT ( 'NONE',  ( 85.40000000000000568, -31.38749999999999574, 101.7320508075688679 ) ) ;
#12044=CARTESIAN_POINT ( 'NONE',  ( 83.90000000000000568, -32.26874999877097139, 102.5980762113533018 ) ) ;
#12045=CARTESIAN_POINT ( 'NONE',  ( 80.24181665639378025, -32.00000000000000000, -97.97695283462226712 ) ) ;
#12047=CARTESIAN_POINT ( 'NONE',  ( 82.39999999999999147, -31.82812499938548356, -103.1828516163667899 ) ) ;
#12050=DIRECTION ( 'NONE',  ( 0.000000000000000000, 1.000000000000000000, 0.000000000000000000 ) ) ;
#12051=CARTESIAN_POINT ( 'NONE',  ( 79.64356964374999848, -34.41562499938548569, -99.99999999999998579 ) ) ;
#12053=FACE_OUTER_BOUND ( 'NONE', #1464, .T. ) ;
#12055=AXIS2_PLACEMENT_3D ( 'NONE', #10621, #14627, #1262 ) ;
#12056=CARTESIAN_POINT ( 'NONE',  ( -79.39999999999999147, -31.57499999999999929, 99.99999999999998579 ) ) ;
#12062=CARTESIAN_POINT ( 'NONE',  ( 85.15643035625001289, -30.14062499938548711, 99.99999999999998579 ) ) ;
#12065=DIRECTION ( 'NONE',  ( 9.251858538542962756E-15, 0.000000000000000000, -1.000000000000000000 ) ) ;
#12066=CARTESIAN_POINT ( 'NONE',  ( -83.90000000000000568, -32.32500000000000284, 97.40192378864668399 ) ) ;
#12068=CARTESIAN_POINT ( 'NONE',  ( 84.74067385206578251, -31.99999999999998579, 101.4666071953140829 ) ) ;
#12069=CARTESIAN_POINT ( 'NONE',  ( 85.15643035624999868, -30.55312499938548854, 98.40857419181659793 ) ) ;
#12070=CARTESIAN_POINT ( 'NONE',  ( -82.40000000000001990, -32.08124999877097139, 103.0000000000000000 ) ) ;
#12071=DIRECTION ( 'NONE',  ( 1.000000000000000000, 0.000000000000000000, 0.000000000000000000 ) ) ;
#12072=CARTESIAN_POINT ( 'NONE',  ( 85.15643035624999868, -35.16562499938547859, -101.5914258081833879 ) ) ;
#12074=VERTEX_POINT ( 'NONE', #14105 ) ;
#12075=CARTESIAN_POINT ( 'NONE',  ( 83.77821517812500929, -31.22812499938548569, 102.3871387122750889 ) ) ;
#12078=CARTESIAN_POINT ( 'NONE',  ( -83.77821517812500929, -30.62812499938548783, 102.3871387122750889 ) ) ;
#12079=CARTESIAN_POINT ( 'NONE',  ( 80.90000000000000568, -33.84374999877096712, -102.5980762113533018 ) ) ;
#12081=CARTESIAN_POINT ( 'NONE',  ( -85.40000000000000568, -30.45000000000000284, -99.99999999999998579 ) ) ;
#12084=CARTESIAN_POINT ( 'NONE',  ( 85.40000000000000568, -34.05000000000000426, -99.99999999999998579 ) ) ;
#12085=CARTESIAN_POINT ( 'NONE',  ( 85.40000000000000568, -34.93124999877096570, -98.26794919243111792 ) ) ;
#12086=CARTESIAN_POINT ( 'NONE',  ( -85.15643035624999868, -32.46562499938548996, -98.40857419181659793 ) ) ;
#12092=CARTESIAN_POINT ( 'NONE',  ( -83.20395887649183919, -35.00000000000001421, -97.36341917746362640 ) ) ;
#12093=CARTESIAN_POINT ( 'NONE',  ( 85.15643035625001289, -32.84062499938548285, 99.99999999999998579 ) ) ;
#12096=CARTESIAN_POINT ( 'NONE',  ( 79.39999999999999147, -34.21874999877096712, -99.99999999999998579 ) ) ;
#12104=EDGE_CURVE ( 'NONE', #5530, #2874, #8191, .T. ) ;
#12112=ORIENTED_EDGE ( 'NONE', *, *, #3769, .T. ) ;
#12115=AXIS2_PLACEMENT_3D ( 'NONE', #13485, #16526, #13774 ) ;
#12117=CARTESIAN_POINT ( 'NONE',  ( -79.64356964374999848, -34.52812499938548285, 99.99999999999998579 ) ) ;
#12123=CARTESIAN_POINT ( 'NONE',  ( -79.39999999999999147, -33.82500000000000284, 99.99999999999998579 ) ) ;
#12125=CARTESIAN_POINT ( 'NONE',  ( -82.40000000000000568, -34.78124999877096712, -96.99999999999998579 ) ) ;
#12126=EDGE_CURVE ( 'NONE', #4990, #14525, #11426, .T. ) ;
#12130=CARTESIAN_POINT ( 'NONE',  ( -82.39999999999999147, -32.50312499938548427, -103.1828516163667899 ) ) ;
#12132=FACE_OUTER_BOUND ( 'NONE', #16552, .T. ) ;
#12141=CARTESIAN_POINT ( 'NONE',  ( -82.39999999999999147, -32.53124999877096712, 103.4641016151377499 ) ) ;
#12142=CARTESIAN_POINT ( 'NONE',  ( 83.90000000000000568, -31.87500000000000000, 102.5980762113533018 ) ) ;
#12143=CARTESIAN_POINT ( 'NONE',  ( 83.90000000000000568, -33.46874999877096712, 97.40192378864668399 ) ) ;
#12146=CARTESIAN_POINT ( 'NONE',  ( 82.39999999999999147, -33.29062499938548569, -103.1828516163667899 ) ) ;
#12147=CARTESIAN_POINT ( 'NONE',  ( 80.07765479359947847, -32.00000000000000000, -98.15128725338327342 ) ) ;
#12148=CARTESIAN_POINT ( 'NONE',  ( 79.64356964375001269, -34.90312499938548285, -101.5914258081833879 ) ) ;
#12153=CARTESIAN_POINT ( 'NONE',  ( 81.02178482187500208, -33.89062499938548711, -97.61286128772489690 ) ) ;
#12157=CARTESIAN_POINT ( 'NONE',  ( -80.90000000000000568, -30.15000000000000213, 97.40192378864668399 ) ) ;
#12166=CARTESIAN_POINT ( 'NONE',  ( 85.15643035624999868, -34.34062499938548285, 101.5914258081833879 ) ) ;
#12167=DIRECTION ( 'NONE',  ( 0.000000000000000000, -1.000000000000000000, 0.000000000000000000 ) ) ;
#12169=CARTESIAN_POINT ( 'NONE',  ( -79.64356964374999848, -32.27812499938548996, 99.99999999999998579 ) ) ;
#12170=CARTESIAN_POINT ( 'NONE',  ( -85.15643035625001289, -33.85312499938549280, -99.99999999999998579 ) ) ;
#12172=ORIENTED_EDGE ( 'NONE', *, *, #14147, .F. ) ;
#12173=CARTESIAN_POINT ( 'NONE',  ( 82.39999999999999147, -34.78124999877096712, 96.53589838486223584 ) ) ;
#12174=CARTESIAN_POINT ( 'NONE',  ( 82.40000000000000568, -34.78124999877096712, -102.9999999999999858 ) ) ;
#12176=CARTESIAN_POINT ( 'NONE',  ( -79.64356964375001269, -31.34062499938548640, 98.40857419181659793 ) ) ;
#12178=ORIENTED_EDGE ( 'NONE', *, *, #6300, .F. ) ;
#12179=CARTESIAN_POINT ( 'NONE',  ( -85.40000000000000568, -30.41249999999999787, -98.26794919243111792 ) ) ;
#12180=CARTESIAN_POINT ( 'NONE',  ( 84.57144699476174310, -35.00000000000000000, 102.0792695867486657 ) ) ;
#12182=CARTESIAN_POINT ( 'NONE',  ( -82.39999999999999147, -33.06562499938548427, -103.1828516163667899 ) ) ;
#12188=CARTESIAN_POINT ( 'NONE',  ( 81.02178482187500208, -32.69062499938548427, 97.61286128772489690 ) ) ;
#12190=DIRECTION ( 'NONE',  ( 0.000000000000000000, -1.000000000000000000, 0.000000000000000000 ) ) ;
#12191=CARTESIAN_POINT ( 'NONE',  ( 79.39999999999999147, -33.73124999877096997, -98.26794919243110371 ) ) ;
#12202=CARTESIAN_POINT ( 'NONE',  ( -79.64356964375001269, -30.32812499938548711, -101.5914258081833879 ) ) ;
#12207=CARTESIAN_POINT ( 'NONE',  ( -82.39999999999999147, -34.83749999999999858, 103.0000000000000000 ) ) ;
#12208=ADVANCED_FACE ( 'NONE', ( #6867 ), #18588, .F. ) ;
#12216=CARTESIAN_POINT ( 'NONE',  ( 81.59615242270665192, -34.81740381056767575, -103.0000000000000000 ) ) ;
#12220=CARTESIAN_POINT ( 'NONE',  ( -82.39999999999999147, -33.40312499938548285, -103.1828516163667899 ) ) ;
#12223=FACE_BOUND ( 'NONE', #15279, .T. ) ;
#12224=CARTESIAN_POINT ( 'NONE',  ( 83.20395887649171129, -35.00000000000000711, -102.6365808225363878 ) ) ;
#12226=FACE_OUTER_BOUND ( 'NONE', #10639, .T. ) ;
#12229=VERTEX_POINT ( 'NONE', #16833 ) ;
#12230=ADVANCED_FACE ( 'NONE', ( #3818 ), #15557, .F. ) ;
#12232=CARTESIAN_POINT ( 'NONE',  ( -80.24533121543032621, -32.00000000000001421, 102.0417045141624044 ) ) ;
#12233=CARTESIAN_POINT ( 'NONE',  ( 80.90000000000000568, -31.05000000000000071, -97.40192378864668399 ) ) ;
#12234=EDGE_CURVE ( 'NONE', #10401, #2299, #7931, .T. ) ;
#12236=CARTESIAN_POINT ( 'NONE',  ( -80.90000000000000568, -31.59374999877097423, 102.5980762113533018 ) ) ;
#12237=CARTESIAN_POINT ( 'NONE',  ( 85.40000000000000568, -31.31250000000000000, 98.26794919243111792 ) ) ;
#12238=CARTESIAN_POINT ( 'NONE',  ( -84.44763168836720979, -32.00000000000001421, -98.15470523285542015 ) ) ;
#12240=CARTESIAN_POINT ( 'NONE',  ( 82.39999999999999147, -34.19062499938548427, -103.1828516163667899 ) ) ;
#12244=CARTESIAN_POINT ( 'NONE',  ( 85.15643035625001289, -33.74062499938548854, -99.99999999999998579 ) ) ;
#12245=ORIENTED_EDGE ( 'NONE', *, *, #18668, .T. ) ;
#12247=CARTESIAN_POINT ( 'NONE',  ( 85.15643035625001289, -32.39062499938548711, -99.99999999999998579 ) ) ;
#12248=CARTESIAN_POINT ( 'NONE',  ( -83.33080762004576059, -35.05289549976084373, 96.44210921874548603 ) ) ;
#12249=DIRECTION ( 'NONE',  ( -0.000000000000000000, 1.000000000000000000, 0.000000000000000000 ) ) ;
#12252=CARTESIAN_POINT ( 'NONE',  ( -85.40000000000000568, -30.93750000000000355, 98.26794919243111792 ) ) ;
#12257=AXIS2_PLACEMENT_3D ( 'NONE', #4439, #12249, #10397 ) ;
#12258=CARTESIAN_POINT ( 'NONE',  ( -82.40000000000001990, -34.16250000000000853, 97.00000000000000000 ) ) ;
#12260=CARTESIAN_POINT ( 'NONE',  ( 82.39999999999999147, -30.70312499938548711, 103.1828516163667899 ) ) ;
#12265=CARTESIAN_POINT ( 'NONE',  ( 79.64356964375001269, -30.85312499938548569, 98.40857419181659793 ) ) ;
#12266=CARTESIAN_POINT ( 'NONE',  ( 79.64356964375001269, -32.69062499938548427, -98.40857419181659793 ) ) ;
#12267=ADVANCED_FACE ( 'NONE', ( #16925 ), #15653, .F. ) ;
#12269=CARTESIAN_POINT ( 'NONE',  ( -81.02178482187500208, -34.15312499938548285, 102.3871387122750889 ) ) ;
#12270=CARTESIAN_POINT ( 'NONE',  ( -81.02178482187500208, -33.10312499938548569, -102.3871387122750889 ) ) ;
#12272=ORIENTED_EDGE ( 'NONE', *, *, #5306, .F. ) ;
#12273=CARTESIAN_POINT ( 'NONE',  ( 85.15643035625001289, -30.25312499938548783, 99.99999999999998579 ) ) ;
#12276=CARTESIAN_POINT ( 'NONE',  ( -79.64356964375001269, -34.94062499938549138, 98.40857419181659793 ) ) ;
#12279=CARTESIAN_POINT ( 'NONE',  ( -82.39999999999999147, -31.23750000000000071, -96.53589838486223584 ) ) ;
#12280=CARTESIAN_POINT ( 'NONE',  ( 83.90000000000000568, -34.57500000000000284, -97.40192378864668399 ) ) ;
#12282=CARTESIAN_POINT ( 'NONE',  ( -81.02178482187500208, -35.05312499938548854, -97.61286128772489690 ) ) ;
#12286=ORIENTED_EDGE ( 'NONE', *, *, #10564, .T. ) ;
#12288=CARTESIAN_POINT ( 'NONE',  ( 80.90000000000000568, -32.79374999877096997, -97.40192378864668399 ) ) ;
#12289=CARTESIAN_POINT ( 'NONE',  ( 81.02178482187500208, -32.24062499938548854, 97.61286128772489690 ) ) ;
#12291=CARTESIAN_POINT ( 'NONE',  ( -85.40000000000000568, -34.40624999877096712, 101.7320508075688821 ) ) ;
#12292=CARTESIAN_POINT ( 'NONE',  ( 80.90000000000000568, -34.74374999877097281, -102.5980762113533018 ) ) ;
#12294=ORIENTED_EDGE ( 'NONE', *, *, #6502, .T. ) ;
#12300=VERTEX_POINT ( 'NONE', #2636 ) ;
#12303=CARTESIAN_POINT ( 'NONE',  ( -83.90000000000000568, -32.32500000000000284, -102.5980762113533018 ) ) ;
#12307=CARTESIAN_POINT ( 'NONE',  ( -79.39999999999999147, -33.35624999877097707, -98.26794919243113213 ) ) ;
#12312=CARTESIAN_POINT ( 'NONE',  ( 80.90000000000000568, -34.14374999877097139, -97.40192378864668399 ) ) ;
#12319=CARTESIAN_POINT ( 'NONE',  ( -79.64356964375001269, -34.00312499938549138, -98.40857419181659793 ) ) ;
#12327=EDGE_CURVE ( 'NONE', #9376, #12074, #7146, .T. ) ;
#12329=EDGE_LOOP ( 'NONE', ( #18751, #2248, #15626, #13647 ) ) ;
#12330=CARTESIAN_POINT ( 'NONE',  ( 80.90000000000000568, -33.39374999877097139, -102.5980762113533018 ) ) ;
#12331=CARTESIAN_POINT ( 'NONE',  ( 83.88339518848731302, -35.16733441503058089, -97.47959136244114120 ) ) ;
#12332=CARTESIAN_POINT ( 'NONE',  ( -82.39999999999999147, -34.78124999877096712, 103.4641016151377499 ) ) ;
#12333=CARTESIAN_POINT ( 'NONE',  ( -82.40000000000001990, -34.16250000000000853, -103.0000000000000000 ) ) ;
#12335=CARTESIAN_POINT ( 'NONE',  ( 82.39999999999999147, -32.16562499938548569, -96.81714838363319586 ) ) ;
#12337=DIRECTION ( 'NONE',  ( 1.000000000000000000, -1.156482317317870344E-15, 0.000000000000000000 ) ) ;
#12338=CARTESIAN_POINT ( 'NONE',  ( -79.64356964375001269, -33.02812499938548285, 98.40857419181659793 ) ) ;
#12339=VECTOR ( 'NONE', #7522, 1000.000000000000000 ) ;
#12341=CARTESIAN_POINT ( 'NONE',  ( 79.64356964375001269, -33.92812499938548854, -98.40857419181659793 ) ) ;
#12344=CARTESIAN_POINT ( 'NONE',  ( -94.79999999999999716, -32.00000000000000000, 150.0000000000000000 ) ) ;
#12345=CARTESIAN_POINT ( 'NONE',  ( 94.79999999999995453, -29.80000000000000071, 150.0000000000000000 ) ) ;
#12349=CARTESIAN_POINT ( 'NONE',  ( -83.90000000000000568, -31.87500000000000000, 97.40192378864668399 ) ) ;
#12350=ADVANCED_FACE ( 'NONE', ( #9983 ), #11445, .F. ) ;
#12351=EDGE_LOOP ( 'NONE', ( #2786, #4173, #13256, #11417 ) ) ;
#12353=VECTOR ( 'NONE', #6330, 1000.000000000000000 ) ;
#12357=CARTESIAN_POINT ( 'NONE',  ( -79.64356964374999848, -32.27812499938548996, -99.99999999999998579 ) ) ;
#12358=CARTESIAN_POINT ( 'NONE',  ( 81.02178482187500208, -34.00312499938548427, 102.3871387122750889 ) ) ;
#12360=EDGE_CURVE ( 'NONE', #2207, #3690, #3513, .T. ) ;
#12361=CARTESIAN_POINT ( 'NONE',  ( 83.77821517812500929, -32.42812499938548854, -102.3871387122750889 ) ) ;
#12363=CARTESIAN_POINT ( 'NONE',  ( -83.77821517812500929, -34.37812499938548427, 97.61286128772489690 ) ) ;
#12364=CARTESIAN_POINT ( 'NONE',  ( -83.77821517812500929, -32.87812499938548427, -97.61286128772489690 ) ) ;
#12367=CARTESIAN_POINT ( 'NONE',  ( 85.15643035624999868, -31.64062499938548356, 101.5914258081833879 ) ) ;
#12370=CARTESIAN_POINT ( 'NONE',  ( -85.15643035624999868, -33.44062499938548427, 98.40857419181659793 ) ) ;
#12373=CARTESIAN_POINT ( 'NONE',  ( -79.39999999999999147, -31.16250000000000497, -98.26794919243113213 ) ) ;
#12374=CARTESIAN_POINT ( 'NONE',  ( 84.42750213138106119, -35.00000000000000000, 102.2200415044236905 ) ) ;
#12377=DIRECTION ( 'NONE',  ( -0.000000000000000000, -1.000000000000000000, -0.000000000000000000 ) ) ;
#12381=VERTEX_POINT ( 'NONE', #17504 ) ;
#12383=CARTESIAN_POINT ( 'NONE',  ( -83.90000000000000568, -33.22500000000000142, 97.40192378864668399 ) ) ;
#12384=CARTESIAN_POINT ( 'NONE',  ( -94.79999999999999716, -5.200000000000000178, 150.0000000000000000 ) ) ;
#12386=CARTESIAN_POINT ( 'NONE',  ( 79.64356964374999848, -30.92812499938548498, -99.99999999999998579 ) ) ;
#12388=ORIENTED_EDGE ( 'NONE', *, *, #14122, .F. ) ;
#12392=VECTOR ( 'NONE', #2128, 1000.000000000000000 ) ;
#12399=CARTESIAN_POINT ( 'NONE',  ( -82.40000000000000568, -33.71249999999998437, -102.9999999999999858 ) ) ;
#12403=CARTESIAN_POINT ( 'NONE',  ( -79.39999999999999147, -34.70624999877097139, -98.26794919243113213 ) ) ;
#12409=FACE_OUTER_BOUND ( 'NONE', #7117, .T. ) ;
#12410=FACE_OUTER_BOUND ( 'NONE', #5963, .T. ) ;
#12417=CARTESIAN_POINT ( 'NONE',  ( -82.39999999999999147, -33.48750000000000426, -97.00000000000000000 ) ) ;
#12423=VECTOR ( 'NONE', #18252, 1000.000000000000000 ) ;
#12424=ORIENTED_EDGE ( 'NONE', *, *, #13900, .F. ) ;
#12427=CARTESIAN_POINT ( 'NONE',  ( 79.39999999999999147, -31.53750000000000497, -98.26794919243110371 ) ) ;
#12428=DIRECTION ( 'NONE',  ( 0.000000000000000000, 0.000000000000000000, -1.000000000000000000 ) ) ;
#12429=CARTESIAN_POINT ( 'NONE',  ( -80.90000000000000568, -33.84374999877096712, 102.5980762113533018 ) ) ;
#12431=CARTESIAN_POINT ( 'NONE',  ( 85.40000000000000568, -32.21250000000000568, -101.7320508075688821 ) ) ;
#12432=CARTESIAN_POINT ( 'NONE',  ( 79.64356964374999848, -34.07812499938548711, -99.99999999999998579 ) ) ;
#12433=CARTESIAN_POINT ( 'NONE',  ( 80.90000000000000568, -33.30000000000000426, -97.40192378864668399 ) ) ;
#12434=CARTESIAN_POINT ( 'NONE',  ( -81.02178482187500208, -32.99062499938548854, 97.61286128772489690 ) ) ;
#12435=CARTESIAN_POINT ( 'NONE',  ( 83.77821517812500929, -32.76562499938548711, -102.3871387122750889 ) ) ;
#12438=CARTESIAN_POINT ( 'NONE',  ( -80.90000000000000568, -34.64999999999999858, 97.40192378864668399 ) ) ;
#12439=CARTESIAN_POINT ( 'NONE',  ( 82.40000000000001990, -32.13750000000000284, 97.00000000000000000 ) ) ;
#12443=CARTESIAN_POINT ( 'NONE',  ( -82.39999999999999147, -31.68750000000000355, 103.4641016151377499 ) ) ;
#12446=CARTESIAN_POINT ( 'NONE',  ( 96.99999999999994316, -29.80000000000000426, -150.0000000000000000 ) ) ;
#12447=CARTESIAN_POINT ( 'NONE',  ( 79.64356964375001269, -33.02812499938548285, 101.5914258081833879 ) ) ;
#12449=CARTESIAN_POINT ( 'NONE',  ( 84.56803305035325025, -32.00000000000000000, -101.7116913729796863 ) ) ;
#12451=CARTESIAN_POINT ( 'NONE',  ( -85.15643035625001289, -32.50312499938548427, -99.99999999999998579 ) ) ;
#12452=CARTESIAN_POINT ( 'NONE',  ( 85.15643035624999868, -30.17812499938548498, 101.5914258081833879 ) ) ;
#12454=CARTESIAN_POINT ( 'NONE',  ( 81.02178482187500208, -30.55312499938548854, -102.3871387122750889 ) ) ;
#12456=CARTESIAN_POINT ( 'NONE',  ( -83.77821517812500929, -34.82812499938548711, 97.61286128772489690 ) ) ;
#12457=CARTESIAN_POINT ( 'NONE',  ( -83.77821517812500929, -34.37812499938548427, -102.3871387122750889 ) ) ;
#12459=CARTESIAN_POINT ( 'NONE',  ( 82.39999999999999147, -31.94062499938548427, 96.81714838363319586 ) ) ;
#12460=CARTESIAN_POINT ( 'NONE',  ( -81.02178482187500208, -34.45312499938548711, 97.61286128772489690 ) ) ;
#12461=CARTESIAN_POINT ( 'NONE',  ( 82.39999999999999147, -32.98124999877096286, 96.99999999999998579 ) ) ;
#12463=CARTESIAN_POINT ( 'NONE',  ( -80.90000000000000568, -32.85000000000000142, -102.5980762113533018 ) ) ;
#12467=CARTESIAN_POINT ( 'NONE',  ( 94.79999999999991189, -3.000000000000000000, -150.0000000000000000 ) ) ;
#12469=CARTESIAN_POINT ( 'NONE',  ( -82.40000000000000568, -30.00000000000000355, 99.99999999999998579 ) ) ;
#12473=ORIENTED_EDGE ( 'NONE', *, *, #4755, .F. ) ;
#12475=CARTESIAN_POINT ( 'NONE',  ( 83.20384757729338787, -34.59240381056766722, -97.00000000000000000 ) ) ;
#12477=CARTESIAN_POINT ( 'NONE',  ( 82.40000000000000568, -34.38749999999999574, 96.99999999999998579 ) ) ;
#12479=CARTESIAN_POINT ( 'NONE',  ( 85.15643035624999868, -30.74062499938548143, -98.40857419181659793 ) ) ;
#12482=CARTESIAN_POINT ( 'NONE',  ( 83.90000000000000568, -30.91874999877096997, 102.5980762113533018 ) ) ;
#12487=ORIENTED_EDGE ( 'NONE', *, *, #10001, .F. ) ;
#12489=CARTESIAN_POINT ( 'NONE',  ( -85.15643035624999868, -31.90312499938548285, -98.40857419181659793 ) ) ;
#12490=CARTESIAN_POINT ( 'NONE',  ( -82.40000000000001990, -33.88124999877096855, -97.00000000000000000 ) ) ;
#12492=ORIENTED_EDGE ( 'NONE', *, *, #17037, .T. ) ;
#12494=CARTESIAN_POINT ( 'NONE',  ( -83.90000000000000568, -33.46874999877096712, -97.40192378864668399 ) ) ;
#12499=DIRECTION ( 'NONE',  ( 0.000000000000000000, 0.000000000000000000, 1.000000000000000000 ) ) ;
#12501=CARTESIAN_POINT ( 'NONE',  ( 82.39999999999999147, -33.65624999877097423, -97.00000000000000000 ) ) ;
#12505=EDGE_CURVE ( 'NONE', #11141, #14672, #18877, .T. ) ;
#12506=DIRECTION ( 'NONE',  ( -0.000000000000000000, -0.000000000000000000, -1.000000000000000000 ) ) ;
#12508=CARTESIAN_POINT ( 'NONE',  ( -80.90000000000000568, -32.94374999877096855, -97.40192378864668399 ) ) ;
#12510=DIRECTION ( 'NONE',  ( -4.625929269271494788E-16, -1.000000000000000000, 0.000000000000000000 ) ) ;
#12518=CARTESIAN_POINT ( 'NONE',  ( 85.40000000000000568, -30.48749999999999716, -98.26794919243111792 ) ) ;
#12520=CARTESIAN_POINT ( 'NONE',  ( -79.39999999999999147, -33.80624999877097281, 101.7320508075688537 ) ) ;
#12522=CARTESIAN_POINT ( 'NONE',  ( 83.20384757729337366, -32.34240381056766722, -97.00000000000000000 ) ) ;
#12524=CARTESIAN_POINT ( 'NONE',  ( 85.15643035625001289, -33.85312499938549280, -99.99999999999998579 ) ) ;
#12526=CARTESIAN_POINT ( 'NONE',  ( -82.39999999999999147, -34.07812499938548711, 103.1828516163667899 ) ) ;
#12527=CARTESIAN_POINT ( 'NONE',  ( 82.39999999999999147, -32.95312499938548711, -96.81714838363319586 ) ) ;
#12529=( BOUNDED_CURVE ( )  B_SPLINE_CURVE ( 2, ( #1942, #18173, #493, #10641, #3215, #116, #13670, #14947, #10737 ),
 .UNSPECIFIED., .F., .F. ) 
 B_SPLINE_CURVE_WITH_KNOTS ( ( 3, 2, 2, 2, 3 ),
 ( 0.8541666666666665186, 0.8611111111111111605, 0.8750000000000000000, 0.8888888888888888395, 0.8958333333333333703 ),
 .UNSPECIFIED. ) 
 CURVE ( )  GEOMETRIC_REPRESENTATION_ITEM ( )  RATIONAL_B_SPLINE_CURVE ( ( 0.9330127018922194093, 0.9330127018922177440, 1.000000000000000000, 0.8660254037844387076, 1.000000000000000000, 0.8660254037844387076, 1.000000000000000000, 0.9330127018922187432, 0.9330127018922192983 ) ) 
 REPRESENTATION_ITEM ( '' )  );
#12531=DIRECTION ( 'NONE',  ( 0.000000000000000000, 0.000000000000000000, 1.000000000000000000 ) ) ;
#12536=CARTESIAN_POINT ( 'NONE',  ( -85.40000000000000568, -31.83750000000000568, 98.26794919243111792 ) ) ;
#12540=CARTESIAN_POINT ( 'NONE',  ( 85.15643035624999868, -31.52812499938547930, 101.5914258081833879 ) ) ;
#12541=VECTOR ( 'NONE', #2736, 1000.000000000000000 ) ;
#12543=CARTESIAN_POINT ( 'NONE',  ( 85.03799702444355546, -31.99999999999997868, -99.18121545504337178 ) ) ;
#12545=CARTESIAN_POINT ( 'NONE',  ( -79.64356964374999848, -32.72812499938548569, -99.99999999999998579 ) ) ;
#12546=CARTESIAN_POINT ( 'NONE',  ( 82.39999999999999147, -33.40312499938548285, 103.1828516163667899 ) ) ;
#12547=CARTESIAN_POINT ( 'NONE',  ( 81.02178482187500208, -32.80312499938548854, -102.3871387122750889 ) ) ;
#12549=CARTESIAN_POINT ( 'NONE',  ( -81.02178482187500208, -34.60312499938549280, 102.3871387122750889 ) ) ;
#12550=CARTESIAN_POINT ( 'NONE',  ( -83.77821517812500929, -34.22812499938549280, -97.61286128772489690 ) ) ;
#12552=CARTESIAN_POINT ( 'NONE',  ( 85.15643035624999868, -32.91562499938549280, 98.40857419181659793 ) ) ;
#12555=CARTESIAN_POINT ( 'NONE',  ( -81.02178482187500208, -31.79062499938548925, 102.3871387122750889 ) ) ;
#12557=CARTESIAN_POINT ( 'NONE',  ( -79.64356964374999848, -33.17812499938548854, 99.99999999999998579 ) ) ;
#12559=VERTEX_POINT ( 'NONE', #12207 ) ;
#12560=CARTESIAN_POINT ( 'NONE',  ( -79.39999999999999147, -34.27499999999999858, -99.99999999999998579 ) ) ;
#12561=ADVANCED_FACE ( 'NONE', ( #3027 ), #1853, .F. ) ;
#12563=CARTESIAN_POINT ( 'NONE',  ( 79.39999999999999147, -32.96250000000000568, -101.7320508075688537 ) ) ;
#12565=CARTESIAN_POINT ( 'NONE',  ( -85.15643035624999868, -34.71562499938548285, -98.40857419181659793 ) ) ;
#12570=CARTESIAN_POINT ( 'NONE',  ( 85.40000000000000568, -34.46249999999999858, -101.7320508075688821 ) ) ;
#12571=CARTESIAN_POINT ( 'NONE',  ( -83.90000000000000568, -33.46874999877096712, -97.40192378864668399 ) ) ;
#12574=LINE ( 'NONE', #7794, #12392 ) ;
#12575=CARTESIAN_POINT ( 'NONE',  ( 85.15643035624999868, -31.19062499938548783, -98.40857419181659793 ) ) ;
#12577=EDGE_CURVE ( 'NONE', #2207, #4201, #9229, .T. ) ;
#12579=CARTESIAN_POINT ( 'NONE',  ( 85.40000000000000568, -31.70624999877096784, 98.26794919243111792 ) ) ;
#12584=CARTESIAN_POINT ( 'NONE',  ( 82.40000000000000568, -34.10624999877096997, 102.9999999999999858 ) ) ;
#12587=CARTESIAN_POINT ( 'NONE',  ( -85.15643035624999868, -31.00312499938548072, -98.40857419181659793 ) ) ;
#12589=ORIENTED_EDGE ( 'NONE', *, *, #14382, .F. ) ;
#12590=CARTESIAN_POINT ( 'NONE',  ( 83.77821517812500929, -33.02812499938548285, 102.3871387122750889 ) ) ;
#12591=CARTESIAN_POINT ( 'NONE',  ( -80.90000000000000568, -34.74374999877097281, -97.40192378864668399 ) ) ;
#12592=CARTESIAN_POINT ( 'NONE',  ( 79.39999999999999147, -33.37500000000000000, 99.99999999999998579 ) ) ;
#12596=CYLINDRICAL_SURFACE ( 'NONE', #9137, 3.000000000000002665 ) ;
#12598=CARTESIAN_POINT ( 'NONE',  ( 79.39999999999999147, -34.25624999877096855, -101.7320508075688537 ) ) ;
#12602=CARTESIAN_POINT ( 'NONE',  ( 81.02178482187500208, -32.09062499938548285, -97.61286128772489690 ) ) ;
#12606=DIRECTION ( 'NONE',  ( 0.000000000000000000, -1.000000000000000000, 0.000000000000000000 ) ) ;
#12609=ORIENTED_EDGE ( 'NONE', *, *, #4040, .F. ) ;
#12613=CARTESIAN_POINT ( 'NONE',  ( -81.59615242270663771, -32.11740381056766580, -96.99999999999998579 ) ) ;
#12614=CARTESIAN_POINT ( 'NONE',  ( 82.39999999999999147, -30.56250000000000355, -96.53589838486223584 ) ) ;
#12615=CARTESIAN_POINT ( 'NONE',  ( -79.77811200999879304, -35.00000000000000000, -99.14934632385212865 ) ) ;
#12616=CARTESIAN_POINT ( 'NONE',  ( -85.40000000000000568, -34.48124999877096997, 98.26794919243111792 ) ) ;
#12618=EDGE_CURVE ( 'NONE', #3019, #1356, #4498, .T. ) ;
#12619=CARTESIAN_POINT ( 'NONE',  ( 82.39999999999999147, -32.36250000000000426, -96.99999999999997158 ) ) ;
#12623=CARTESIAN_POINT ( 'NONE',  ( -79.64356964374999848, -33.96562499938548285, 99.99999999999998579 ) ) ;
#12624=DIRECTION ( 'NONE',  ( -1.000000000000000000, 0.000000000000000000, 0.000000000000000000 ) ) ;
#12627=CARTESIAN_POINT ( 'NONE',  ( -80.90000000000000568, -34.20000000000000284, 97.40192378864668399 ) ) ;
#12630=CARTESIAN_POINT ( 'NONE',  ( 82.40000000000000568, -33.71249999999998437, 102.9999999999999858 ) ) ;
#12635=CARTESIAN_POINT ( 'NONE',  ( -81.59615242270662350, -33.73259618943233562, -102.9999999999999858 ) ) ;
#12636=CARTESIAN_POINT ( 'NONE',  ( 85.15643035624999868, -32.42812499938548854, 101.5914258081833879 ) ) ;
#12638=CARTESIAN_POINT ( 'NONE',  ( 79.39999999999999147, -32.02500000000000568, -99.99999999999998579 ) ) ;
#12641=CARTESIAN_POINT ( 'NONE',  ( 82.86160995759657055, -31.99999999999997158, 97.18959324165044222 ) ) ;
#12642=CARTESIAN_POINT ( 'NONE',  ( 82.39999999999999147, -31.37812499938548427, 96.81714838363319586 ) ) ;
#12643=CARTESIAN_POINT ( 'NONE',  ( 85.15643035624999868, -33.89062499938548711, -98.40857419181659793 ) ) ;
#12645=CARTESIAN_POINT ( 'NONE',  ( -82.39999999999999147, -33.06562499938548427, 96.81714838363319586 ) ) ;
#12646=CARTESIAN_POINT ( 'NONE',  ( -79.64356964374999848, -31.71562499938548285, -99.99999999999998579 ) ) ;
#12648=CARTESIAN_POINT ( 'NONE',  ( 79.64356964375001269, -32.76562499938548711, 98.40857419181659793 ) ) ;
#12653=CARTESIAN_POINT ( 'NONE',  ( -79.64356964374999848, -31.26562499938548356, 99.99999999999998579 ) ) ;
#12654=CARTESIAN_POINT ( 'NONE',  ( -79.64356964375001269, -33.66562499938549280, 101.5914258081833879 ) ) ;
#12657=CARTESIAN_POINT ( 'NONE',  ( -83.90000000000000568, -32.77499999999999858, -102.5980762113533018 ) ) ;
#12662=CARTESIAN_POINT ( 'NONE',  ( 82.40000000000000568, -30.00000000000000355, 103.0000000000000000 ) ) ;
#12664=CARTESIAN_POINT ( 'NONE',  ( 85.15643035624999868, -31.19062499938548783, 101.5914258081833879 ) ) ;
#12665=VECTOR ( 'NONE', #12013, 1000.000000000000000 ) ;
#12668=CARTESIAN_POINT ( 'NONE',  ( 85.15643035624999868, -32.01562499938548711, -101.5914258081833879 ) ) ;
#12671=VERTEX_POINT ( 'NONE', #17987 ) ;
#12672=CARTESIAN_POINT ( 'NONE',  ( 83.90000000000000568, -31.36874999877096926, 102.5980762113533018 ) ) ;
#12681=CARTESIAN_POINT ( 'NONE',  ( -81.02178482187500208, -32.24062499938548854, -97.61286128772489690 ) ) ;
#12682=CARTESIAN_POINT ( 'NONE',  ( -94.79999999999999716, -35.00000000000000000, -150.0000000000000000 ) ) ;
#12685=CARTESIAN_POINT ( 'NONE',  ( 85.15643035625001289, -33.85312499938549280, 99.99999999999998579 ) ) ;
#12686=CARTESIAN_POINT ( 'NONE',  ( -83.90000000000000568, -34.81874999877096855, -97.40192378864668399 ) ) ;
#12688=FACE_OUTER_BOUND ( 'NONE', #10709, .T. ) ;
#12689=CARTESIAN_POINT ( 'NONE',  ( -79.77811200999887831, -35.00000000000000000, 100.8506536761481414 ) ) ;
#12692=CARTESIAN_POINT ( 'NONE',  ( 85.29357727955090240, -35.00000000000000000, -100.3154961327749817 ) ) ;
#12695=VECTOR ( 'NONE', #13463, 1000.000000000000000 ) ;
#12699=CARTESIAN_POINT ( 'NONE',  ( 82.39999999999999147, -33.85312499938548569, -96.81714838363319586 ) ) ;
#12714=CARTESIAN_POINT ( 'NONE',  ( 80.90000000000000568, -33.89999999999999858, -102.5980762113533018 ) ) ;
#12715=DIRECTION ( 'NONE',  ( -0.000000000000000000, -1.000000000000000000, -0.000000000000000000 ) ) ;
#12717=( BOUNDED_CURVE ( )  B_SPLINE_CURVE ( 2, ( #2306, #5455, #9935, #16084, #14504, #15892, #858, #2690, #1049 ),
 .UNSPECIFIED., .F., .F. ) 
 B_SPLINE_CURVE_WITH_KNOTS ( ( 3, 2, 2, 2, 3 ),
 ( 0.4374999999999999445, 0.4444444444444444198, 0.4583333333333333148, 0.4722222222222222099, 0.4791666666666666297 ),
 .UNSPECIFIED. ) 
 CURVE ( )  GEOMETRIC_REPRESENTATION_ITEM ( )  RATIONAL_B_SPLINE_CURVE ( ( 0.9330127018922192983, 0.9330127018922187432, 1.000000000000000000, 0.8660254037844387076, 1.000000000000000000, 0.8660254037844387076, 1.000000000000000000, 0.9330127018922196314, 0.9330127018922194093 ) ) 
 REPRESENTATION_ITEM ( '' )  );
#12719=CARTESIAN_POINT ( 'NONE',  ( -82.39999999999999147, -35.23124999877096997, 103.4641016151377499 ) ) ;
#12722=CARTESIAN_POINT ( 'NONE',  ( 81.59615242270662350, -33.41115380933863577, 96.99999999999998579 ) ) ;
#12723=EDGE_CURVE ( 'NONE', #15743, #5107, #1888, .T. ) ;
#12724=CARTESIAN_POINT ( 'NONE',  ( 82.40000000000000568, -34.38749999999999574, 96.99999999999998579 ) ) ;
#12725=CIRCLE ( 'NONE', #6480, 2.649999999999982148 ) ;
#12727=CARTESIAN_POINT ( 'NONE',  ( -79.64356964375001269, -33.47812499938547859, 98.40857419181659793 ) ) ;
#12728=CARTESIAN_POINT ( 'NONE',  ( -96.99999999999998579, 0.000000000000000000, 150.0000000000000000 ) ) ;
#12739=CARTESIAN_POINT ( 'NONE',  ( -83.03192786677300319, -34.99999999999999289, -97.31096265645996368 ) ) ;
#12742=CARTESIAN_POINT ( 'NONE',  ( 85.15643035624999868, -32.80312499938548854, 98.40857419181659793 ) ) ;
#12747=CARTESIAN_POINT ( 'NONE',  ( -79.64356964374998427, -33.21562499938548996, -98.40857419181659793 ) ) ;
#12748=CARTESIAN_POINT ( 'NONE',  ( 79.64356964374999848, -33.06562499938548427, 99.99999999999998579 ) ) ;
#12749=CARTESIAN_POINT ( 'NONE',  ( 83.77821517812500929, -33.92812499938548854, -97.61286128772489690 ) ) ;
#12751=CARTESIAN_POINT ( 'NONE',  ( -82.39999999999999147, -32.95312499938548711, 96.81714838363319586 ) ) ;
#12753=CARTESIAN_POINT ( 'NONE',  ( 81.02178482187500208, -31.75312499938548427, 102.3871387122750889 ) ) ;
#12756=CARTESIAN_POINT ( 'NONE',  ( -85.15643035624999868, -30.17812499938548498, 98.40857419181659793 ) ) ;
#12757=CARTESIAN_POINT ( 'NONE',  ( -85.15643035624999868, -31.97812499938548925, 98.40857419181659793 ) ) ;
#12759=ORIENTED_EDGE ( 'NONE', *, *, #18852, .F. ) ;
#12761=CARTESIAN_POINT ( 'NONE',  ( -83.90000000000000568, -33.97500000000000853, -97.40192378864668399 ) ) ;
#12766=DIRECTION ( 'NONE',  ( 0.000000000000000000, 0.000000000000000000, 1.000000000000000000 ) ) ;
#12769=CARTESIAN_POINT ( 'NONE',  ( -83.20384757729335945, -33.00134618820329990, -96.99999999999997158 ) ) ;
#12770=( BOUNDED_CURVE ( )  B_SPLINE_CURVE ( 2, ( #17059, #15598, #18918, #17258, #753, #10023, #3765 ),
 .UNSPECIFIED., .F., .F. ) 
 B_SPLINE_CURVE_WITH_KNOTS ( ( 3, 2, 2, 3 ),
 ( 0.8958333333333333703, 0.9027777777777777901, 0.9166666666666666297, 0.9258785066912882389 ),
 .UNSPECIFIED. ) 
 CURVE ( )  GEOMETRIC_REPRESENTATION_ITEM ( )  RATIONAL_B_SPLINE_CURVE ( ( 0.9330127018922192983, 0.9330127018922198534, 1.000000000000000000, 0.8660254037844387076, 1.000000000000000000, 0.9111410165655264848, 0.9401539157124900736 ) ) 
 REPRESENTATION_ITEM ( '' )  );
#12772=CARTESIAN_POINT ( 'NONE',  ( 82.40000000000000568, -30.00000000000000355, -96.99999999999998579 ) ) ;
#12773=CARTESIAN_POINT ( 'NONE',  ( 85.15643035624999868, -30.66562499938548569, -101.5914258081833879 ) ) ;
#12774=CARTESIAN_POINT ( 'NONE',  ( -82.39999999999999147, -32.98124999877096286, 102.9999999999999858 ) ) ;
#12775=ORIENTED_EDGE ( 'NONE', *, *, #12327, .T. ) ;
#12776=CARTESIAN_POINT ( 'NONE',  ( 79.39999999999999147, -30.58124999877096784, 101.7320508075688821 ) ) ;
#12783=CARTESIAN_POINT ( 'NONE',  ( -81.02178482187500208, -30.44062499938548783, -97.61286128772489690 ) ) ;
#12784=DIRECTION ( 'NONE',  ( -0.000000000000000000, -1.000000000000000000, -0.000000000000000000 ) ) ;
#12785=ORIENTED_EDGE ( 'NONE', *, *, #13656, .F. ) ;
#12786=CARTESIAN_POINT ( 'NONE',  ( 79.64356964374999848, -34.52812499938548285, 99.99999999999998579 ) ) ;
#12787=CARTESIAN_POINT ( 'NONE',  ( -82.39999999999999147, -31.71562499938548640, -103.1828516163667899 ) ) ;
#12788=CARTESIAN_POINT ( 'NONE',  ( 83.90000000000000568, -34.42500000000000426, 97.40192378864668399 ) ) ;
#12792=CARTESIAN_POINT ( 'NONE',  ( -85.15643035625001289, -33.77812499938548285, -101.5914258081833879 ) ) ;
#12798=CARTESIAN_POINT ( 'NONE',  ( 85.15643035625001289, -32.87812499938548427, -98.40857419181659793 ) ) ;
#12802=EDGE_LOOP ( 'NONE', ( #11886, #14003, #8072, #1931 ) ) ;
#12808=EDGE_CURVE ( 'NONE', #1356, #18009, #12977, .T. ) ;
#12810=CARTESIAN_POINT ( 'NONE',  ( -79.58826230849692251, -32.00000000000093792, -101.0460072438472139 ) ) ;
#12811=CARTESIAN_POINT ( 'NONE',  ( 80.90000000000000568, -33.00000000000000000, -102.5980762113533018 ) ) ;
#12812=CARTESIAN_POINT ( 'NONE',  ( 82.40000000000000568, -30.00000000000000355, -103.0000000000000000 ) ) ;
#12815=CARTESIAN_POINT ( 'NONE',  ( -81.02178482187500208, -32.35312499938548569, 102.3871387122750889 ) ) ;
#12819=CARTESIAN_POINT ( 'NONE',  ( 83.77821517812500929, -32.01562499938548001, 102.3871387122750889 ) ) ;
#12820=CARTESIAN_POINT ( 'NONE',  ( 82.40000000000000568, -33.71249999999998437, 102.9999999999999858 ) ) ;
#12821=CARTESIAN_POINT ( 'NONE',  ( -79.64356964375001269, -34.82812499938548711, 98.40857419181659793 ) ) ;
#12823=ORIENTED_EDGE ( 'NONE', *, *, #8155, .F. ) ;
#12824=CARTESIAN_POINT ( 'NONE',  ( 81.59615242270662350, -32.83259618943233704, 102.9999999999999716 ) ) ;
#12830=EDGE_CURVE ( 'NONE', #11098, #3049, #4569, .T. ) ;
#12833=ORIENTED_EDGE ( 'NONE', *, *, #7219, .T. ) ;
#12837=CARTESIAN_POINT ( 'NONE',  ( 82.39999999999999147, -32.05312499938548854, 103.1828516163667899 ) ) ;
#12839=LINE ( 'NONE', #4143, #16719 ) ;
#12841=CARTESIAN_POINT ( 'NONE',  ( -83.77821517812500929, -34.37812499938548427, -102.3871387122750889 ) ) ;
#12842=CARTESIAN_POINT ( 'NONE',  ( 83.77821517812500929, -32.91562499938547859, 102.3871387122750889 ) ) ;
#12843=CARTESIAN_POINT ( 'NONE',  ( 85.15643035624999868, -34.34062499938548285, -98.40857419181659793 ) ) ;
#12845=CARTESIAN_POINT ( 'NONE',  ( -83.77821517812500929, -33.66562499938548569, 102.3871387122750889 ) ) ;
#12846=CARTESIAN_POINT ( 'NONE',  ( 81.02178482187500208, -30.89062499938548711, -102.3871387122750889 ) ) ;
#12847=VERTEX_POINT ( 'NONE', #1551 ) ;
#12851=CARTESIAN_POINT ( 'NONE',  ( -79.64356964375001269, -31.75312499938548427, 101.5914258081833879 ) ) ;
#12852=CARTESIAN_POINT ( 'NONE',  ( -85.15643035624999868, -30.55312499938548854, 101.5914258081833879 ) ) ;
#12854=CARTESIAN_POINT ( 'NONE',  ( -83.90000000000000568, -33.67500000000000426, -102.5980762113533018 ) ) ;
#12858=CARTESIAN_POINT ( 'NONE',  ( 83.41996205656103314, -34.99999999999999289, -97.17173842519744653 ) ) ;
#12865=CARTESIAN_POINT ( 'NONE',  ( 81.02178482187500208, -30.40312499938548640, 102.3871387122750889 ) ) ;
#12867=CARTESIAN_POINT ( 'NONE',  ( 85.15643035624999868, -34.79062499938548569, -98.40857419181659793 ) ) ;
#12870=CARTESIAN_POINT ( 'NONE',  ( 80.90000000000000568, -33.69374999877096855, 102.5980762113533018 ) ) ;
#12873=CARTESIAN_POINT ( 'NONE',  ( -79.64356964374999848, -30.47812499938548569, 99.99999999999998579 ) ) ;
#12874=CARTESIAN_POINT ( 'NONE',  ( -85.29357727954830182, -35.00000000000000711, -99.68450386720851952 ) ) ;
#12876=CARTESIAN_POINT ( 'NONE',  ( -85.15643035624999868, -31.45312499938548356, -98.40857419181659793 ) ) ;
#12877=CARTESIAN_POINT ( 'NONE',  ( 83.90000000000000568, -33.07500000000000284, 97.40192378864668399 ) ) ;
#12878=ORIENTED_EDGE ( 'NONE', *, *, #9240, .F. ) ;
#12879=CARTESIAN_POINT ( 'NONE',  ( 83.77821517812500929, -32.57812499938548711, 102.3871387122750889 ) ) ;
#12880=EDGE_CURVE ( 'NONE', #5078, #14237, #9560, .T. ) ;
#12881=CARTESIAN_POINT ( 'NONE',  ( -79.64356964374999848, -31.37812499938548427, -99.99999999999998579 ) ) ;
#12883=( BOUNDED_CURVE ( )  B_SPLINE_CURVE ( 2, ( #7374, #13430, #60, #16177, #8930, #10311, #11865, #13044, #3070 ),
 .UNSPECIFIED., .F., .F. ) 
 B_SPLINE_CURVE_WITH_KNOTS ( ( 3, 2, 2, 2, 3 ),
 ( 0.5208333333333333703, 0.5277777777777777901, 0.5416666666666666297, 0.5555555555555555802, 0.5625000000000000000 ),
 .UNSPECIFIED. ) 
 CURVE ( )  GEOMETRIC_REPRESENTATION_ITEM ( )  RATIONAL_B_SPLINE_CURVE ( ( 0.9330127018922192983, 0.9330127018922198534, 1.000000000000000000, 0.8660254037844387076, 1.000000000000000000, 0.8660254037844387076, 1.000000000000000000, 0.9330127018922194093, 0.9330127018922194093 ) ) 
 REPRESENTATION_ITEM ( '' )  );
#12884=CARTESIAN_POINT ( 'NONE',  ( -80.90000000000000568, -30.54374999877096997, -102.5980762113533018 ) ) ;
#12885=CARTESIAN_POINT ( 'NONE',  ( -79.67114894419042059, -35.00000000000001421, 99.22311565912312403 ) ) ;
#12888=CARTESIAN_POINT ( 'NONE',  ( -83.77821517812500929, -32.76562499938548711, -97.61286128772489690 ) ) ;
#12890=CARTESIAN_POINT ( 'NONE',  ( 79.39999999999999147, -32.90624999877096712, -101.7320508075688537 ) ) ;
#12893=CARTESIAN_POINT ( 'NONE',  ( 81.02178482187500208, -32.24062499938548854, -102.3871387122750889 ) ) ;
#12896=DIRECTION ( 'NONE',  ( -0.000000000000000000, -1.000000000000000000, -0.000000000000000000 ) ) ;
#12900=EDGE_CURVE ( 'NONE', #5530, #14645, #2074, .T. ) ;
#12902=CARTESIAN_POINT ( 'NONE',  ( 79.58826230851033756, -31.99999999999998579, 101.0460072438832952 ) ) ;
#12907=CARTESIAN_POINT ( 'NONE',  ( -94.79999999999999716, -29.80000000000000426, 150.0000000000000000 ) ) ;
#12908=CARTESIAN_POINT ( 'NONE',  ( 85.40000000000000568, -33.11250000000000426, -101.7320508075688679 ) ) ;
#12910=CARTESIAN_POINT ( 'NONE',  ( -85.15643035624999868, -31.11562499938548854, 101.5914258081833879 ) ) ;
#12912=CARTESIAN_POINT ( 'NONE',  ( -80.90000000000000568, -34.80000000000000426, -97.40192378864668399 ) ) ;
#12914=CARTESIAN_POINT ( 'NONE',  ( 85.15643035625001289, -34.79062499938548569, -98.40857419181659793 ) ) ;
#12915=CARTESIAN_POINT ( 'NONE',  ( -81.59615242270665192, -33.67634618820330417, 97.00000000000000000 ) ) ;
#12916=CARTESIAN_POINT ( 'NONE',  ( -85.15643035624999868, -34.67812499938548143, 98.40857419181659793 ) ) ;
#12925=VERTEX_POINT ( 'NONE', #9713 ) ;
#12927=CARTESIAN_POINT ( 'NONE',  ( -83.60689295392862164, -35.00000000000000000, -102.7535308243270293 ) ) ;
#12928=CARTESIAN_POINT ( 'NONE',  ( 79.64356964374999848, -34.86562499938548143, 99.99999999999998579 ) ) ;
#12929=DIRECTION ( 'NONE',  ( -0.000000000000000000, 0.000000000000000000, -1.000000000000000000 ) ) ;
#12933=CARTESIAN_POINT ( 'NONE',  ( -82.39999999999999147, -34.86562499938548854, -103.1828516163667899 ) ) ;
#12934=CARTESIAN_POINT ( 'NONE',  ( 82.39999999999999147, -32.95312499938548711, 103.1828516163667899 ) ) ;
#12935=CARTESIAN_POINT ( 'NONE',  ( 83.77821517812500929, -33.47812499938548569, -97.61286128772489690 ) ) ;
#12937=CARTESIAN_POINT ( 'NONE',  ( -81.02178482187500208, -34.04062499938548569, 102.3871387122750889 ) ) ;
#12938=CARTESIAN_POINT ( 'NONE',  ( 83.77821517812500929, -30.51562499938548711, -102.3871387122750889 ) ) ;
#12941=CARTESIAN_POINT ( 'NONE',  ( 85.15643035625001289, -35.20312499938548711, 99.99999999999998579 ) ) ;
#12944=CARTESIAN_POINT ( 'NONE',  ( -82.39999999999999147, -33.40312499938548285, 96.81714838363319586 ) ) ;
#12945=CARTESIAN_POINT ( 'NONE',  ( -85.15643035624999868, -31.00312499938548072, 101.5914258081833879 ) ) ;
#12946=DIRECTION ( 'NONE',  ( 0.000000000000000000, 0.000000000000000000, 1.000000000000000000 ) ) ;
#12947=AXIS2_PLACEMENT_3D ( 'NONE', #17262, #14216, #5252 ) ;
#12954=CARTESIAN_POINT ( 'NONE',  ( -84.70388354820684640, -35.00002705695768412, 98.07851859032987818 ) ) ;
#12955=CARTESIAN_POINT ( 'NONE',  ( -82.39999999999999147, -33.20624999877097849, -102.9999999999999858 ) ) ;
#12957=CARTESIAN_POINT ( 'NONE',  ( 85.15643035625001289, -30.25312499938548783, 99.99999999999998579 ) ) ;
#12961=CARTESIAN_POINT ( 'NONE',  ( 81.02178482187500208, -32.65312499938548996, -97.61286128772489690 ) ) ;
#12963=AXIS2_PLACEMENT_3D ( 'NONE', #11369, #6979, #13120 ) ;
#12965=CARTESIAN_POINT ( 'NONE',  ( 80.90000000000000568, -32.79374999877096997, 102.5980762113533018 ) ) ;
#12968=CARTESIAN_POINT ( 'NONE',  ( 83.20384757729338787, -34.59240381056766722, 102.9999999999999858 ) ) ;
#12972=CARTESIAN_POINT ( 'NONE',  ( -79.64356964375001269, -33.10312499938549280, -98.40857419181659793 ) ) ;
#12973=LINE ( 'NONE', #8385, #9110 ) ;
#12974=EDGE_LOOP ( 'NONE', ( #17305, #990, #11478, #17812 ) ) ;
#12975=CARTESIAN_POINT ( 'NONE',  ( 82.39999999999999147, -33.29062499938548569, 96.81714838363319586 ) ) ;
#12976=CARTESIAN_POINT ( 'NONE',  ( -85.15643035624999868, -31.56562499938548427, -98.40857419181659793 ) ) ;
#12977=CIRCLE ( 'NONE', #12992, 5.199999999999996625 ) ;
#12978=CARTESIAN_POINT ( 'NONE',  ( 85.40000000000000568, -34.53750000000000142, 101.7320508075688679 ) ) ;
#12982=CARTESIAN_POINT ( 'NONE',  ( -82.39999999999999147, -32.50312499938548427, -103.1828516163667899 ) ) ;
#12985=CARTESIAN_POINT ( 'NONE',  ( 82.39999999999999147, -32.08124999877097139, -103.4641016151377499 ) ) ;
#12988=ORIENTED_EDGE ( 'NONE', *, *, #17971, .F. ) ;
#12989=CARTESIAN_POINT ( 'NONE',  ( 82.39999999999999147, -34.75312499938548427, -96.81714838363319586 ) ) ;
#12992=AXIS2_PLACEMENT_3D ( 'NONE', #11803, #14722, #13547 ) ;
#12995=ORIENTED_EDGE ( 'NONE', *, *, #10081, .T. ) ;
#12996=ORIENTED_EDGE ( 'NONE', *, *, #17168, .T. ) ;
#12999=CARTESIAN_POINT ( 'NONE',  ( -83.20384757729338787, -32.10134618820330132, 102.9999999999999858 ) ) ;
#13001=CARTESIAN_POINT ( 'NONE',  ( 80.90000000000000568, -32.40000000000000568, -97.40192378864668399 ) ) ;
#13002=DIRECTION ( 'NONE',  ( 0.000000000000000000, 1.000000000000000000, 0.000000000000000000 ) ) ;
#13003=CARTESIAN_POINT ( 'NONE',  ( 79.58826230851033756, -31.99999999999998579, 101.0460072438832952 ) ) ;
#13004=CARTESIAN_POINT ( 'NONE',  ( -79.64356964375001269, -32.69062499938548427, 98.40857419181659793 ) ) ;
#13010=CYLINDRICAL_SURFACE ( 'NONE', #6516, 3.000000000000002665 ) ;
#13011=CARTESIAN_POINT ( 'NONE',  ( -96.99999999999998579, -29.80000000000000426, 150.0000000000000000 ) ) ;
#13015=CARTESIAN_POINT ( 'NONE',  ( -81.02178482187500208, -30.74062499938548498, -102.3871387122750889 ) ) ;
#13017=CYLINDRICAL_SURFACE ( 'NONE', #13940, 3.000000000000002665 ) ;
#13024=CARTESIAN_POINT ( 'NONE',  ( -83.90000000000000568, -30.76874999877097139, 102.5980762113533018 ) ) ;
#13025=CARTESIAN_POINT ( 'NONE',  ( 85.15643035624999868, -35.11426541925033007, 101.0032526477118751 ) ) ;
#13026=VECTOR ( 'NONE', #5416, 1000.000000000000000 ) ;
#13030=AXIS2_PLACEMENT_3D ( 'NONE', #14619, #4178, #10138 ) ;
#13031=CARTESIAN_POINT ( 'NONE',  ( -85.15643035625001289, -32.91562499938548569, -98.40857419181659793 ) ) ;
#13032=CARTESIAN_POINT ( 'NONE',  ( 79.64356964374999848, -33.51562499938548711, 99.99999999999998579 ) ) ;
#13033=CARTESIAN_POINT ( 'NONE',  ( 83.77821517812500929, -35.12812499938548427, -102.3871387122750889 ) ) ;
#13035=CARTESIAN_POINT ( 'NONE',  ( -81.02178482187500208, -32.69062499938548427, 102.3871387122750889 ) ) ;
#13036=CARTESIAN_POINT ( 'NONE',  ( 82.39999999999999147, -30.47812499938548569, -103.1828516163667899 ) ) ;
#13038=CYLINDRICAL_SURFACE ( 'NONE', #3814, 3.000000000000002665 ) ;
#13039=CARTESIAN_POINT ( 'NONE',  ( 82.40000000000001990, -33.88124999877096855, 97.00000000000000000 ) ) ;
#13041=CARTESIAN_POINT ( 'NONE',  ( -79.64356964375001269, -34.37812499938548427, 98.40857419181659793 ) ) ;
#13042=CARTESIAN_POINT ( 'NONE',  ( -85.15643035624999868, -31.52812499938547930, 98.40857419181659793 ) ) ;
#13043=ORIENTED_EDGE ( 'NONE', *, *, #12104, .F. ) ;
#13044=CARTESIAN_POINT ( 'NONE',  ( -81.59615242270662350, -33.01740381056767148, 102.9999999999999858 ) ) ;
#13052=CARTESIAN_POINT ( 'NONE',  ( -82.40000000000000568, -34.38749999999999574, 102.9999999999999858 ) ) ;
#13054=CARTESIAN_POINT ( 'NONE',  ( -81.59615242270662350, -33.22634618820330843, -102.9999999999999858 ) ) ;
#13056=CARTESIAN_POINT ( 'NONE',  ( 81.02178482187500208, -32.80312499938548854, 97.61286128772489690 ) ) ;
#13059=CARTESIAN_POINT ( 'NONE',  ( 79.64356964375001269, -33.66562499938549280, -101.5914258081833879 ) ) ;
#13060=CIRCLE ( 'NONE', #15563, 2.649999999999982148 ) ;
#13063=CARTESIAN_POINT ( 'NONE',  ( 82.39999999999999147, -32.53124999877096712, 96.53589838486223584 ) ) ;
#13065=CARTESIAN_POINT ( 'NONE',  ( 83.90000000000000568, -32.56874999877096855, 97.40192378864668399 ) ) ;
#13067=CARTESIAN_POINT ( 'NONE',  ( 83.20384757729335945, -34.40759618943233988, 96.99999999999998579 ) ) ;
#13068=CARTESIAN_POINT ( 'NONE',  ( -82.40000000000000568, -30.00000000000000355, 99.99999999999998579 ) ) ;
#13069=ORIENTED_EDGE ( 'NONE', *, *, #17408, .F. ) ;
#13070=CARTESIAN_POINT ( 'NONE',  ( -85.15643035624999868, -33.77812499938548285, -101.5914258081833879 ) ) ;
#13071=ADVANCED_FACE ( 'NONE', ( #17527 ), #6978, .F. ) ;
#13072=DIRECTION ( 'NONE',  ( -0.000000000000000000, -1.000000000000000000, -0.000000000000000000 ) ) ;
#13073=VERTEX_POINT ( 'NONE', #17435 ) ;
#13074=CARTESIAN_POINT ( 'NONE',  ( -82.39999999999999147, -30.36562499938549209, -103.1828516163667899 ) ) ;
#13075=CARTESIAN_POINT ( 'NONE',  ( -83.90000000000000568, -31.66874999877096997, -97.40192378864668399 ) ) ;
#13078=CARTESIAN_POINT ( 'NONE',  ( -85.15643035625001289, -32.80312499938548854, -98.40857419181659793 ) ) ;
#13080=CARTESIAN_POINT ( 'NONE',  ( 80.90000000000000568, -32.04374999877096997, -102.5980762113533018 ) ) ;
#13083=CARTESIAN_POINT ( 'NONE',  ( 96.99999999999998579, 4.758098676964956264E-15, 150.0000000000000000 ) ) ;
#13089=VERTEX_POINT ( 'NONE', #5619 ) ;
#13090=VERTEX_POINT ( 'NONE', #18997 ) ;
#13091=CARTESIAN_POINT ( 'NONE',  ( 79.39999999999999147, -34.23750000000000426, -98.26794919243110371 ) ) ;
#13093=VERTEX_POINT ( 'NONE', #11564 ) ;
#13094=CARTESIAN_POINT ( 'NONE',  ( 82.40000000000001990, -32.53124999877097423, -103.0000000000000000 ) ) ;
#13095=CARTESIAN_POINT ( 'NONE',  ( 80.90000000000000568, -33.30000000000000426, -97.40192378864668399 ) ) ;
#13096=EDGE_CURVE ( 'NONE', #5485, #5078, #15960, .T. ) ;
#13098=CARTESIAN_POINT ( 'NONE',  ( -81.02178482187500208, -31.30312499938548498, 97.61286128772489690 ) ) ;
#13100=LINE ( 'NONE', #16237, #11488 ) ;
#13101=ADVANCED_FACE ( 'NONE', ( #17622 ), #7357, .F. ) ;
#13103=CARTESIAN_POINT ( 'NONE',  ( -81.02178482187500208, -34.94062499938548427, 102.3871387122750889 ) ) ;
#13106=FILL_AREA_STYLE_COLOUR ( '', #15204 ) ;
#13107=CARTESIAN_POINT ( 'NONE',  ( -85.15643035625001289, -31.94062499938548427, -99.99999999999998579 ) ) ;
#13108=CARTESIAN_POINT ( 'NONE',  ( 85.40000000000000568, -34.89374999877097139, 99.99999999999998579 ) ) ;
#13113=VERTEX_POINT ( 'NONE', #4139 ) ;
#13117=CARTESIAN_POINT ( 'NONE',  ( 85.15643035624999868, -33.70312499938548711, 98.40857419181659793 ) ) ;
#13118=DIRECTION ( 'NONE',  ( 0.000000000000000000, 0.000000000000000000, -1.000000000000000000 ) ) ;
#13120=DIRECTION ( 'NONE',  ( 0.000000000000000000, 0.000000000000000000, -1.000000000000000000 ) ) ;
#13121=CARTESIAN_POINT ( 'NONE',  ( -79.39999999999999147, -33.78750000000000853, 98.26794919243110371 ) ) ;
#13122=CARTESIAN_POINT ( 'NONE',  ( -81.02178482187500208, -33.55312499938548854, -102.3871387122750889 ) ) ;
#13123=CARTESIAN_POINT ( 'NONE',  ( 79.64356964374999848, -34.86562499938548143, 99.99999999999998579 ) ) ;
#13124=CARTESIAN_POINT ( 'NONE',  ( 82.39999999999999147, -30.47812499938548569, -103.1828516163667899 ) ) ;
#13126=CARTESIAN_POINT ( 'NONE',  ( -79.64356964374998427, -33.02812499938548285, 98.40857419181659793 ) ) ;
#13127=CARTESIAN_POINT ( 'NONE',  ( 81.02178482187500208, -30.29062499938548569, -97.61286128772489690 ) ) ;
#13128=VERTEX_POINT ( 'NONE', #8529 ) ;
#13131=CARTESIAN_POINT ( 'NONE',  ( -85.15643035624999868, -33.77812499938548285, 98.40857419181659793 ) ) ;
#13136=CARTESIAN_POINT ( 'NONE',  ( 85.40000000000000568, -33.56250000000000000, -101.7320508075688821 ) ) ;
#13137=CARTESIAN_POINT ( 'NONE',  ( -85.40000000000000568, -34.50000000000000000, 99.99999999999998579 ) ) ;
#13140=CARTESIAN_POINT ( 'NONE',  ( -94.79999999999999716, 0.000000000000000000, 150.0000000000000000 ) ) ;
#13141=CARTESIAN_POINT ( 'NONE',  ( 82.39999999999999147, -33.74062499938548854, 96.81714838363319586 ) ) ;
#13144=CARTESIAN_POINT ( 'NONE',  ( 82.39999999999999147, -33.74062499938548854, -103.1828516163667899 ) ) ;
#13145=CARTESIAN_POINT ( 'NONE',  ( -85.15643035625001289, -31.15312499938548996, -99.99999999999998579 ) ) ;
#13147=CARTESIAN_POINT ( 'NONE',  ( 85.40000000000000568, -32.68124999877097281, 101.7320508075688679 ) ) ;
#13149=PLANE ( 'NONE',  #14893 ) ;
#13151=CIRCLE ( 'NONE', #16919, 2.199999999999993516 ) ;
#13153=CLOSED_SHELL ( 'NONE', ( #15436, #1868, #5200, #6379, #18251, #7845, #2083, #18309, #2062, #1135, #15453, #18667, #2439, #14964, #3066, #12230, #8335, #16441, #15592, #1448, #6426, #14518, #4210, #13767, #16034, #1975, #10710, #1990, #11433, #6973, #2337, #3252, #4828, #6012, #14929, #12208, #13661, #8059, #14850, #12267, #12350, #15081, #13101, #18489, #8552, #10885, #4604, #8522, #13071, #17249, #4965, #4361, #10776, #9099, #5678, #9755, #3160, #18071, #7821, #3844, #17629, #14361, #5962, #9965, #15684, #18920, #5792, #11617, #2590, #1080, #17860, #9122, #2699, #2069, #16793, #8447, #19140, #17802, #15702, #16540, #18807, #13171, #12561, #3742, #14739, #1527, #17715, #1677, #2193, #17225, #10685, #13995, #3156, #17137, #6988, #9950, #9041, #16217, #10694, #14138, #6260, #15587, #1287, #831, #10681, #18072, #1744, #17112 ) ) ;
#13156=EDGE_LOOP ( 'NONE', ( #12785, #6100, #17980, #12286 ) ) ;
#13157=CARTESIAN_POINT ( 'NONE',  ( -83.77821517812500929, -34.71562499938548285, -102.3871387122750889 ) ) ;
#13159=ORIENTED_EDGE ( 'NONE', *, *, #8801, .T. ) ;
#13161=CARTESIAN_POINT ( 'NONE',  ( -85.15643035625001289, -30.25312499938548783, -99.99999999999998579 ) ) ;
#13163=CARTESIAN_POINT ( 'NONE',  ( -82.39999999999999147, -31.40624999877097068, -103.4641016151377499 ) ) ;
#13168=CARTESIAN_POINT ( 'NONE',  ( -82.39999999999999147, -33.62812499938548427, -96.81714838363319586 ) ) ;
#13169=CARTESIAN_POINT ( 'NONE',  ( 82.39999999999999147, -32.58750000000000568, -102.9999999999999858 ) ) ;
#13171=ADVANCED_FACE ( 'NONE', ( #19289 ), #7260, .T. ) ;
#13173=CARTESIAN_POINT ( 'NONE',  ( 83.90000000000000568, -31.21874999877097068, -102.5980762113533018 ) ) ;
#13176=CARTESIAN_POINT ( 'NONE',  ( 85.15643035625001289, -34.19062499938548427, -99.99999999999998579 ) ) ;
#13179=EDGE_CURVE ( 'NONE', #16539, #11084, #7236, .T. ) ;
#13182=ORIENTED_EDGE ( 'NONE', *, *, #4818, .F. ) ;
#13183=CARTESIAN_POINT ( 'NONE',  ( 82.40000000000001990, -34.16250000000000853, -97.00000000000000000 ) ) ;
#13185=CARTESIAN_POINT ( 'NONE',  ( -82.49978216248248941, -35.00000000000000000, -97.23961338448006586 ) ) ;
#13188=ORIENTED_EDGE ( 'NONE', *, *, #12880, .T. ) ;
#13189=CARTESIAN_POINT ( 'NONE',  ( 79.39999999999999147, -32.45624999877097139, -101.7320508075688537 ) ) ;
#13192=CARTESIAN_POINT ( 'NONE',  ( -85.15643035624999868, -31.19062499938548783, 98.40857419181659793 ) ) ;
#13194=CARTESIAN_POINT ( 'NONE',  ( -82.40000000000000568, -30.00000000000000355, 103.0000000000000000 ) ) ;
#13195=CARTESIAN_POINT ( 'NONE',  ( 82.40000000000000568, -33.71249999999998437, -96.99999999999998579 ) ) ;
#13196=LINE ( 'NONE', #4121, #9003 ) ;
#13197=CARTESIAN_POINT ( 'NONE',  ( -79.64356964375001269, -34.45312499938548711, 101.5914258081833879 ) ) ;
#13198=AXIS2_PLACEMENT_3D ( 'NONE', #2253, #17013, #2166 ) ;
#13199=CARTESIAN_POINT ( 'NONE',  ( -82.39999999999999147, -34.33124999877097139, -97.00000000000000000 ) ) ;
#13201=CARTESIAN_POINT ( 'NONE',  ( -79.64356964375001269, -31.67812499938548143, -101.5914258081833879 ) ) ;
#13214=CARTESIAN_POINT ( 'NONE',  ( 85.40000000000000568, -30.00000000000000355, 99.99999999999998579 ) ) ;
#13215=CARTESIAN_POINT ( 'NONE',  ( 83.90000000000000568, -34.12500000000000000, -97.40192378864668399 ) ) ;
#13219=CARTESIAN_POINT ( 'NONE',  ( 83.77821517812500929, -34.26562499938548711, 102.3871387122750889 ) ) ;
#13221=CARTESIAN_POINT ( 'NONE',  ( 83.77821517812500929, -30.51562499938548711, -102.3871387122750889 ) ) ;
#13226=CARTESIAN_POINT ( 'NONE',  ( 82.39999999999999147, -35.09062499938548285, 96.81714838363319586 ) ) ;
#13229=CARTESIAN_POINT ( 'NONE',  ( -79.64356964375001269, -32.65312499938548285, 101.5914258081833879 ) ) ;
#13230=ORIENTED_EDGE ( 'NONE', *, *, #13179, .T. ) ;
#13231=CARTESIAN_POINT ( 'NONE',  ( -84.06832524826180020, -35.00000000000001421, 102.2567273996599226 ) ) ;
#13236=CARTESIAN_POINT ( 'NONE',  ( -85.40000000000000568, -33.14999999999999858, -99.99999999999998579 ) ) ;
#13240=CARTESIAN_POINT ( 'NONE',  ( 82.39999999999999147, -32.84062499938548996, 96.81714838363319586 ) ) ;
#13241=CARTESIAN_POINT ( 'NONE',  ( 79.68596062386926349, -32.00000000000000000, 98.72172371342817598 ) ) ;
#13244=CARTESIAN_POINT ( 'NONE',  ( 85.15643035624999868, -34.26562499938548711, -101.5914258081833879 ) ) ;
#13245=CARTESIAN_POINT ( 'NONE',  ( -83.77821517812500929, -30.77812499938548640, -102.3871387122750889 ) ) ;
#13247=CARTESIAN_POINT ( 'NONE',  ( 85.40000000000000568, -33.09374999877096712, 99.99999999999998579 ) ) ;
#13251=CARTESIAN_POINT ( 'NONE',  ( 83.90000000000000568, -34.57500000000000284, 102.5980762113533018 ) ) ;
#13252=CARTESIAN_POINT ( 'NONE',  ( 81.59615242270665192, -33.67634618820330417, -97.00000000000000000 ) ) ;
#13253=ORIENTED_EDGE ( 'NONE', *, *, #4469, .F. ) ;
#13254=CARTESIAN_POINT ( 'NONE',  ( -81.02178482187500208, -32.99062499938548854, -102.3871387122750889 ) ) ;
#13256=ORIENTED_EDGE ( 'NONE', *, *, #6194, .T. ) ;
#13258=CARTESIAN_POINT ( 'NONE',  ( -79.64356964375001269, -33.14062499938548711, -101.5914258081833879 ) ) ;
#13259=CARTESIAN_POINT ( 'NONE',  ( -83.52022063337570046, -32.00000000000000000, -102.5731757466075180 ) ) ;
#13260=CARTESIAN_POINT ( 'NONE',  ( -85.40000000000000568, -31.25624999877096855, -98.26794919243111792 ) ) ;
#13264=CARTESIAN_POINT ( 'NONE',  ( -85.40000000000000568, -33.58124999877097139, 98.26794919243111792 ) ) ;
#13265=CARTESIAN_POINT ( 'NONE',  ( -82.40000000000000568, -30.00000000000000355, 96.99999999999998579 ) ) ;
#13266=( BOUNDED_CURVE ( )  B_SPLINE_CURVE ( 2, ( #19178, #11745, #17712, #2856, #8813, #19277, #15348, #9383, #12033 ),
 .UNSPECIFIED., .F., .F. ) 
 B_SPLINE_CURVE_WITH_KNOTS ( ( 3, 2, 2, 2, 3 ),
 ( 0.6041666666666666297, 0.6111111111111111605, 0.6250000000000000000, 0.6388888888888888395, 0.6458333333333332593 ),
 .UNSPECIFIED. ) 
 CURVE ( )  GEOMETRIC_REPRESENTATION_ITEM ( )  RATIONAL_B_SPLINE_CURVE ( ( 0.9330127018922192983, 0.9330127018922187432, 1.000000000000000000, 0.8660254037844387076, 1.000000000000000000, 0.8660254037844387076, 1.000000000000000000, 0.9330127018922198534, 0.9330127018922192983 ) ) 
 REPRESENTATION_ITEM ( '' )  );
#13267=CYLINDRICAL_SURFACE ( 'NONE', #547, 3.000000000000002665 ) ;
#13268=CARTESIAN_POINT ( 'NONE',  ( 85.40000000000000568, -30.80624999877096926, -101.7320508075688679 ) ) ;
#13270=VERTEX_POINT ( 'NONE', #13702 ) ;
#13271=CARTESIAN_POINT ( 'NONE',  ( 82.05869624310412291, -34.96883842999723413, -102.9857998004475235 ) ) ;
#13275=VERTEX_POINT ( 'NONE', #6195 ) ;
#13283=DIRECTION ( 'NONE',  ( 0.000000000000000000, -1.000000000000000000, 0.000000000000000000 ) ) ;
#13284=DIRECTION ( 'NONE',  ( 1.000000000000000000, 0.000000000000000000, 4.625929269271481378E-15 ) ) ;
#13285=CARTESIAN_POINT ( 'NONE',  ( -85.15643035624999868, -33.89062499938548711, 98.40857419181659793 ) ) ;
#13289=EDGE_CURVE ( 'NONE', #19014, #4990, #14438, .T. ) ;
#13291=CARTESIAN_POINT ( 'NONE',  ( -82.17437583783130606, -35.00000000000002132, -102.9802575795477537 ) ) ;
#13292=VECTOR ( 'NONE', #4916, 1000.000000000000000 ) ;
#13294=EDGE_LOOP ( 'NONE', ( #13627, #17703, #11235, #14538 ) ) ;
#13295=CARTESIAN_POINT ( 'NONE',  ( -79.64356964374999848, -34.97812499938548569, -99.99999999999998579 ) ) ;
#13305=CARTESIAN_POINT ( 'NONE',  ( -85.15643035624999868, -32.09062499938548996, 98.40857419181659793 ) ) ;
#13308=ORIENTED_EDGE ( 'NONE', *, *, #4701, .F. ) ;
#13309=PLANE ( 'NONE',  #437 ) ;
#13311=EDGE_CURVE ( 'NONE', #11864, #18009, #14977, .T. ) ;
#13312=CARTESIAN_POINT ( 'NONE',  ( -79.39999999999999147, -31.06874999877096855, 99.99999999999998579 ) ) ;
#13313=CARTESIAN_POINT ( 'NONE',  ( 81.02178482187500208, -34.49062499938548854, 97.61286128772489690 ) ) ;
#13317=CARTESIAN_POINT ( 'NONE',  ( 85.15643035625001289, -34.64062499938548711, 99.99999999999998579 ) ) ;
#13318=CARTESIAN_POINT ( 'NONE',  ( 81.02178482187500208, -30.74062499938548498, -97.61286128772489690 ) ) ;
#13321=CARTESIAN_POINT ( 'NONE',  ( -85.15643035625001289, -34.67812499938548143, 98.40857419181659793 ) ) ;
#13322=CARTESIAN_POINT ( 'NONE',  ( 85.15643035625001289, -33.74062499938548854, -99.99999999999998579 ) ) ;
#13323=VECTOR ( 'NONE', #10435, 1000.000000000000000 ) ;
#13324=ORIENTED_EDGE ( 'NONE', *, *, #5431, .F. ) ;
#13325=DIRECTION ( 'NONE',  ( -0.000000000000000000, -0.000000000000000000, -1.000000000000000000 ) ) ;
#13326=CARTESIAN_POINT ( 'NONE',  ( 80.90000000000000568, -33.75000000000000000, -97.40192378864668399 ) ) ;
#13328=CARTESIAN_POINT ( 'NONE',  ( -85.40000000000000568, -30.45000000000000284, 99.99999999999998579 ) ) ;
#13329=EDGE_LOOP ( 'NONE', ( #8805, #6255, #14522, #9881 ) ) ;
#13332=CARTESIAN_POINT ( 'NONE',  ( -81.59615242270665192, -34.18259618943233136, 97.00000000000000000 ) ) ;
#13335=EDGE_CURVE ( 'NONE', #10447, #12229, #5903, .T. ) ;
#13336=VECTOR ( 'NONE', #17946, 1000.000000000000000 ) ;
#13337=( BOUNDED_CURVE ( )  B_SPLINE_CURVE ( 2, ( #8894, #8997, #13486, #18186, #1674, #127, #4808, #19266, #12125 ),
 .UNSPECIFIED., .F., .F. ) 
 B_SPLINE_CURVE_WITH_KNOTS ( ( 3, 2, 2, 2, 3 ),
 ( 0.7708333333333331483, 0.7777777777777777901, 0.7916666666666666297, 0.8055555555555555802, 0.8125000000000001110 ),
 .UNSPECIFIED. ) 
 CURVE ( )  GEOMETRIC_REPRESENTATION_ITEM ( )  RATIONAL_B_SPLINE_CURVE ( ( 0.9330127018922194093, 0.9330127018922177440, 1.000000000000000000, 0.8660254037844387076, 1.000000000000000000, 0.8660254037844387076, 1.000000000000000000, 0.9330127018922182991, 0.9330127018922194093 ) ) 
 REPRESENTATION_ITEM ( '' )  );
#13339=CARTESIAN_POINT ( 'NONE',  ( -79.39999999999999147, -32.38124999877096855, 98.26794919243110371 ) ) ;
#13342=CARTESIAN_POINT ( 'NONE',  ( 85.15643035625001289, -32.05312499938548854, 99.99999999999998579 ) ) ;
#13343=CARTESIAN_POINT ( 'NONE',  ( 82.40000000000000568, -30.00000000000000355, 103.0000000000000000 ) ) ;
#13345=EDGE_CURVE ( 'NONE', #7737, #17378, #10712, .T. ) ;
#13347=CARTESIAN_POINT ( 'NONE',  ( -85.15643035624999868, -32.02817623523065294, 101.0587761908873290 ) ) ;
#13348=CARTESIAN_POINT ( 'NONE',  ( -79.64356964375001269, -31.41562499938548569, -98.40857419181659793 ) ) ;
#13349=VERTEX_POINT ( 'NONE', #17916 ) ;
#13350=CARTESIAN_POINT ( 'NONE',  ( 84.69813954184694182, -35.39427337414329600, 101.9283554252781272 ) ) ;
#13353=VECTOR ( 'NONE', #2548, 1000.000000000000000 ) ;
#13354=VECTOR ( 'NONE', #721, 1000.000000000000000 ) ;
#13355=CARTESIAN_POINT ( 'NONE',  ( -85.15643035624999868, -32.01562499938548711, 101.5914258081833879 ) ) ;
#13357=ORIENTED_EDGE ( 'NONE', *, *, #18220, .F. ) ;
#13358=CARTESIAN_POINT ( 'NONE',  ( -83.88339518848731302, -35.16733441503058089, -102.5204086375588162 ) ) ;
#13362=CARTESIAN_POINT ( 'NONE',  ( -81.02178482187500208, -33.25312499938548427, -97.61286128772489690 ) ) ;
#13363=CARTESIAN_POINT ( 'NONE',  ( -82.85293433256504159, -32.00000000000002132, -102.8010948079636080 ) ) ;
#13364=CARTESIAN_POINT ( 'NONE',  ( -85.40000000000000568, -30.88124999877097210, -101.7320508075688679 ) ) ;
#13368=CARTESIAN_POINT ( 'NONE',  ( -81.02178482187500208, -34.94062499938548427, -97.61286128772489690 ) ) ;
#13369=CARTESIAN_POINT ( 'NONE',  ( 83.77821517812500929, -34.26562499938548711, 102.3871387122750889 ) ) ;
#13370=PLANE ( 'NONE',  #5559 ) ;
#13372=CARTESIAN_POINT ( 'NONE',  ( 83.90000000000000568, -33.91874999877096997, -102.5980762113533018 ) ) ;
#13374=VERTEX_POINT ( 'NONE', #3242 ) ;
#13375=CARTESIAN_POINT ( 'NONE',  ( 79.64356964374998427, -34.90312499938548285, -101.5914258081833879 ) ) ;
#13379=EDGE_LOOP ( 'NONE', ( #8, #3829, #14290, #5013 ) ) ;
#13383=CARTESIAN_POINT ( 'NONE',  ( -85.40000000000000568, -32.15624999877096712, 101.7320508075688821 ) ) ;
#13385=CARTESIAN_POINT ( 'NONE',  ( -83.20395887649198130, -35.00000000000002132, 102.6365808225363025 ) ) ;
#13387=CARTESIAN_POINT ( 'NONE',  ( -83.77821517812500929, -33.32812499938548711, 102.3871387122750889 ) ) ;
#13398=CARTESIAN_POINT ( 'NONE',  ( -79.64356964375001269, -33.10312499938549280, -98.40857419181659793 ) ) ;
#13400=CARTESIAN_POINT ( 'NONE',  ( -82.40000000000000568, -30.00000000000000355, -103.0000000000000000 ) ) ;
#13401=CARTESIAN_POINT ( 'NONE',  ( 79.83361526238435601, -35.00000000000000711, -101.0217260113603572 ) ) ;
#13407=ORIENTED_EDGE ( 'NONE', *, *, #3268, .F. ) ;
#13408=VERTEX_POINT ( 'NONE', #3821 ) ;
#13409=CARTESIAN_POINT ( 'NONE',  ( -85.11512745526620449, -32.00000000000000000, 100.5952676699193802 ) ) ;
#13411=CARTESIAN_POINT ( 'NONE',  ( -85.40000000000000568, -31.74374999877096926, 99.99999999999998579 ) ) ;
#13412=CARTESIAN_POINT ( 'NONE',  ( 85.40000000000000568, -31.76249999999999929, 98.26794919243111792 ) ) ;
#13416=CARTESIAN_POINT ( 'NONE',  ( 85.15643035624999868, -35.11426555956768425, 101.0032586025029815 ) ) ;
#13419=CARTESIAN_POINT ( 'NONE',  ( 85.15643035624999868, -31.52812499938547930, -98.40857419181659793 ) ) ;
#13420=ORIENTED_EDGE ( 'NONE', *, *, #5795, .T. ) ;
#13422=EDGE_CURVE ( 'NONE', #5491, #2466, #7429, .T. ) ;
#13424=CARTESIAN_POINT ( 'NONE',  ( 85.15643035624999868, -34.22812499938547859, -98.40857419181659793 ) ) ;
#13428=CARTESIAN_POINT ( 'NONE',  ( -79.39999999999999147, -30.22500000000000142, 99.99999999999998579 ) ) ;
#13430=CARTESIAN_POINT ( 'NONE',  ( -81.59615242270662350, -32.83259618943233704, 96.99999999999998579 ) ) ;
#13432=LINE ( 'NONE', #3166, #15786 ) ;
#13434=CARTESIAN_POINT ( 'NONE',  ( 82.40000000000001990, -32.30624999877097281, -97.00000000000000000 ) ) ;
#13438=CARTESIAN_POINT ( 'NONE',  ( 85.15643035625001289, -31.60312499938548569, 99.99999999999998579 ) ) ;
#13440=CARTESIAN_POINT ( 'NONE',  ( -81.02178482187500208, -32.65312499938548996, 97.61286128772489690 ) ) ;
#13441=CARTESIAN_POINT ( 'NONE',  ( -85.15643035625001289, -30.70312499938548711, -99.99999999999998579 ) ) ;
#13443=CARTESIAN_POINT ( 'NONE',  ( 85.40000000000000568, -34.85624999877096997, 98.26794919243111792 ) ) ;
#13447=CARTESIAN_POINT ( 'NONE',  ( -85.15643035625001289, -32.05312499938548854, 99.99999999999998579 ) ) ;
#13448=CARTESIAN_POINT ( 'NONE',  ( 84.11496519894906498, -31.99999999999998579, 102.1846009218925104 ) ) ;
#13449=ORIENTED_EDGE ( 'NONE', *, *, #9393, .F. ) ;
#13450=CARTESIAN_POINT ( 'NONE',  ( -83.90000000000000568, -30.07499999999999929, -102.5980762113533018 ) ) ;
#13451=( BOUNDED_CURVE ( )  B_SPLINE_CURVE ( 2, ( #3, #11899, #98, #3008, #14633, #17870, #5757, #10533, #13169 ),
 .UNSPECIFIED., .F., .F. ) 
 B_SPLINE_CURVE_WITH_KNOTS ( ( 3, 2, 2, 2, 3 ),
 ( 0.4375000000000000555, 0.4444444444444444198, 0.4583333333333333148, 0.4722222222222222099, 0.4791666666666666297 ),
 .UNSPECIFIED. ) 
 CURVE ( )  GEOMETRIC_REPRESENTATION_ITEM ( )  RATIONAL_B_SPLINE_CURVE ( ( 0.9330127018922192983, 0.9330127018922198534, 1.000000000000000000, 0.8660254037844387076, 1.000000000000000000, 0.8660254037844387076, 1.000000000000000000, 0.9330127018922196314, 0.9330127018922194093 ) ) 
 REPRESENTATION_ITEM ( '' )  );
#13453=DIRECTION ( 'NONE',  ( -0.000000000000000000, -1.000000000000000000, -0.000000000000000000 ) ) ;
#13455=CARTESIAN_POINT ( 'NONE',  ( -79.64356964375001269, -33.21562499938548996, -98.40857419181659793 ) ) ;
#13461=CARTESIAN_POINT ( 'NONE',  ( 82.39999999999999147, -32.72812499938548569, 96.81714838363319586 ) ) ;
#13462=FACE_OUTER_BOUND ( 'NONE', #12351, .T. ) ;
#13463=DIRECTION ( 'NONE',  ( -0.000000000000000000, -0.000000000000000000, -1.000000000000000000 ) ) ;
#13464=CARTESIAN_POINT ( 'NONE',  ( 79.39999999999999147, -33.31874999877096855, -99.99999999999998579 ) ) ;
#13478=LINE ( 'NONE', #118, #176 ) ;
#13480=CARTESIAN_POINT ( 'NONE',  ( -81.02178482187500208, -33.25312499938548427, 102.3871387122750889 ) ) ;
#13483=CARTESIAN_POINT ( 'NONE',  ( 82.40000000000001990, -32.75624999877096855, 103.0000000000000000 ) ) ;
#13485=CARTESIAN_POINT ( 'NONE',  ( 82.40000000000000568, -30.00000000000000355, 99.99999999999998579 ) ) ;
#13486=CARTESIAN_POINT ( 'NONE',  ( -80.90000000000000568, -34.59374999877096712, -102.5980762113533018 ) ) ;
#13487=CARTESIAN_POINT ( 'NONE',  ( -85.40000000000000568, -34.40624999877096712, -98.26794919243111792 ) ) ;
#13489=EDGE_CURVE ( 'NONE', #11146, #4397, #17340, .T. ) ;
#13490=CARTESIAN_POINT ( 'NONE',  ( -85.15643035624999868, -33.32812499938548001, -101.5914258081833879 ) ) ;
#13493=AXIS2_PLACEMENT_3D ( 'NONE', #14064, #6457, #13967 ) ;
#13495=CARTESIAN_POINT ( 'NONE',  ( 82.32247963938024782, -34.99999999999999289, -102.7610832838413444 ) ) ;
#13497=CARTESIAN_POINT ( 'NONE',  ( 83.20384757729335945, -33.24240381056766580, -96.99999999999998579 ) ) ;
#13499=VERTEX_POINT ( 'NONE', #12333 ) ;
#13501=CARTESIAN_POINT ( 'NONE',  ( -82.39999999999999147, -34.83749999999999858, -96.53589838486223584 ) ) ;
#13503=CARTESIAN_POINT ( 'NONE',  ( -80.90000000000000568, -32.79374999877096997, 97.40192378864668399 ) ) ;
#13504=CARTESIAN_POINT ( 'NONE',  ( 80.90000000000000568, -31.20000000000000284, 97.40192378864668399 ) ) ;
#13505=CARTESIAN_POINT ( 'NONE',  ( -84.29633955546280788, -32.00000000000001421, -97.97042480180299151 ) ) ;
#13509=CARTESIAN_POINT ( 'NONE',  ( 83.20384757729338787, -32.10134618820330132, 97.00000000000000000 ) ) ;
#13510=CARTESIAN_POINT ( 'NONE',  ( -80.90000000000000568, -32.04374999877096997, -97.40192378864668399 ) ) ;
#13511=CARTESIAN_POINT ( 'NONE',  ( 79.64356964374999848, -31.26562499938548356, -99.99999999999998579 ) ) ;
#13514=PLANE ( 'NONE',  #18499 ) ;
#13515=CARTESIAN_POINT ( 'NONE',  ( 82.39999999999999147, -32.50312499938548427, -96.81714838363319586 ) ) ;
#13519=CARTESIAN_POINT ( 'NONE',  ( -83.90000000000000568, -30.97500000000000142, 97.40192378864668399 ) ) ;
#13520=VERTEX_POINT ( 'NONE', #1977 ) ;
#13521=CARTESIAN_POINT ( 'NONE',  ( -85.16220480609818821, -34.99999999999999289, 98.91314642829009074 ) ) ;
#13523=DIRECTION ( 'NONE',  ( -0.000000000000000000, -0.000000000000000000, -1.000000000000000000 ) ) ;
#13525=CARTESIAN_POINT ( 'NONE',  ( -79.58826230849687988, -32.00000000000094502, 98.95399275615287138 ) ) ;
#13526=CARTESIAN_POINT ( 'NONE',  ( -81.59615242270662350, -32.06115380933863435, 103.0000000000000000 ) ) ;
#13528=CARTESIAN_POINT ( 'NONE',  ( 79.64356964374999848, -34.97812499938548569, 99.99999999999998579 ) ) ;
#13529=EDGE_CURVE ( 'NONE', #17007, #800, #9219, .T. ) ;
#13532=CARTESIAN_POINT ( 'NONE',  ( -82.39999999999999147, -31.49062499938548854, -96.81714838363319586 ) ) ;
#13534=CARTESIAN_POINT ( 'NONE',  ( 81.02178482187500208, -31.00312499938548783, 97.61286128772489690 ) ) ;
#13537=CARTESIAN_POINT ( 'NONE',  ( -81.02178482187500208, -30.55312499938548854, 102.3871387122750889 ) ) ;
#13539=ORIENTED_EDGE ( 'NONE', *, *, #8289, .F. ) ;
#13540=CARTESIAN_POINT ( 'NONE',  ( -85.40000000000000568, -30.00000000000000355, -99.99999999999998579 ) ) ;
#13543=EDGE_CURVE ( 'NONE', #779, #3049, #2099, .T. ) ;
#13545=CARTESIAN_POINT ( 'NONE',  ( -79.64356964375001269, -32.24062499938548854, -101.5914258081833879 ) ) ;
#13547=DIRECTION ( 'NONE',  ( 1.000000000000000000, 0.000000000000000000, 0.000000000000000000 ) ) ;
#13551=CARTESIAN_POINT ( 'NONE',  ( -79.64356964374998427, -34.45312499938548711, -98.40857419181659793 ) ) ;
#13552=CARTESIAN_POINT ( 'NONE',  ( 85.15643035625001289, -33.25312499938548427, 98.40857419181659793 ) ) ;
#13554=CARTESIAN_POINT ( 'NONE',  ( 83.90000000000000568, -33.16874999877096286, -97.40192378864668399 ) ) ;
#13572=CARTESIAN_POINT ( 'NONE',  ( -85.15643035624999868, -34.26562499938548711, 101.5914258081833879 ) ) ;
#13574=EDGE_CURVE ( 'NONE', #17308, #6543, #8131, .T. ) ;
#13578=FACE_OUTER_BOUND ( 'NONE', #17321, .T. ) ;
#13580=CARTESIAN_POINT ( 'NONE',  ( -80.85389467647067363, -35.00000000000000000, -102.4890844034573831 ) ) ;
#13582=ORIENTED_EDGE ( 'NONE', *, *, #8517, .T. ) ;
#13583=CARTESIAN_POINT ( 'NONE',  ( -81.02178482187500208, -32.99062499938548854, -102.3871387122750889 ) ) ;
#13590=ORIENTED_EDGE ( 'NONE', *, *, #17160, .T. ) ;
#13592=CARTESIAN_POINT ( 'NONE',  ( -82.86160995759654213, -32.00000000000002132, 102.8104067583495578 ) ) ;
#13594=CARTESIAN_POINT ( 'NONE',  ( -83.90000000000000568, -32.56874999877096855, 102.5980762113533018 ) ) ;
#13595=CARTESIAN_POINT ( 'NONE',  ( 79.39999999999999147, -31.61250000000000071, 98.26794919243113213 ) ) ;
#13596=CARTESIAN_POINT ( 'NONE',  ( 82.39999999999999147, -33.43124999877097281, 96.99999999999998579 ) ) ;
#13598=CIRCLE ( 'NONE', #2680, 2.199999999999993516 ) ;
#13600=CARTESIAN_POINT ( 'NONE',  ( 79.79868554276785630, -32.00000000000000000, -98.52838665788617334 ) ) ;
#13601=CARTESIAN_POINT ( 'NONE',  ( 81.02178482187500208, -33.59062499938548285, -102.3871387122750889 ) ) ;
#13604=CARTESIAN_POINT ( 'NONE',  ( 83.90000000000000568, -34.87500000000000000, -102.5980762113533018 ) ) ;
#13605=CARTESIAN_POINT ( 'NONE',  ( 79.64356964375001269, -33.55312499938548854, -101.5914258081833879 ) ) ;
#13607=DIRECTION ( 'NONE',  ( -0.000000000000000000, -1.000000000000000000, -0.000000000000000000 ) ) ;
#13610=CARTESIAN_POINT ( 'NONE',  ( -79.39999999999999147, -30.67500000000000071, 99.99999999999998579 ) ) ;
#13613=( BOUNDED_CURVE ( )  B_SPLINE_CURVE ( 2, ( #15426, #6351, #6641, #18556, #14054, #5081, #12303, #688, #4887 ),
 .UNSPECIFIED., .F., .F. ) 
 B_SPLINE_CURVE_WITH_KNOTS ( ( 3, 2, 2, 2, 3 ),
 ( 0.3958333333333334259, 0.4027777777777777901, 0.4166666666666666852, 0.4305555555555555802, 0.4375000000000000555 ),
 .UNSPECIFIED. ) 
 CURVE ( )  GEOMETRIC_REPRESENTATION_ITEM ( )  RATIONAL_B_SPLINE_CURVE ( ( 0.9330127018922192983, 0.9330127018922200755, 1.000000000000000000, 0.8660254037844387076, 1.000000000000000000, 0.8660254037844387076, 1.000000000000000000, 0.9330127018922187432, 0.9330127018922192983 ) ) 
 REPRESENTATION_ITEM ( '' )  );
#13622=CARTESIAN_POINT ( 'NONE',  ( 85.15643035624999868, -35.16562499938547859, 98.40857419181659793 ) ) ;
#13623=CARTESIAN_POINT ( 'NONE',  ( -85.40000000000000568, -32.73750000000000426, 98.26794919243111792 ) ) ;
#13625=CARTESIAN_POINT ( 'NONE',  ( -81.02178482187500208, -32.20312499938548711, 97.61286128772489690 ) ) ;
#13626=CARTESIAN_POINT ( 'NONE',  ( -82.39999999999999147, -33.96562499938548285, -103.1828516163667899 ) ) ;
#13627=ORIENTED_EDGE ( 'NONE', *, *, #16494, .T. ) ;
#13628=CARTESIAN_POINT ( 'NONE',  ( 81.02178482187500208, -31.30312499938548498, 102.3871387122750889 ) ) ;
#13632=CARTESIAN_POINT ( 'NONE',  ( -82.39999999999999147, -32.61562499938548854, 96.81714838363319586 ) ) ;
#13635=CARTESIAN_POINT ( 'NONE',  ( -85.40000000000000568, -31.80000000000000071, -99.99999999999998579 ) ) ;
#13636=AXIS2_PLACEMENT_3D ( 'NONE', #18448, #483, #3688 ) ;
#13637=EDGE_CURVE ( 'NONE', #5607, #4516, #11350, .T. ) ;
#13639=EDGE_CURVE ( 'NONE', #893, #15550, #1369, .T. ) ;
#13640=CARTESIAN_POINT ( 'NONE',  ( 83.60689295392862164, -35.00000000000000000, 102.7535308243271288 ) ) ;
#13641=DIRECTION ( 'NONE',  ( -0.000000000000000000, -0.000000000000000000, -1.000000000000000000 ) ) ;
#13642=CARTESIAN_POINT ( 'NONE',  ( -79.64356964375001269, -32.31562499938548427, -98.40857419181659793 ) ) ;
#13647=ORIENTED_EDGE ( 'NONE', *, *, #13574, .T. ) ;
#13649=CARTESIAN_POINT ( 'NONE',  ( -83.90000000000000568, -33.46874999877096712, 102.5980762113533018 ) ) ;
#13650=CARTESIAN_POINT ( 'NONE',  ( 85.15643035625001289, -34.15312499938548285, 98.40857419181659793 ) ) ;
#13652=CARTESIAN_POINT ( 'NONE',  ( -82.40000000000001990, -33.88124999877096855, -97.00000000000000000 ) ) ;
#13653=CARTESIAN_POINT ( 'NONE',  ( 80.90000000000000568, -34.29374999877096997, -102.5980762113533018 ) ) ;
#13656=EDGE_CURVE ( 'NONE', #11864, #2988, #13100, .T. ) ;
#13661=ADVANCED_FACE ( 'NONE', ( #5778 ), #8604, .F. ) ;
#13666=ORIENTED_EDGE ( 'NONE', *, *, #8793, .F. ) ;
#13667=VERTEX_POINT ( 'NONE', #6960 ) ;
#13668=CARTESIAN_POINT ( 'NONE',  ( -81.02178482187500208, -30.29062499938548569, -102.3871387122750889 ) ) ;
#13670=CARTESIAN_POINT ( 'NONE',  ( -80.90000000000000568, -34.80000000000000426, 102.5980762113533018 ) ) ;
#13672=FACE_OUTER_BOUND ( 'NONE', #9123, .T. ) ;
#13674=AXIS2_PLACEMENT_3D ( 'NONE', #3685, #18928, #15990 ) ;
#13678=CARTESIAN_POINT ( 'NONE',  ( -96.99999999999998579, -29.80000000000000426, -150.0000000000000000 ) ) ;
#13679=CARTESIAN_POINT ( 'NONE',  ( -80.90000000000000568, -33.75000000000000000, 97.40192378864668399 ) ) ;
#13680=PLANE ( 'NONE',  #10556 ) ;
#13684=CARTESIAN_POINT ( 'NONE',  ( -81.02178482187500208, -33.44062499938548427, -102.3871387122750889 ) ) ;
#13693=B_SPLINE_CURVE_WITH_KNOTS ( 'NONE', 3,
 ( #470, #10618, #376, #8702, #13640, #10713, #18244, #12374, #12180, #7329 ),
 .UNSPECIFIED., .F., .F.,
 ( 4, 2, 2, 2, 4 ),
 ( 0.3612006186103786654, 0.3925526867148934063, 0.4239047548194081472, 0.4552568229239228881, 0.4866088910284376290 ),
 .UNSPECIFIED. ) ;
#13694=FACE_OUTER_BOUND ( 'NONE', #18347, .T. ) ;
#13695=ORIENTED_EDGE ( 'NONE', *, *, #1401, .T. ) ;
#13698=CARTESIAN_POINT ( 'NONE',  ( 83.90000000000000568, -30.97500000000000142, -97.40192378864668399 ) ) ;
#13699=CARTESIAN_POINT ( 'NONE',  ( -83.90000000000000568, -33.16874999877096286, 97.40192378864668399 ) ) ;
#13700=CARTESIAN_POINT ( 'NONE',  ( 85.40000000000000568, -31.83750000000000568, 101.7320508075688679 ) ) ;
#13702=CARTESIAN_POINT ( 'NONE',  ( -82.39999999999999147, -32.81250000000000000, 97.00000000000000000 ) ) ;
#13704=CARTESIAN_POINT ( 'NONE',  ( 79.64356964374998427, -34.11562499938548854, -101.5914258081833879 ) ) ;
#13705=CYLINDRICAL_SURFACE ( 'NONE', #1523, 3.000000000000002665 ) ;
#13706=CARTESIAN_POINT ( 'NONE',  ( 81.02178482187500208, -33.14062499938548711, -102.3871387122750889 ) ) ;
#13709=CARTESIAN_POINT ( 'NONE',  ( 82.39999999999999147, -32.27812499938548285, -103.1828516163667899 ) ) ;
#13710=CARTESIAN_POINT ( 'NONE',  ( 85.15643035624999868, -33.70312499938548711, -101.5914258081833879 ) ) ;
#13714=CARTESIAN_POINT ( 'NONE',  ( -85.40000000000000568, -30.90000000000000213, 99.99999999999998579 ) ) ;
#13718=CARTESIAN_POINT ( 'NONE',  ( 81.02178482187500208, -30.74062499938548498, 102.3871387122750889 ) ) ;
#13719=CARTESIAN_POINT ( 'NONE',  ( 85.40000000000000568, -32.64374999877097139, -99.99999999999998579 ) ) ;
#13722=CARTESIAN_POINT ( 'NONE',  ( 79.64356964375001269, -30.77812499938548285, 101.5914258081833879 ) ) ;
#13723=CARTESIAN_POINT ( 'NONE',  ( 79.64356964375001269, -32.24062499938548854, -98.40857419181659793 ) ) ;
#13725=CARTESIAN_POINT ( 'NONE',  ( -84.56803305035340657, -32.00000000000000000, -98.28830862702052684 ) ) ;
#13726=CARTESIAN_POINT ( 'NONE',  ( -79.64356964375001269, -33.59062499938548285, -101.5914258081833879 ) ) ;
#13728=VERTEX_POINT ( 'NONE', #7048 ) ;
#13729=CARTESIAN_POINT ( 'NONE',  ( 83.90000000000000568, -34.81874999877096855, 97.40192378864668399 ) ) ;
#13733=CARTESIAN_POINT ( 'NONE',  ( -82.39999999999999147, -32.84062499938548996, 103.1828516163667899 ) ) ;
#13736=CARTESIAN_POINT ( 'NONE',  ( -83.25523545990762386, -35.19352049914630953, -103.2690260512239604 ) ) ;
#13737=CARTESIAN_POINT ( 'NONE',  ( 83.33080762004576059, -35.05289549976084373, -96.44210921874548603 ) ) ;
#13738=CARTESIAN_POINT ( 'NONE',  ( 81.59615242270665192, -33.67634618820330417, 103.0000000000000000 ) ) ;
#13739=CARTESIAN_POINT ( 'NONE',  ( 82.40000000000000568, -33.71249999999998437, 102.9999999999999858 ) ) ;
#13745=CARTESIAN_POINT ( 'NONE',  ( -83.20384757729335945, -33.63615380933863008, 96.99999999999998579 ) ) ;
#13746=CARTESIAN_POINT ( 'NONE',  ( 85.15643035625001289, -32.42812499938548854, 101.5914258081833879 ) ) ;
#13749=CARTESIAN_POINT ( 'NONE',  ( 82.39999999999999147, -34.10624999877096997, -96.53589838486223584 ) ) ;
#13757=CARTESIAN_POINT ( 'NONE',  ( -81.59615242270662350, -32.83259618943233704, -102.9999999999999716 ) ) ;
#13760=CARTESIAN_POINT ( 'NONE',  ( -82.14831453752226764, -31.99999999999999289, 97.14155664245926403 ) ) ;
#13761=CARTESIAN_POINT ( 'NONE',  ( -79.39999999999999147, -33.73124999877096997, -101.7320508075688963 ) ) ;
#13765=CARTESIAN_POINT ( 'NONE',  ( 85.15643035625001289, -32.05312499938548854, 99.99999999999998579 ) ) ;
#13766=CARTESIAN_POINT ( 'NONE',  ( -85.40000000000000568, -33.58124999877097139, -101.7320508075688679 ) ) ;
#13767=ADVANCED_FACE ( 'NONE', ( #8082 ), #7979, .F. ) ;
#13772=CARTESIAN_POINT ( 'NONE',  ( -82.40000000000000568, -33.93750000000000711, 102.9999999999999858 ) ) ;
#13773=CARTESIAN_POINT ( 'NONE',  ( 79.39999999999999147, -34.72500000000000142, -99.99999999999998579 ) ) ;
#13774=DIRECTION ( 'NONE',  ( 0.000000000000000000, 0.000000000000000000, 1.000000000000000000 ) ) ;
#13779=CARTESIAN_POINT ( 'NONE',  ( -83.77821517812500929, -32.46562499938548285, -102.3871387122750889 ) ) ;
#13781=ORIENTED_EDGE ( 'NONE', *, *, #5603, .T. ) ;
#13785=ORIENTED_EDGE ( 'NONE', *, *, #7470, .F. ) ;
#13789=ORIENTED_EDGE ( 'NONE', *, *, #16365, .T. ) ;
#13790=CARTESIAN_POINT ( 'NONE',  ( 82.39999999999999147, -30.11250000000000426, -96.53589838486223584 ) ) ;
#13791=CARTESIAN_POINT ( 'NONE',  ( -83.90000000000000568, -33.46874999877096712, 102.5980762113533018 ) ) ;
#13792=CARTESIAN_POINT ( 'NONE',  ( -83.74167325096722436, -32.00000000000001421, -97.53412486788926117 ) ) ;
#13794=CARTESIAN_POINT ( 'NONE',  ( 85.15643035625001289, -33.89062499938548711, -98.40857419181659793 ) ) ;
#13795=CARTESIAN_POINT ( 'NONE',  ( 83.92761994968586237, -31.99999999999999289, -97.66884955413871694 ) ) ;
#13797=CARTESIAN_POINT ( 'NONE',  ( 85.15643035625001289, -34.64062499938548711, -99.99999999999998579 ) ) ;
#13800=CARTESIAN_POINT ( 'NONE',  ( -82.39999999999999147, -34.61250000000000426, 96.53589838486223584 ) ) ;
#13801=CARTESIAN_POINT ( 'NONE',  ( 82.40000000000000568, -33.43124999877096570, -102.9999999999999858 ) ) ;
#13806=CARTESIAN_POINT ( 'NONE',  ( -82.39999999999999147, -33.03750000000000142, 103.4641016151377499 ) ) ;
#13807=VERTEX_POINT ( 'NONE', #3394 ) ;
#13812=CARTESIAN_POINT ( 'NONE',  ( 85.12124608221321864, -32.00000000000000000, -99.52644304242026863 ) ) ;
#13814=CARTESIAN_POINT ( 'NONE',  ( 83.77821517812500929, -34.22812499938549280, 97.61286128772489690 ) ) ;
#13815=CARTESIAN_POINT ( 'NONE',  ( 82.39999999999999147, -30.59062499938548640, -103.1828516163667899 ) ) ;
#13817=CARTESIAN_POINT ( 'NONE',  ( -81.02178482187500208, -32.09062499938548285, 97.61286128772489690 ) ) ;
#13818=CARTESIAN_POINT ( 'NONE',  ( -82.39999999999999147, -34.19062499938548427, -96.81714838363319586 ) ) ;
#13820=ORIENTED_EDGE ( 'NONE', *, *, #16453, .T. ) ;
#13821=CARTESIAN_POINT ( 'NONE',  ( 83.77821517812500929, -33.02812499938548285, 102.3871387122750889 ) ) ;
#13824=CARTESIAN_POINT ( 'NONE',  ( -79.64356964375001269, -33.59062499938548285, 98.40857419181659793 ) ) ;
#13825=DIRECTION ( 'NONE',  ( -0.000000000000000000, -1.000000000000000000, -0.000000000000000000 ) ) ;
#13827=CARTESIAN_POINT ( 'NONE',  ( -82.39999999999999147, -30.78750000000000497, -96.53589838486223584 ) ) ;
#13828=CARTESIAN_POINT ( 'NONE',  ( 85.40000000000000568, -34.95000000000000284, -99.99999999999998579 ) ) ;
#13829=CARTESIAN_POINT ( 'NONE',  ( -83.32052461991715120, -34.98323688327303671, -102.9326364780328760 ) ) ;
#13830=FACE_OUTER_BOUND ( 'NONE', #2412, .T. ) ;
#13836=CARTESIAN_POINT ( 'NONE',  ( 85.40000000000000568, -34.53750000000000142, -98.26794919243111792 ) ) ;
#13838=CARTESIAN_POINT ( 'NONE',  ( 82.40000000000001990, -32.08124999877097139, -103.0000000000000000 ) ) ;
#13839=FACE_OUTER_BOUND ( 'NONE', #4719, .T. ) ;
#13840=CARTESIAN_POINT ( 'NONE',  ( 85.15643035624999868, -31.64062499938548356, -98.40857419181659793 ) ) ;
#13849=ORIENTED_EDGE ( 'NONE', *, *, #14158, .F. ) ;
#13850=ORIENTED_EDGE ( 'NONE', *, *, #4155, .T. ) ;
#13852=CARTESIAN_POINT ( 'NONE',  ( -79.39999999999999147, -33.76874999877097139, -99.99999999999998579 ) ) ;
#13856=CARTESIAN_POINT ( 'NONE',  ( -80.90000000000000568, -33.24374999877097281, -102.5980762113533018 ) ) ;
#13862=CYLINDRICAL_SURFACE ( 'NONE', #10072, 3.000000000000002665 ) ;
#13865=ORIENTED_EDGE ( 'NONE', *, *, #18798, .T. ) ;
#13867=CARTESIAN_POINT ( 'NONE',  ( 94.79999999999995453, -5.200000000000000178, -150.0000000000000000 ) ) ;
#13868=CARTESIAN_POINT ( 'NONE',  ( -69.99999999999998579, -32.00000000000000000, 150.0000000000000000 ) ) ;
#13869=ORIENTED_EDGE ( 'NONE', *, *, #14250, .F. ) ;
#13873=CARTESIAN_POINT ( 'NONE',  ( 85.40000000000000568, -33.11250000000000426, -101.7320508075688821 ) ) ;
#13874=ORIENTED_EDGE ( 'NONE', *, *, #496, .F. ) ;
#13881=CARTESIAN_POINT ( 'NONE',  ( 83.90000000000000568, -31.42500000000000071, -97.40192378864668399 ) ) ;
#13884=CARTESIAN_POINT ( 'NONE',  ( -80.90000000000000568, -33.39374999877097139, 102.5980762113533018 ) ) ;
#13887=CARTESIAN_POINT ( 'NONE',  ( 81.02178482187500208, -33.55312499938548854, -97.61286128772489690 ) ) ;
#13888=CARTESIAN_POINT ( 'NONE',  ( 84.11496519894586754, -32.00000000000000000, -97.81539907810424950 ) ) ;
#13889=CARTESIAN_POINT ( 'NONE',  ( -85.15643035624999868, -33.70312499938548711, 101.5914258081833879 ) ) ;
#13890=VECTOR ( 'NONE', #5148, 1000.000000000000000 ) ;
#13891=CARTESIAN_POINT ( 'NONE',  ( 79.64356964375001269, -34.37812499938548427, -98.40857419181659793 ) ) ;
#13892=ORIENTED_EDGE ( 'NONE', *, *, #8892, .F. ) ;
#13900=EDGE_CURVE ( 'NONE', #13349, #11282, #16684, .T. ) ;
#13901=CARTESIAN_POINT ( 'NONE',  ( -85.40000000000000568, -33.14999999999999858, 99.99999999999998579 ) ) ;
#13902=ORIENTED_EDGE ( 'NONE', *, *, #1479, .F. ) ;
#13905=CARTESIAN_POINT ( 'NONE',  ( 80.80861089413670584, -34.99999999999999289, 97.72105564972112290 ) ) ;
#13906=CARTESIAN_POINT ( 'NONE',  ( 85.15643035625001289, -32.39062499938548711, 99.99999999999998579 ) ) ;
#13910=CARTESIAN_POINT ( 'NONE',  ( -81.02178482187500208, -32.35312499938548569, -97.61286128772489690 ) ) ;
#13911=CARTESIAN_POINT ( 'NONE',  ( 82.39999999999999147, -33.96562499938548285, 103.1828516163667899 ) ) ;
#13913=CARTESIAN_POINT ( 'NONE',  ( 82.39999999999999147, -31.94062499938548427, -103.1828516163667899 ) ) ;
#13915=CARTESIAN_POINT ( 'NONE',  ( -81.02178482187500208, -34.00312499938548427, 97.61286128772489690 ) ) ;
#13916=CARTESIAN_POINT ( 'NONE',  ( -83.77821517812500929, -33.32812499938548711, -97.61286128772489690 ) ) ;
#13918=ORIENTED_EDGE ( 'NONE', *, *, #1592, .F. ) ;
#13919=CARTESIAN_POINT ( 'NONE',  ( 83.77821517812500929, -33.92812499938548854, 102.3871387122750889 ) ) ;
#13921=CARTESIAN_POINT ( 'NONE',  ( -79.64356964375001269, -30.32812499938548711, 98.40857419181659793 ) ) ;
#13922=CARTESIAN_POINT ( 'NONE',  ( -85.15643035625001289, -34.30312499938548854, 99.99999999999998579 ) ) ;
#13925=ORIENTED_EDGE ( 'NONE', *, *, #11902, .F. ) ;
#13927=CARTESIAN_POINT ( 'NONE',  ( -83.90000000000000568, -33.22500000000000142, -102.5980762113533018 ) ) ;
#13933=ORIENTED_EDGE ( 'NONE', *, *, #15583, .T. ) ;
#13938=DIRECTION ( 'NONE',  ( -1.000000000000000000, 0.000000000000000000, 0.000000000000000000 ) ) ;
#13940=AXIS2_PLACEMENT_3D ( 'NONE', #8518, #9800, #4036 ) ;
#13941=CARTESIAN_POINT ( 'NONE',  ( 85.15643035624999868, -30.29062499938548925, -98.40857419181659793 ) ) ;
#13944=CARTESIAN_POINT ( 'NONE',  ( 82.39999999999999147, -30.50624999877097210, 103.4641016151377499 ) ) ;
#13952=ORIENTED_EDGE ( 'NONE', *, *, #18321, .F. ) ;
#13953=CARTESIAN_POINT ( 'NONE',  ( -82.39999999999999147, -31.82812499938548356, -96.81714838363319586 ) ) ;
#13956=ORIENTED_EDGE ( 'NONE', *, *, #8958, .T. ) ;
#13958=CARTESIAN_POINT ( 'NONE',  ( -85.40000000000000568, -34.93124999877096570, -101.7320508075688679 ) ) ;
#13964=( BOUNDED_SURFACE ( )  B_SPLINE_SURFACE ( 1, 2, ( 
 ( #14706, #75, #1432, #7196, #1537, #8850, #16479, #7486, #170, #10609, #8942, #15008, #13441, #4365, #13245, #17758, #19217, #2802, #17655, #3083, #11975, #5834, #18049, #14806, #13145, #6121, #7387, #1626, #10228, #14909, #16195, #13348, #17943, #13532, #11786, #10325, #16284, #7581, #19119, #11879, #4554, #2894, #8754, #18630, #5932, #4659, #16576, #17847, #1343, #3176, #10511, #7290, #4459, #10414, #16377, #2986, #9136, #5738, #11687, #3566, #15192, #11083, #1810, #10701, #16758, #3374, #3466, #18423, #654, #10796, #12364, #2103, #9326, #5044, #7773, #6602, #12270, #16667, #461, #10893, #4758, #9424, #13916, #9525, #1905, #3665, #3272, #6512, #15491, #13726, #18234, #6409, #15392, #367, #554, #14018, #12170, #4851, #15290, #13626, #5138, #8063, #9629, #6316, #7867, #13818, #12550, #1716, #17053, #7670, #12457, #18332, #4951, #18521, #269, #16861, #2003, #7962, #6223, #10985, #16954, #18138, #9228, #8806, #7342, #8514, #13295, #17607, #10282, #5887, #11739, #5785, #2753, #14763, #15951 ),
 ( #14465, #14663, #17706, #16143, #16244, #1298, #19271, #14562, #1097, #4220, #10178, #8710, #7157, #7056, #2199, #2552, #13015, #7245, #4321, #11647, #19173, #2646, #747, #2851, #11836, #1393, #17804, #5238, #18985, #4414, #16044, #15591, #5608, #8612, #11552, #8161, #6702, #11187, #14110, #18620, #19076, #13201, #12646, #9722, #17150, #3757, #17515, #4126, #13107, #10088, #1199, #5694, #6275, #17902, #3229, #4612, #18285, #4711, #12027, #328, #10656, #3324, #13779, #12130, #18190, #16623, #7534, #16431, #1584, #3040, #9001, #10371, #10464, #14961, #9188, #1768, #13583, #6081, #15150, #13398, #1865, #16335, #4509, #10567, #224, #13490, #7728, #12220, #13684, #4811, #131, #7440, #10752, #18100, #16716, #9284, #15252, #2944, #7824, #419, #6367, #18000, #16531, #12319, #8897, #14860, #6178, #5980, #1487, #30, #11930, #3132, #9091, #15054, #1678, #7629, #3615, #9577, #6559, #3520, #13972, #1959, #14257, #8115, #7918, #610, #15641, #15441, #895, #3805, #15343, #17200, #6658, #9478, #15544 ) ),
 .UNSPECIFIED., .F., .F., .F. ) 
 B_SPLINE_SURFACE_WITH_KNOTS ( ( 2, 2 ),
 ( 3, 2, 2, 2, 2, 2, 2, 2, 2, 2, 2, 2, 2, 2, 2, 2, 2, 2, 2, 2, 2, 2, 2, 2, 2, 2, 2, 2, 2, 2, 2, 2, 2, 2, 2, 2, 2, 2, 2, 2, 2, 2, 2, 2, 2, 2, 2, 2, 2, 2, 2, 2, 2, 2, 2, 2, 2, 2, 2, 2, 2, 2, 2, 2, 2, 2, 2, 3 ),
 ( 0.000000000000000000, 1.000000000000000000 ),
 ( 0.000000000000000000, 0.01388888888888888812, 0.02777777777777777624, 0.04166666666666666435, 0.05555555555555555247, 0.06944444444444444753, 0.08333333333333332871, 0.09722222222222222376, 0.1111111111111111049, 0.1250000000000000000, 0.1388888888888888951, 0.1527777777777777901, 0.1666666666666666574, 0.1805555555555555525, 0.1944444444444444475, 0.2083333333333333426, 0.2222222222222222099, 0.2361111111111111049, 0.2500000000000000000, 0.2638888888888888951, 0.2777777777777777901, 0.2916666666666666852, 0.3055555555555555802, 0.3194444444444444198, 0.3333333333333333148, 0.3472222222222222099, 0.3611111111111111049, 0.3750000000000000000, 0.3888888888888888951, 0.4027777777777777901, 0.4166666666666666852, 0.4305555555555555802, 0.4444444444444444198, 0.4583333333333333148, 0.4722222222222222099, 0.4861111111111111049, 0.5000000000000000000, 0.5138888888888888395, 0.5277777777777777901, 0.5416666666666666297, 0.5555555555555555802, 0.5694444444444444198, 0.5833333333333333703, 0.5972222222222222099, 0.6111111111111111605, 0.6250000000000000000, 0.6388888888888888395, 0.6527777777777777901, 0.6666666666666666297, 0.6805555555555555802, 0.6944444444444444198, 0.7083333333333333703, 0.7222222222222222099, 0.7361111111111111605, 0.7500000000000000000, 0.7638888888888888395, 0.7777777777777777901, 0.7916666666666666297, 0.8055555555555555802, 0.8194444444444444198, 0.8333333333333333703, 0.8472222222222222099, 0.8611111111111111605, 0.8750000000000000000, 0.8888888888888888395, 0.9027777777777777901, 0.9166666666666666297, 0.9258785565094813652 ),
 .UNSPECIFIED. ) 
 GEOMETRIC_REPRESENTATION_ITEM ( )  RATIONAL_B_SPLINE_SURFACE ( (
 ( 1.000000000000000000, 0.8660254037844387076, 1.000000000000000000, 0.8660254037844387076, 1.000000000000000000, 0.8660254037844387076, 1.000000000000000000, 0.8660254037844387076, 1.000000000000000000, 0.8660254037844387076, 1.000000000000000000, 0.8660254037844387076, 1.000000000000000000, 0.8660254037844387076, 1.000000000000000000, 0.8660254037844387076, 1.000000000000000000, 0.8660254037844387076, 1.000000000000000000, 0.8660254037844387076, 1.000000000000000000, 0.8660254037844387076, 1.000000000000000000, 0.8660254037844387076, 1.000000000000000000, 0.8660254037844387076, 1.000000000000000000, 0.8660254037844387076, 1.000000000000000000, 0.8660254037844387076, 1.000000000000000000, 0.8660254037844387076, 1.000000000000000000, 0.8660254037844387076, 1.000000000000000000, 0.8660254037844387076, 1.000000000000000000, 0.8660254037844387076, 1.000000000000000000, 0.8660254037844387076, 1.000000000000000000, 0.8660254037844387076, 1.000000000000000000, 0.8660254037844387076, 1.000000000000000000, 0.8660254037844387076, 1.000000000000000000, 0.8660254037844387076, 1.000000000000000000, 0.8660254037844387076, 1.000000000000000000, 0.8660254037844387076, 1.000000000000000000, 0.8660254037844387076, 1.000000000000000000, 0.8660254037844387076, 1.000000000000000000, 0.8660254037844387076, 1.000000000000000000, 0.8660254037844387076, 1.000000000000000000, 0.8660254037844387076, 1.000000000000000000, 0.8660254037844387076, 1.000000000000000000, 0.8660254037844387076, 1.000000000000000000, 0.8660254037844387076, 1.000000000000000000, 0.8660254037844387076, 1.000000000000000000, 0.8660254037844387076, 1.000000000000000000, 0.8660254037844387076, 1.000000000000000000, 0.8660254037844387076, 1.000000000000000000, 0.8660254037844387076, 1.000000000000000000, 0.8660254037844387076, 1.000000000000000000, 0.8660254037844387076, 1.000000000000000000, 0.8660254037844387076, 1.000000000000000000, 0.8660254037844387076, 1.000000000000000000, 0.8660254037844387076, 1.000000000000000000, 0.8660254037844387076, 1.000000000000000000, 0.8660254037844387076, 1.000000000000000000, 0.8660254037844387076, 1.000000000000000000, 0.8660254037844387076, 1.000000000000000000, 0.8660254037844387076, 1.000000000000000000, 0.8660254037844387076, 1.000000000000000000, 0.8660254037844387076, 1.000000000000000000, 0.8660254037844387076, 1.000000000000000000, 0.8660254037844387076, 1.000000000000000000, 0.8660254037844387076, 1.000000000000000000, 0.8660254037844387076, 1.000000000000000000, 0.8660254037844387076, 1.000000000000000000, 0.8660254037844387076, 1.000000000000000000, 0.8660254037844387076, 1.000000000000000000, 0.8660254037844387076, 1.000000000000000000, 0.8660254037844387076, 1.000000000000000000, 0.8660254037844387076, 1.000000000000000000, 0.8660254037844387076, 1.000000000000000000, 0.8660254037844387076, 1.000000000000000000, 0.8660254037844387076, 1.000000000000000000, 0.8660254037844387076, 1.000000000000000000, 0.8660254037844387076, 1.000000000000000000, 0.9111405360107203144, 0.9401542295229963209),
 ( 1.000000000000000000, 0.8660254037844387076, 1.000000000000000000, 0.8660254037844387076, 1.000000000000000000, 0.8660254037844387076, 1.000000000000000000, 0.8660254037844387076, 1.000000000000000000, 0.8660254037844387076, 1.000000000000000000, 0.8660254037844387076, 1.000000000000000000, 0.8660254037844387076, 1.000000000000000000, 0.8660254037844387076, 1.000000000000000000, 0.8660254037844387076, 1.000000000000000000, 0.8660254037844387076, 1.000000000000000000, 0.8660254037844387076, 1.000000000000000000, 0.8660254037844387076, 1.000000000000000000, 0.8660254037844387076, 1.000000000000000000, 0.8660254037844387076, 1.000000000000000000, 0.8660254037844387076, 1.000000000000000000, 0.8660254037844387076, 1.000000000000000000, 0.8660254037844387076, 1.000000000000000000, 0.8660254037844387076, 1.000000000000000000, 0.8660254037844387076, 1.000000000000000000, 0.8660254037844387076, 1.000000000000000000, 0.8660254037844387076, 1.000000000000000000, 0.8660254037844387076, 1.000000000000000000, 0.8660254037844387076, 1.000000000000000000, 0.8660254037844387076, 1.000000000000000000, 0.8660254037844387076, 1.000000000000000000, 0.8660254037844387076, 1.000000000000000000, 0.8660254037844387076, 1.000000000000000000, 0.8660254037844387076, 1.000000000000000000, 0.8660254037844387076, 1.000000000000000000, 0.8660254037844387076, 1.000000000000000000, 0.8660254037844387076, 1.000000000000000000, 0.8660254037844387076, 1.000000000000000000, 0.8660254037844387076, 1.000000000000000000, 0.8660254037844387076, 1.000000000000000000, 0.8660254037844387076, 1.000000000000000000, 0.8660254037844387076, 1.000000000000000000, 0.8660254037844387076, 1.000000000000000000, 0.8660254037844387076, 1.000000000000000000, 0.8660254037844387076, 1.000000000000000000, 0.8660254037844387076, 1.000000000000000000, 0.8660254037844387076, 1.000000000000000000, 0.8660254037844387076, 1.000000000000000000, 0.8660254037844387076, 1.000000000000000000, 0.8660254037844387076, 1.000000000000000000, 0.8660254037844387076, 1.000000000000000000, 0.8660254037844387076, 1.000000000000000000, 0.8660254037844387076, 1.000000000000000000, 0.8660254037844387076, 1.000000000000000000, 0.8660254037844387076, 1.000000000000000000, 0.8660254037844387076, 1.000000000000000000, 0.8660254037844387076, 1.000000000000000000, 0.8660254037844387076, 1.000000000000000000, 0.8660254037844387076, 1.000000000000000000, 0.8660254037844387076, 1.000000000000000000, 0.8660254037844387076, 1.000000000000000000, 0.8660254037844387076, 1.000000000000000000, 0.8660254037844387076, 1.000000000000000000, 0.8660254037844387076, 1.000000000000000000, 0.8660254037844387076, 1.000000000000000000, 0.8660254037844387076, 1.000000000000000000, 0.8660254037844387076, 1.000000000000000000, 0.8660254037844387076, 1.000000000000000000, 0.8660254037844387076, 1.000000000000000000, 0.8660254037844387076, 1.000000000000000000, 0.8660254037844387076, 1.000000000000000000, 0.8660254037844387076, 1.000000000000000000, 0.9111405360107203144, 0.9401542295229963209) ) ) 
 REPRESENTATION_ITEM ( '' )  SURFACE ( )  );
#13967=DIRECTION ( 'NONE',  ( 1.000000000000000000, 5.337610695313256118E-15, 0.000000000000000000 ) ) ;
#13969=ORIENTED_EDGE ( 'NONE', *, *, #11532, .T. ) ;
#13972=CARTESIAN_POINT ( 'NONE',  ( -85.15643035625001289, -34.64062499938548711, -99.99999999999998579 ) ) ;
#13975=FACE_OUTER_BOUND ( 'NONE', #6410, .T. ) ;
#13977=EDGE_LOOP ( 'NONE', ( #181, #8090, #14135, #4161 ) ) ;
#13980=AXIS2_PLACEMENT_3D ( 'NONE', #1005, #4027, #5689 ) ;
#13981=ORIENTED_EDGE ( 'NONE', *, *, #17977, .F. ) ;
#13982=ORIENTED_EDGE ( 'NONE', *, *, #14141, .F. ) ;
#13984=CARTESIAN_POINT ( 'NONE',  ( 80.90000000000000568, -31.50000000000000000, -97.40192378864668399 ) ) ;
#13986=CARTESIAN_POINT ( 'NONE',  ( -85.40000000000000568, -35.34374999877096712, 99.99999999999998579 ) ) ;
#13989=CARTESIAN_POINT ( 'NONE',  ( 82.39999999999999147, -33.06562499938548427, -96.81714838363319586 ) ) ;
#13991=CARTESIAN_POINT ( 'NONE',  ( -82.39999999999999147, -33.62812499938549138, 103.1828516163667899 ) ) ;
#13992=CARTESIAN_POINT ( 'NONE',  ( 85.15643035624999868, -33.70312499938548711, -101.5914258081833879 ) ) ;
#13994=CARTESIAN_POINT ( 'NONE',  ( -85.39999999999999147, -34.97364041986484295, 98.90809577818232867 ) ) ;
#13995=ADVANCED_FACE ( 'NONE', ( #15408 ), #9442, .F. ) ;
#13997=EDGE_CURVE ( 'NONE', #5564, #15718, #4945, .T. ) ;
#14002=CARTESIAN_POINT ( 'NONE',  ( -79.39999999999999147, -32.02500000000000568, 99.99999999999998579 ) ) ;
#14003=ORIENTED_EDGE ( 'NONE', *, *, #7428, .F. ) ;
#14005=CARTESIAN_POINT ( 'NONE',  ( 82.49978216248237572, -34.99999999999998579, 97.23961338447999481 ) ) ;
#14006=CARTESIAN_POINT ( 'NONE',  ( 83.77821517812500929, -33.36562499938548854, 102.3871387122750889 ) ) ;
#14008=EDGE_CURVE ( 'NONE', #18284, #15758, #635, .T. ) ;
#14009=CARTESIAN_POINT ( 'NONE',  ( 85.11512745526610502, -31.99999999999997868, -100.5952676699196218 ) ) ;
#14012=CARTESIAN_POINT ( 'NONE',  ( -79.64356964374998427, -32.31562499938548427, -98.40857419181659793 ) ) ;
#14013=CARTESIAN_POINT ( 'NONE',  ( 85.15643035624999868, -31.90312499938548285, 98.40857419181659793 ) ) ;
#14014=B_SPLINE_CURVE_WITH_KNOTS ( 'NONE', 3,
 ( #8739, #14693, #7277, #13231, #5821, #17745, #11769, #3455, #9412, #10880, #10783, #18034, #18317, #9124, #13521, #7565, #15087, #6496 ),
 .UNSPECIFIED., .F., .F.,
 ( 4, 2, 2, 2, 2, 2, 2, 2, 4 ),
 ( 0.000000000000000000, 0.0007089252359835931331, 0.001417850471967186266, 0.002126775707950779616, 0.002835700943934372532, 0.003544626179917965449, 0.004253551415901559232, 0.004962476651885152149, 0.005671401887868745065 ),
 .UNSPECIFIED. ) ;
#14015=CARTESIAN_POINT ( 'NONE',  ( 82.39999999999999147, -32.16562499938549280, -96.81714838363319586 ) ) ;
#14017=CARTESIAN_POINT ( 'NONE',  ( -85.15643035625001289, -32.99062499938548854, 98.40857419181659793 ) ) ;
#14018=CARTESIAN_POINT ( 'NONE',  ( -85.15643035624999868, -33.81562499938549138, -98.40857419181659793 ) ) ;
#14021=CARTESIAN_POINT ( 'NONE',  ( 82.39999999999999147, -32.61562499938548854, 103.1828516163667899 ) ) ;
#14023=CARTESIAN_POINT ( 'NONE',  ( -81.02178482187500208, -30.44062499938548783, 102.3871387122750889 ) ) ;
#14024=CARTESIAN_POINT ( 'NONE',  ( -81.02178482187500208, -33.55312499938548854, 97.61286128772489690 ) ) ;
#14025=DIRECTION ( 'NONE',  ( -0.000000000000000000, -1.000000000000000000, -0.000000000000000000 ) ) ;
#14026=ORIENTED_EDGE ( 'NONE', *, *, #13489, .F. ) ;
#14027=CARTESIAN_POINT ( 'NONE',  ( -85.40000000000000568, -34.05000000000000426, -99.99999999999998579 ) ) ;
#14037=CARTESIAN_POINT ( 'NONE',  ( -85.40000000000000568, -33.14999999999999858, 99.99999999999998579 ) ) ;
#14038=CARTESIAN_POINT ( 'NONE',  ( 83.20384757729337366, -34.35134618820330843, -103.0000000000000000 ) ) ;
#14039=CARTESIAN_POINT ( 'NONE',  ( 83.90000000000000568, -32.77499999999999858, -97.40192378864668399 ) ) ;
#14040=CARTESIAN_POINT ( 'NONE',  ( 82.39999999999999147, -31.04062499938548569, -103.1828516163667899 ) ) ;
#14042=( BOUNDED_CURVE ( )  B_SPLINE_CURVE ( 2, ( #16029, #8788, #10163, #4399, #17885, #2630, #17591 ),
 .UNSPECIFIED., .F., .F. ) 
 B_SPLINE_CURVE_WITH_KNOTS ( ( 3, 2, 2, 3 ),
 ( 0.3702305174533208065, 0.3750000000000000000, 0.3888888888888888951, 0.3958333333333334259 ),
 .UNSPECIFIED. ) 
 CURVE ( )  GEOMETRIC_REPRESENTATION_ITEM ( )  RATIONAL_B_SPLINE_CURVE ( ( 0.9395835397642970932, 0.9539927561189072147, 1.000000000000000000, 0.8660254037844387076, 1.000000000000000000, 0.9330127018922185211, 0.9330127018922192983 ) ) 
 REPRESENTATION_ITEM ( '' )  );
#14043=ORIENTED_EDGE ( 'NONE', *, *, #2420, .F. ) ;
#14044=CARTESIAN_POINT ( 'NONE',  ( 82.39999999999999147, -31.63124999877097210, 96.53589838486223584 ) ) ;
#14050=ORIENTED_EDGE ( 'NONE', *, *, #1497, .T. ) ;
#14053=CARTESIAN_POINT ( 'NONE',  ( -85.15643035625001289, -31.04062499938548569, -99.99999999999998579 ) ) ;
#14054=CARTESIAN_POINT ( 'NONE',  ( -85.40000000000000568, -32.25000000000000000, -99.99999999999998579 ) ) ;
#14056=CARTESIAN_POINT ( 'NONE',  ( 81.02178482187500208, -32.80312499938548854, 97.61286128772489690 ) ) ;
#14057=CARTESIAN_POINT ( 'NONE',  ( -79.39999999999999147, -34.21874999877096712, -99.99999999999998579 ) ) ;
#14058=CARTESIAN_POINT ( 'NONE',  ( 80.90000000000000568, -32.10000000000000142, 97.40192378864668399 ) ) ;
#14062=CARTESIAN_POINT ( 'NONE',  ( 82.40000000000000568, -30.00000000000000355, 99.99999999999998579 ) ) ;
#14064=CARTESIAN_POINT ( 'NONE',  ( 94.79999999999995453, -5.200000000000000178, 150.0000000000000000 ) ) ;
#14067=CARTESIAN_POINT ( 'NONE',  ( 81.02178482187500208, -33.14062499938548711, -102.3871387122750889 ) ) ;
#14070=CARTESIAN_POINT ( 'NONE',  ( -80.90000000000000568, -32.79374999877096997, -102.5980762113533018 ) ) ;
#14071=ORIENTED_EDGE ( 'NONE', *, *, #704, .F. ) ;
#14072=CARTESIAN_POINT ( 'NONE',  ( -82.40000000000001990, -33.26250000000000284, -103.0000000000000000 ) ) ;
#14073=CARTESIAN_POINT ( 'NONE',  ( 82.85452780460281019, -34.99999999999999289, -102.7245357809972575 ) ) ;
#14075=ORIENTED_EDGE ( 'NONE', *, *, #17376, .T. ) ;
#14078=CARTESIAN_POINT ( 'NONE',  ( 79.39999999999999147, -30.26249999999999929, -101.7320508075688537 ) ) ;
#14081=CARTESIAN_POINT ( 'NONE',  ( -82.39999999999999147, -33.20624999877097139, 96.53589838486223584 ) ) ;
#14083=CARTESIAN_POINT ( 'NONE',  ( 94.79999999999991189, -3.000000000000000000, 150.0000000000000000 ) ) ;
#14085=CARTESIAN_POINT ( 'NONE',  ( 79.64356964374998427, -32.76562499938548711, -101.5914258081833879 ) ) ;
#14086=CARTESIAN_POINT ( 'NONE',  ( 80.90000000000000568, -33.75000000000000000, 102.5980762113533018 ) ) ;
#14087=CARTESIAN_POINT ( 'NONE',  ( -82.39999999999999147, -32.72812499938548569, 103.1828516163667899 ) ) ;
#14090=( NAMED_UNIT ( * ) PLANE_ANGLE_UNIT ( ) SI_UNIT ( $, .RADIAN. ) );
#14091=CARTESIAN_POINT ( 'NONE',  ( -79.39999999999999147, -33.86250000000000426, 101.7320508075688537 ) ) ;
#14096=CARTESIAN_POINT ( 'NONE',  ( -79.39999999999999147, -32.06250000000000000, 101.7320508075688537 ) ) ;
#14098=CARTESIAN_POINT ( 'NONE',  ( -81.79008970393689992, -35.00000000000000000, -97.30603528924575585 ) ) ;
#14100=CARTESIAN_POINT ( 'NONE',  ( 79.64356964375001269, -33.55312499938548854, 98.40857419181659793 ) ) ;
#14103=CARTESIAN_POINT ( 'NONE',  ( 83.20384757729337366, -32.55134618820330417, -103.0000000000000000 ) ) ;
#14105=CARTESIAN_POINT ( 'NONE',  ( 94.79999999999995453, -32.00000000000000000, 150.0000000000000000 ) ) ;
#14106=CARTESIAN_POINT ( 'NONE',  ( 79.64356964374999848, -32.61562499938548854, 99.99999999999998579 ) ) ;
#14107=CARTESIAN_POINT ( 'NONE',  ( 83.77821517812500929, -31.22812499938548569, -97.61286128772489690 ) ) ;
#14109=CARTESIAN_POINT ( 'NONE',  ( -85.15643035625001289, -34.30312499938548854, 99.99999999999998579 ) ) ;
#14110=CARTESIAN_POINT ( 'NONE',  ( -83.77821517812500929, -31.56562499938548427, -102.3871387122750889 ) ) ;
#14112=CARTESIAN_POINT ( 'NONE',  ( 82.39999999999999147, -33.51562499938548001, 103.1828516163667899 ) ) ;
#14114=CARTESIAN_POINT ( 'NONE',  ( -81.02178482187500208, -32.09062499938548285, 97.61286128772489690 ) ) ;
#14115=CARTESIAN_POINT ( 'NONE',  ( -85.15643035625001289, -33.40312499938548285, 99.99999999999998579 ) ) ;
#14116=CARTESIAN_POINT ( 'NONE',  ( 82.40000000000000568, -30.00000000000000355, 99.99999999999998579 ) ) ;
#14118=CARTESIAN_POINT ( 'NONE',  ( -79.39999999999999147, -34.31250000000000000, -98.26794919243113213 ) ) ;
#14119=DIRECTION ( 'NONE',  ( 0.000000000000000000, 0.000000000000000000, 1.000000000000000000 ) ) ;
#14122=EDGE_CURVE ( 'NONE', #11560, #5607, #12717, .T. ) ;
#14126=CARTESIAN_POINT ( 'NONE',  ( 79.39999999999999147, -32.83124999877097139, -98.26794919243110371 ) ) ;
#14127=CARTESIAN_POINT ( 'NONE',  ( 83.20395887649176814, -35.00000000000002132, 97.36341917746361219 ) ) ;
#14128=CARTESIAN_POINT ( 'NONE',  ( 79.64356964374999848, -30.92812499938548498, 99.99999999999998579 ) ) ;
#14132=DIRECTION ( 'NONE',  ( 0.000000000000000000, 0.000000000000000000, -1.000000000000000000 ) ) ;
#14133=CARTESIAN_POINT ( 'NONE',  ( 82.39999999999999147, -31.94062499938548427, -103.1828516163667899 ) ) ;
#14135=ORIENTED_EDGE ( 'NONE', *, *, #9187, .F. ) ;
#14136=CARTESIAN_POINT ( 'NONE',  ( 80.90000000000000568, -31.14374999877097139, 97.40192378864668399 ) ) ;
#14137=SHAPE_DEFINITION_REPRESENTATION ( #18565, #406 ) ;
#14138=ADVANCED_FACE ( 'NONE', ( #2498 ), #763, .F. ) ;
#14141=EDGE_CURVE ( 'NONE', #16515, #5564, #8095, .T. ) ;
#14146=CARTESIAN_POINT ( 'NONE',  ( -79.64356964375001269, -32.12812499938548427, -101.5914258081833879 ) ) ;
#14147=EDGE_CURVE ( 'NONE', #14, #16006, #16597, .T. ) ;
#14148=DIRECTION ( 'NONE',  ( -1.000000000000000000, 0.000000000000000000, 0.000000000000000000 ) ) ;
#14150=CARTESIAN_POINT ( 'NONE',  ( 83.77821517812500929, -32.87812499938548427, 97.61286128772489690 ) ) ;
#14151=CARTESIAN_POINT ( 'NONE',  ( -79.39999999999999147, -34.25624999877096855, -98.26794919243113213 ) ) ;
#14152=CARTESIAN_POINT ( 'NONE',  ( 83.90000000000000568, -34.57500000000000284, 102.5980762113533018 ) ) ;
#14156=CARTESIAN_POINT ( 'NONE',  ( 83.65502553131049979, -34.99999999999999289, -102.4885329066889028 ) ) ;
#14158=EDGE_CURVE ( 'NONE', #16231, #17606, #4735, .T. ) ;
#14161=ORIENTED_EDGE ( 'NONE', *, *, #6672, .T. ) ;
#14162=CARTESIAN_POINT ( 'NONE',  ( 81.02178482187500208, -32.54062499938548569, -97.61286128772489690 ) ) ;
#14168=CYLINDRICAL_SURFACE ( 'NONE', #6497, 3.000000000000002665 ) ;
#14174=CARTESIAN_POINT ( 'NONE',  ( 80.90000000000000568, -33.75000000000000000, -97.40192378864668399 ) ) ;
#14176=CARTESIAN_POINT ( 'NONE',  ( -81.02178482187500208, -34.90312499938548285, -102.3871387122750889 ) ) ;
#14177=CARTESIAN_POINT ( 'NONE',  ( -80.90000000000000568, -35.04374999877096997, 97.40192378864668399 ) ) ;
#14179=CARTESIAN_POINT ( 'NONE',  ( 83.90000000000000568, -32.32500000000000284, -97.40192378864668399 ) ) ;
#14183=CARTESIAN_POINT ( 'NONE',  ( -81.02178482187500208, -33.14062499938548711, 102.3871387122750889 ) ) ;
#14184=CARTESIAN_POINT ( 'NONE',  ( 82.40000000000000568, -30.00000000000000355, -99.99999999999998579 ) ) ;
#14187=CARTESIAN_POINT ( 'NONE',  ( -82.40000000000000568, -30.00000000000000355, -103.0000000000000000 ) ) ;
#14193=ORIENTED_EDGE ( 'NONE', *, *, #3870, .T. ) ;
#14194=APPLICATION_CONTEXT ( 'automotive_design' ) ;
#14196=CARTESIAN_POINT ( 'NONE',  ( 83.03192786677290371, -34.99999999999999289, 97.31096265645994947 ) ) ;
#14197=CARTESIAN_POINT ( 'NONE',  ( 81.02178482187500208, -32.09062499938548285, 102.3871387122750889 ) ) ;
#14201=CARTESIAN_POINT ( 'NONE',  ( -81.02178482187500208, -32.20312499938548711, -102.3871387122750889 ) ) ;
#14202=CARTESIAN_POINT ( 'NONE',  ( 85.15643035624999868, -32.80312499938548854, 98.40857419181659793 ) ) ;
#14203=CARTESIAN_POINT ( 'NONE',  ( 79.64356964375001269, -35.01562499938548711, -101.5914258081833879 ) ) ;
#14205=CARTESIAN_POINT ( 'NONE',  ( -84.05108659120801917, -32.00820041275124339, 97.77040367152252998 ) ) ;
#14206=EDGE_LOOP ( 'NONE', ( #14043, #18392, #18441, #14919 ) ) ;
#14207=CARTESIAN_POINT ( 'NONE',  ( 82.39999999999999147, -31.71562499938548640, 103.1828516163667899 ) ) ;
#14210=CARTESIAN_POINT ( 'NONE',  ( -85.15643035624999868, -30.62812499938548427, 98.40857419181659793 ) ) ;
#14211=CARTESIAN_POINT ( 'NONE',  ( -85.15643035624999868, -31.90312499938548285, 101.5914258081833879 ) ) ;
#14213=VERTEX_POINT ( 'NONE', #10220 ) ;
#14214=CARTESIAN_POINT ( 'NONE',  ( -80.90000000000000568, -34.20000000000000284, -102.5980762113533018 ) ) ;
#14216=DIRECTION ( 'NONE',  ( -0.000000000000000000, -0.000000000000000000, -1.000000000000000000 ) ) ;
#14219=CARTESIAN_POINT ( 'NONE',  ( -82.40000000000000568, -34.78124999877096712, -96.99999999999998579 ) ) ;
#14220=CARTESIAN_POINT ( 'NONE',  ( 83.90000000000000568, -34.06874999877096855, -97.40192378864668399 ) ) ;
#14221=CARTESIAN_POINT ( 'NONE',  ( -82.39999999999999147, -33.43124999877097281, -96.99999999999998579 ) ) ;
#14222=CARTESIAN_POINT ( 'NONE',  ( -83.20384757729335945, -33.05759618943233136, 102.9999999999999858 ) ) ;
#14223=CARTESIAN_POINT ( 'NONE',  ( 85.15643035625001289, -30.70312499938548711, 99.99999999999998579 ) ) ;
#14225=CARTESIAN_POINT ( 'NONE',  ( -85.40000000000000568, -32.66250000000000142, -98.26794919243111792 ) ) ;
#14226=CARTESIAN_POINT ( 'NONE',  ( 83.77821517812500929, -30.62812499938548783, -102.3871387122750889 ) ) ;
#14229=EDGE_LOOP ( 'NONE', ( #13982, #13590, #16416, #8020 ) ) ;
#14230=CARTESIAN_POINT ( 'NONE',  ( 79.39999999999999147, -30.61874999877096926, 99.99999999999998579 ) ) ;
#14234=EDGE_CURVE ( 'NONE', #8302, #14497, #6019, .T. ) ;
#14236=CARTESIAN_POINT ( 'NONE',  ( -83.65502553130849606, -35.00000000000002842, -97.51146709331030138 ) ) ;
#14237=VERTEX_POINT ( 'NONE', #1621 ) ;
#14238=CARTESIAN_POINT ( 'NONE',  ( -81.02178482187500208, -30.89062499938548711, -97.61286128772489690 ) ) ;
#14240=VERTEX_POINT ( 'NONE', #14799 ) ;
#14241=CARTESIAN_POINT ( 'NONE',  ( 85.15643035625001289, -32.46562499938548996, 98.40857419181659793 ) ) ;
#14242=CARTESIAN_POINT ( 'NONE',  ( -81.02178482187500208, -30.55312499938548854, -97.61286128772489690 ) ) ;
#14243=( BOUNDED_CURVE ( )  B_SPLINE_CURVE ( 2, ( #10519, #13252, #16487, #7393, #8950, #19126, #12079, #14918, #2994 ),
 .UNSPECIFIED., .F., .F. ) 
 B_SPLINE_CURVE_WITH_KNOTS ( ( 3, 2, 2, 2, 3 ),
 ( 0.6041666666666666297, 0.6111111111111111605, 0.6250000000000000000, 0.6388888888888888395, 0.6458333333333333703 ),
 .UNSPECIFIED. ) 
 CURVE ( )  GEOMETRIC_REPRESENTATION_ITEM ( )  RATIONAL_B_SPLINE_CURVE ( ( 0.9330127018922192983, 0.9330127018922187432, 1.000000000000000000, 0.8660254037844387076, 1.000000000000000000, 0.8660254037844387076, 1.000000000000000000, 0.9330127018922187432, 0.9330127018922192983 ) ) 
 REPRESENTATION_ITEM ( '' )  );
#14244=CARTESIAN_POINT ( 'NONE',  ( 79.39999999999999147, -34.76250000000000284, 98.26794919243113213 ) ) ;
#14245=CARTESIAN_POINT ( 'NONE',  ( -80.85389467647070205, -34.99999999999999289, 97.51091559654260266 ) ) ;
#14248=CARTESIAN_POINT ( 'NONE',  ( -79.64356964374998427, -33.55312499938548854, -98.40857419181659793 ) ) ;
#14250=EDGE_CURVE ( 'NONE', #3130, #15577, #14697, .T. ) ;
#14252=CARTESIAN_POINT ( 'NONE',  ( 94.79999999999995453, -29.80000000000000071, -150.0000000000000000 ) ) ;
#14256=CARTESIAN_POINT ( 'NONE',  ( 82.39999999999999147, -33.62812499938548427, -103.1828516163667899 ) ) ;
#14257=CARTESIAN_POINT ( 'NONE',  ( -83.77821517812500929, -34.71562499938548285, -102.3871387122750889 ) ) ;
#14259=VERTEX_POINT ( 'NONE', #1336 ) ;
#14263=ORIENTED_EDGE ( 'NONE', *, *, #8428, .F. ) ;
#14264=CARTESIAN_POINT ( 'NONE',  ( -82.39999999999999147, -32.98124999877096286, -96.99999999999998579 ) ) ;
#14268=CARTESIAN_POINT ( 'NONE',  ( 79.39999999999999147, -31.98750000000000071, -98.26794919243110371 ) ) ;
#14272=CARTESIAN_POINT ( 'NONE',  ( -83.77821517812500929, -32.12812499938548427, 97.61286128772489690 ) ) ;
#14274=UNCERTAINTY_MEASURE_WITH_UNIT (LENGTH_MEASURE( 1.000000000000000082E-05 ), #533, 'distance_accuracy_value', 'NONE');
#14277=CARTESIAN_POINT ( 'NONE',  ( 84.28136653320183314, -32.00000000000000711, 102.0145392219077394 ) ) ;
#14278=VECTOR ( 'NONE', #3354, 1000.000000000000000 ) ;
#14280=CARTESIAN_POINT ( 'NONE',  ( -85.15643035625001289, -32.39062499938548711, 99.99999999999998579 ) ) ;
#14281=DIRECTION ( 'NONE',  ( 0.000000000000000000, 0.000000000000000000, 1.000000000000000000 ) ) ;
#14282=ORIENTED_EDGE ( 'NONE', *, *, #10777, .T. ) ;
#14286=CARTESIAN_POINT ( 'NONE',  ( 83.32052461991715120, -34.98323688327303671, 102.9326364780328760 ) ) ;
#14290=ORIENTED_EDGE ( 'NONE', *, *, #11902, .T. ) ;
#14292=AXIS2_PLACEMENT_3D ( 'NONE', #4958, #13825, #10901 ) ;
#14295=CARTESIAN_POINT ( 'NONE',  ( -79.39999999999999147, -33.78750000000000853, -101.7320508075688963 ) ) ;
#14296=CARTESIAN_POINT ( 'NONE',  ( 82.39999999999999147, -32.27812499938548285, 96.81714838363319586 ) ) ;
#14297=DIRECTION ( 'NONE',  ( 1.000000000000000000, 0.000000000000000000, 4.625929269271481378E-15 ) ) ;
#14300=CARTESIAN_POINT ( 'NONE',  ( -85.15643035625001289, -33.44062499938548427, -101.5914258081833879 ) ) ;
#14301=CARTESIAN_POINT ( 'NONE',  ( 82.39999999999999147, -32.72812499938548569, 96.81714838363319586 ) ) ;
#14302=CARTESIAN_POINT ( 'NONE',  ( 85.15643035625001289, -33.40312499938548285, -99.99999999999998579 ) ) ;
#14304=CARTESIAN_POINT ( 'NONE',  ( -79.64356964374999848, -33.51562499938548711, 99.99999999999998579 ) ) ;
#14305=CARTESIAN_POINT ( 'NONE',  ( 79.64356964375001269, -30.32812499938548711, -98.40857419181659793 ) ) ;
#14310=CARTESIAN_POINT ( 'NONE',  ( -83.77821517812500929, -30.21562499938548285, 97.61286128772489690 ) ) ;
#14311=CARTESIAN_POINT ( 'NONE',  ( -85.15643035624999868, -31.45312499938548356, 101.5914258081833879 ) ) ;
#14313=EDGE_LOOP ( 'NONE', ( #11574, #10161, #7419, #1653 ) ) ;
#14314=CARTESIAN_POINT ( 'NONE',  ( -85.40000000000000568, -33.56250000000000000, -98.26794919243111792 ) ) ;
#14316=LINE ( 'NONE', #955, #17949 ) ;
#14322=CARTESIAN_POINT ( 'NONE',  ( -82.39999999999999147, -32.98124999877096286, -96.99999999999998579 ) ) ;
#14325=CARTESIAN_POINT ( 'NONE',  ( 94.79999999999984084, 0.000000000000000000, -150.0000000000000000 ) ) ;
#14326=CARTESIAN_POINT ( 'NONE',  ( 79.64356964374999848, -33.17812499938548854, -99.99999999999998579 ) ) ;
#14327=ORIENTED_EDGE ( 'NONE', *, *, #18568, .T. ) ;
#14328=CARTESIAN_POINT ( 'NONE',  ( 85.40000000000000568, -31.33124999877096428, 101.7320508075688679 ) ) ;
#14334=ORIENTED_EDGE ( 'NONE', *, *, #7911, .T. ) ;
#14335=CARTESIAN_POINT ( 'NONE',  ( -83.77821517812500929, -31.86562499938548498, -97.61286128772489690 ) ) ;
#14336=LINE ( 'NONE', #17570, #7858 ) ;
#14337=ORIENTED_EDGE ( 'NONE', *, *, #3251, .F. ) ;
#14338=CARTESIAN_POINT ( 'NONE',  ( 81.02178482187500208, -32.65312499938548996, 102.3871387122750889 ) ) ;
#14339=CARTESIAN_POINT ( 'NONE',  ( -85.15643035625001289, -32.05312499938548854, -99.99999999999998579 ) ) ;
#14340=CARTESIAN_POINT ( 'NONE',  ( -83.90000000000000568, -30.46874999877096712, -102.5980762113533018 ) ) ;
#14341=CARTESIAN_POINT ( 'NONE',  ( 80.90000000000000568, -34.74374999877097281, -102.5980762113533018 ) ) ;
#14344=CARTESIAN_POINT ( 'NONE',  ( -83.77821517812500929, -32.91562499938547859, -102.3871387122750889 ) ) ;
#14348=CARTESIAN_POINT ( 'NONE',  ( 80.90000000000000568, -30.69374999877097210, -102.5980762113533018 ) ) ;
#14351=CARTESIAN_POINT ( 'NONE',  ( 85.15643035625001289, -33.25312499938548427, -101.5914258081833879 ) ) ;
#14358=ORIENTED_EDGE ( 'NONE', *, *, #15091, .T. ) ;
#14361=ADVANCED_FACE ( 'NONE', ( #1315 ), #4338, .T. ) ;
#14364=CARTESIAN_POINT ( 'NONE',  ( 82.39999999999999147, -33.93750000000000000, -103.4641016151377499 ) ) ;
#14366=CARTESIAN_POINT ( 'NONE',  ( -85.15643035624999868, -31.56562499938548427, 101.5914258081833879 ) ) ;
#14368=CARTESIAN_POINT ( 'NONE',  ( -82.39999999999999147, -34.83749999999999858, -97.00000000000000000 ) ) ;
#14371=CARTESIAN_POINT ( 'NONE',  ( 82.40000000000000568, -34.10624999877096997, 102.9999999999999858 ) ) ;
#14373=CARTESIAN_POINT ( 'NONE',  ( 84.70388354820681798, -35.00002705695767702, 101.9214814096700934 ) ) ;
#14382=EDGE_CURVE ( 'NONE', #13090, #3915, #5248, .T. ) ;
#14385=CARTESIAN_POINT ( 'NONE',  ( 85.40000000000000568, -32.23124999877096997, -98.26794919243111792 ) ) ;
#14386=CARTESIAN_POINT ( 'NONE',  ( 79.64356964375001269, -34.00312499938549138, 98.40857419181659793 ) ) ;
#14387=DIRECTION ( 'NONE',  ( -0.000000000000000000, -1.000000000000000000, -0.000000000000000000 ) ) ;
#14390=CARTESIAN_POINT ( 'NONE',  ( -85.15643035625001289, -34.30312499938548854, -99.99999999999998579 ) ) ;
#14391=CARTESIAN_POINT ( 'NONE',  ( 79.64356964375001269, -31.75312499938548427, 98.40857419181659793 ) ) ;
#14392=CARTESIAN_POINT ( 'NONE',  ( 79.64356964375001269, -33.59062499938548285, -98.40857419181659793 ) ) ;
#14393=EDGE_CURVE ( 'NONE', #15931, #4595, #17626, .T. ) ;
#14395=CARTESIAN_POINT ( 'NONE',  ( -85.15643035625001289, -33.77812499938548285, 98.40857419181659793 ) ) ;
#14396=CARTESIAN_POINT ( 'NONE',  ( 79.64356964375001269, -31.75312499938548427, -101.5914258081833879 ) ) ;
#14397=ORIENTED_EDGE ( 'NONE', *, *, #14008, .F. ) ;
#14399=DIRECTION ( 'NONE',  ( 1.000000000000000000, -1.586032892321652285E-15, 0.000000000000000000 ) ) ;
#14401=CARTESIAN_POINT ( 'NONE',  ( -79.64356964375001269, -33.47812499938547859, 98.40857419181659793 ) ) ;
#14402=CARTESIAN_POINT ( 'NONE',  ( -82.39999999999999147, -30.92812499938548143, 103.1828516163667899 ) ) ;
#14403=LINE ( 'NONE', #6905, #4628 ) ;
#14410=CARTESIAN_POINT ( 'NONE',  ( 85.40000000000000568, -33.95624999877097139, -101.7320508075688821 ) ) ;
#14413=CARTESIAN_POINT ( 'NONE',  ( -83.90000000000000568, -33.01874999877097139, -97.40192378864668399 ) ) ;
#14415=CARTESIAN_POINT ( 'NONE',  ( -83.20384757729335945, -32.60759618943233562, -96.99999999999997158 ) ) ;
#14416=CARTESIAN_POINT ( 'NONE',  ( 83.77821517812500929, -33.47812499938548569, -97.61286128772489690 ) ) ;
#14420=ORIENTED_EDGE ( 'NONE', *, *, #2788, .T. ) ;
#14421=CARTESIAN_POINT ( 'NONE',  ( 82.39999999999999147, -34.33124999877097139, 96.53589838486223584 ) ) ;
#14426=CARTESIAN_POINT ( 'NONE',  ( 99.99999999999998579, 0.000000000000000000, 150.0000000000000000 ) ) ;
#14428=CARTESIAN_POINT ( 'NONE',  ( -85.15643035625001289, -34.19062499938548427, -99.99999999999998579 ) ) ;
#14429=CARTESIAN_POINT ( 'NONE',  ( 85.40000000000000568, -33.18750000000000000, 101.7320508075688821 ) ) ;
#14431=CARTESIAN_POINT ( 'NONE',  ( 85.15643035625001289, -32.54062499938548569, 101.5914258081833879 ) ) ;
#14432=CARTESIAN_POINT ( 'NONE',  ( -83.77821517812500929, -31.67812499938548498, -102.3871387122750889 ) ) ;
#14434=CARTESIAN_POINT ( 'NONE',  ( 83.90000000000000568, -33.67500000000000426, 102.5980762113533018 ) ) ;
#14438=B_SPLINE_CURVE_WITH_KNOTS ( 'NONE', 3,
 ( #4427, #9300, #16445, #10582, #237, #43, #7745, #15264, #1690, #3055, #7547, #17817, #7838, #342, #13792, #11945, #13505, #12238 ),
 .UNSPECIFIED., .F., .F.,
 ( 4, 2, 2, 2, 2, 2, 2, 2, 4 ),
 ( 0.000000000000000000, 0.0007106627595359221467, 0.001421325519071844293, 0.002131988278607766657, 0.002842651038143688587, 0.003553313797679610517, 0.004263976557215533314, 0.004974639316751455244, 0.005685302076287377174 ),
 .UNSPECIFIED. ) ;
#14439=CARTESIAN_POINT ( 'NONE',  ( -80.90000000000000568, -34.29374999877096997, -97.40192378864668399 ) ) ;
#14440=CARTESIAN_POINT ( 'NONE',  ( 85.40000000000000568, -32.23124999877096997, -98.26794919243111792 ) ) ;
#14442=EDGE_LOOP ( 'NONE', ( #10596, #6029, #748, #13789 ) ) ;
#14454=CARTESIAN_POINT ( 'NONE',  ( 85.40000000000000568, -33.60000000000000142, -99.99999999999998579 ) ) ;
#14455=CARTESIAN_POINT ( 'NONE',  ( 83.52979456739228681, -32.00000000000000000, -102.5803447510191972 ) ) ;
#14456=CARTESIAN_POINT ( 'NONE',  ( -82.39999999999999147, -30.59062499938548640, 103.1828516163667899 ) ) ;
#14465=CARTESIAN_POINT ( 'NONE',  ( -85.15643035625001289, -30.14062499938548711, -99.99999999999998579 ) ) ;
#14466=CARTESIAN_POINT ( 'NONE',  ( -82.40000000000000568, -30.00000000000000355, -96.99999999999998579 ) ) ;
#14469=CARTESIAN_POINT ( 'NONE',  ( 83.90000000000000568, -34.81874999877096855, 97.40192378864668399 ) ) ;
#14477=CARTESIAN_POINT ( 'NONE',  ( -82.39999999999999147, -30.73124999877096641, 103.4641016151377499 ) ) ;
#14478=CARTESIAN_POINT ( 'NONE',  ( 82.39999999999999147, -34.07812499938548711, 96.81714838363319586 ) ) ;
#14481=CARTESIAN_POINT ( 'NONE',  ( 83.20384757729335945, -32.73615380933863150, -96.99999999999998579 ) ) ;
#14483=CARTESIAN_POINT ( 'NONE',  ( -82.39999999999999147, -33.06562499938548427, -103.1828516163667899 ) ) ;
#14484=CARTESIAN_POINT ( 'NONE',  ( 82.39999999999999147, -33.20624999877097849, -97.00000000000000000 ) ) ;
#14486=CARTESIAN_POINT ( 'NONE',  ( 79.64356964374999848, -34.52812499938548285, -99.99999999999998579 ) ) ;
#14488=CARTESIAN_POINT ( 'NONE',  ( -82.39999999999999147, -33.85312499938548569, 96.81714838363319586 ) ) ;
#14491=ORIENTED_EDGE ( 'NONE', *, *, #9393, .T. ) ;
#14492=CARTESIAN_POINT ( 'NONE',  ( 85.15643035625001289, -34.30312499938548854, 99.99999999999998579 ) ) ;
#14493=CARTESIAN_POINT ( 'NONE',  ( -82.39999999999999147, -32.58750000000000568, 102.9999999999999858 ) ) ;
#14495=CARTESIAN_POINT ( 'NONE',  ( -82.39999999999999147, -33.62812499938549138, 103.1828516163667899 ) ) ;
#14496=CARTESIAN_POINT ( 'NONE',  ( -85.15643035624999868, -31.07812499938548356, 98.40857419181659793 ) ) ;
#14497=VERTEX_POINT ( 'NONE', #3800 ) ;
#14498=CARTESIAN_POINT ( 'NONE',  ( -82.40000000000000568, -33.71249999999998437, -102.9999999999999858 ) ) ;
#14501=CARTESIAN_POINT ( 'NONE',  ( -94.79999999999999716, -32.00000000000000000, 150.0000000000000000 ) ) ;
#14504=CARTESIAN_POINT ( 'NONE',  ( -79.39999999999999147, -32.86874999877097281, 99.99999999999998579 ) ) ;
#14506=CARTESIAN_POINT ( 'NONE',  ( 84.67508262029681987, -32.00000000000000000, 98.43364869553350616 ) ) ;
#14508=LINE ( 'NONE', #1144, #10254 ) ;
#14509=FACE_OUTER_BOUND ( 'NONE', #5956, .T. ) ;
#14510=CARTESIAN_POINT ( 'NONE',  ( 81.02178482187500208, -34.45312499938548711, -97.61286128772489690 ) ) ;
#14513=VERTEX_POINT ( 'NONE', #889 ) ;
#14515=CARTESIAN_POINT ( 'NONE',  ( 80.90000000000000568, -32.34374999877096712, 102.5980762113533018 ) ) ;
#14518=ADVANCED_FACE ( 'NONE', ( #12409 ), #4896, .F. ) ;
#14521=CARTESIAN_POINT ( 'NONE',  ( -83.20395887649183919, -35.00000000000001421, -97.36341917746362640 ) ) ;
#14522=ORIENTED_EDGE ( 'NONE', *, *, #15000, .T. ) ;
#14523=CARTESIAN_POINT ( 'NONE',  ( -83.77821517812500929, -34.11562499938548854, -97.61286128772489690 ) ) ;
#14525=VERTEX_POINT ( 'NONE', #3515 ) ;
#14528=CARTESIAN_POINT ( 'NONE',  ( -82.39999999999999147, -32.16562499938549280, -103.1828516163667899 ) ) ;
#14530=CARTESIAN_POINT ( 'NONE',  ( -80.90000000000000568, -31.14374999877097139, -97.40192378864668399 ) ) ;
#14531=CARTESIAN_POINT ( 'NONE',  ( -79.69416654173919312, -34.99999999999999289, 100.6274906301336216 ) ) ;
#14534=CARTESIAN_POINT ( 'NONE',  ( -79.64356964374999848, -32.61562499938548854, -99.99999999999998579 ) ) ;
#14536=CARTESIAN_POINT ( 'NONE',  ( 83.90000000000000568, -31.66874999877096997, -102.5980762113533018 ) ) ;
#14538=ORIENTED_EDGE ( 'NONE', *, *, #14234, .T. ) ;
#14545=ORIENTED_EDGE ( 'NONE', *, *, #10564, .F. ) ;
#14548=ORIENTED_EDGE ( 'NONE', *, *, #1020, .F. ) ;
#14549=CARTESIAN_POINT ( 'NONE',  ( -82.65333140691201663, -34.99995246259153703, -102.9892844631211943 ) ) ;
#14550=CARTESIAN_POINT ( 'NONE',  ( 83.90000000000000568, -32.32500000000000284, -97.40192378864668399 ) ) ;
#14552=CARTESIAN_POINT ( 'NONE',  ( -82.39999999999999147, -31.04062499938548569, 103.1828516163667899 ) ) ;
#14554=DIRECTION ( 'NONE',  ( 0.000000000000000000, -1.000000000000000000, 0.000000000000000000 ) ) ;
#14555=CARTESIAN_POINT ( 'NONE',  ( 85.15643035625001289, -34.60312499938548569, 98.40857419181659793 ) ) ;
#14557=DIRECTION ( 'NONE',  ( -0.000000000000000000, -0.000000000000000000, -1.000000000000000000 ) ) ;
#14561=SURFACE_STYLE_FILL_AREA ( #4125 ) ;
#14562=CARTESIAN_POINT ( 'NONE',  ( -79.64356964375001269, -30.40312499938548285, -98.40857419181659793 ) ) ;
#14573=CARTESIAN_POINT ( 'NONE',  ( 79.39999999999999147, -30.22500000000000142, 99.99999999999998579 ) ) ;
#14576=CARTESIAN_POINT ( 'NONE',  ( -82.40000000000000568, -30.00000000000000355, 99.99999999999998579 ) ) ;
#14581=CARTESIAN_POINT ( 'NONE',  ( -79.64356964374999848, -33.62812499938548427, -99.99999999999998579 ) ) ;
#14582=CARTESIAN_POINT ( 'NONE',  ( 81.02178482187500208, -33.89062499938548711, 102.3871387122750889 ) ) ;
#14584=( BOUNDED_CURVE ( )  B_SPLINE_CURVE ( 2, ( #11736, #16042, #3037, #4318, #5978, #19074, #11834, #7154, #16241 ),
 .UNSPECIFIED., .F., .F. ) 
 B_SPLINE_CURVE_WITH_KNOTS ( ( 3, 2, 2, 2, 3 ),
 ( 0.8125000000000000000, 0.8194444444444444198, 0.8333333333333333703, 0.8472222222222222099, 0.8541666666666665186 ),
 .UNSPECIFIED. ) 
 CURVE ( )  GEOMETRIC_REPRESENTATION_ITEM ( )  RATIONAL_B_SPLINE_CURVE ( ( 0.9330127018922194093, 0.9330127018922194093, 1.000000000000000000, 0.8660254037844387076, 1.000000000000000000, 0.8660254037844387076, 1.000000000000000000, 0.9330127018922209636, 0.9330127018922194093 ) ) 
 REPRESENTATION_ITEM ( '' )  );
#14585=( GEOMETRIC_REPRESENTATION_CONTEXT ( 3 ) GLOBAL_UNCERTAINTY_ASSIGNED_CONTEXT ( ( #15274 ) ) GLOBAL_UNIT_ASSIGNED_CONTEXT ( ( #16243, #7156, #10370 ) ) REPRESENTATION_CONTEXT ( 'NONE', 'WORKASPACE' ) );
#14586=EDGE_CURVE ( 'NONE', #15758, #11141, #17970, .T. ) ;
#14587=CARTESIAN_POINT ( 'NONE',  ( 85.15643035624999868, -35.22676555956768141, -98.99674139749697588 ) ) ;
#14589=CARTESIAN_POINT ( 'NONE',  ( -83.77821517812500929, -33.36562499938548854, 97.61286128772489690 ) ) ;
#14595=CARTESIAN_POINT ( 'NONE',  ( -82.39999999999999147, -32.72812499938548569, 103.1828516163667899 ) ) ;
#14603=CARTESIAN_POINT ( 'NONE',  ( 80.48808202378427268, -35.00000000000000711, -97.80480077079582202 ) ) ;
#14609=CARTESIAN_POINT ( 'NONE',  ( 79.64356964375001269, -33.59062499938548285, 101.5914258081833879 ) ) ;
#14611=CARTESIAN_POINT ( 'NONE',  ( -99.99999999999998579, -3.000000000000000000, -150.0000000000000000 ) ) ;
#14613=CARTESIAN_POINT ( 'NONE',  ( 85.15643035625001289, -34.30312499938548854, -99.99999999999998579 ) ) ;
#14615=CARTESIAN_POINT ( 'NONE',  ( 79.39999999999999147, -32.90624999877096712, 98.26794919243113213 ) ) ;
#14619=CARTESIAN_POINT ( 'NONE',  ( 110.9999999999999574, -21.80000000000003268, -139.9999999999999716 ) ) ;
#14621=VERTEX_POINT ( 'NONE', #15730 ) ;
#14622=CARTESIAN_POINT ( 'NONE',  ( -85.15643035624999868, -33.25312499938548427, -98.40857419181659793 ) ) ;
#14623=CARTESIAN_POINT ( 'NONE',  ( 94.79999999999995453, -32.00000000000000000, 150.0000000000000000 ) ) ;
#14624=ORIENTED_EDGE ( 'NONE', *, *, #10245, .F. ) ;
#14626=CARTESIAN_POINT ( 'NONE',  ( -79.39999999999999147, -35.15624999877096712, -98.26794919243113213 ) ) ;
#14627=DIRECTION ( 'NONE',  ( 0.000000000000000000, -0.000000000000000000, -1.000000000000000000 ) ) ;
#14628=CARTESIAN_POINT ( 'NONE',  ( -79.39999999999999147, -31.10624999877097352, -98.26794919243113213 ) ) ;
#14632=CARTESIAN_POINT ( 'NONE',  ( -83.77821517812500929, -33.36562499938548854, -102.3871387122750889 ) ) ;
#14633=CARTESIAN_POINT ( 'NONE',  ( 79.39999999999999147, -32.47500000000000142, -99.99999999999998579 ) ) ;
#14635=CARTESIAN_POINT ( 'NONE',  ( 82.40000000000000568, -34.38749999999999574, -102.9999999999999858 ) ) ;
#14636=CARTESIAN_POINT ( 'NONE',  ( 82.39999999999999147, -31.85624999877097352, -96.53589838486223584 ) ) ;
#14638=ORIENTED_EDGE ( 'NONE', *, *, #10234, .T. ) ;
#14639=FACE_OUTER_BOUND ( 'NONE', #13294, .T. ) ;
#14644=ORIENTED_EDGE ( 'NONE', *, *, #8170, .F. ) ;
#14645=VERTEX_POINT ( 'NONE', #16114 ) ;
#14651=CARTESIAN_POINT ( 'NONE',  ( 79.39999999999999147, -34.76250000000000284, -101.7320508075688537 ) ) ;
#14653=PRODUCT_DEFINITION ( 'UNKNOWN', '', #10805, #6317 ) ;
#14654=CARTESIAN_POINT ( 'NONE',  ( -79.64356964375001269, -31.34062499938548640, 98.40857419181659793 ) ) ;
#14659=CARTESIAN_POINT ( 'NONE',  ( 82.17437583783167554, -34.99999999999999289, 102.9802575795477679 ) ) ;
#14660=CARTESIAN_POINT ( 'NONE',  ( -83.77821517812500929, -34.71562499938548285, 97.61286128772489690 ) ) ;
#14662=ORIENTED_EDGE ( 'NONE', *, *, #18365, .F. ) ;
#14663=CARTESIAN_POINT ( 'NONE',  ( -85.15643035624999868, -30.17812499938548498, -101.5914258081833879 ) ) ;
#14665=( BOUNDED_CURVE ( )  B_SPLINE_CURVE ( 2, ( #13052, #17457, #19018, #16081, #13137, #857, #19111, #6819, #5731 ),
 .UNSPECIFIED., .F., .F. ) 
 B_SPLINE_CURVE_WITH_KNOTS ( ( 3, 2, 2, 2, 3 ),
 ( 0.8125000000000000000, 0.8194444444444444198, 0.8333333333333333703, 0.8472222222222222099, 0.8541666666666665186 ),
 .UNSPECIFIED. ) 
 CURVE ( )  GEOMETRIC_REPRESENTATION_ITEM ( )  RATIONAL_B_SPLINE_CURVE ( ( 0.9330127018922194093, 0.9330127018922194093, 1.000000000000000000, 0.8660254037844387076, 1.000000000000000000, 0.8660254037844387076, 1.000000000000000000, 0.9330127018922209636, 0.9330127018922194093 ) ) 
 REPRESENTATION_ITEM ( '' )  );
#14672=VERTEX_POINT ( 'NONE', #14635 ) ;
#14673=CARTESIAN_POINT ( 'NONE',  ( -84.41281071784420931, -32.00000000000000000, 98.10821574224533492 ) ) ;
#14675=CARTESIAN_POINT ( 'NONE',  ( -94.79999999999999716, -35.00000000000000000, 150.0000000000000000 ) ) ;
#14676=CARTESIAN_POINT ( 'NONE',  ( 85.15643035624999868, -34.60312499938548569, 98.40857419181659793 ) ) ;
#14677=CARTESIAN_POINT ( 'NONE',  ( 85.40000000000000568, -34.08749999999999858, -98.26794919243111792 ) ) ;
#14680=B_SPLINE_CURVE_WITH_KNOTS ( 'NONE', 3,
 ( #15478, #1281, #8698, #5424, #11364, #7229, #17233, #11266, #9805, #14098, #15672, #737, #13185, #2375, #12739, #8146 ),
 .UNSPECIFIED., .F., .F.,
 ( 4, 2, 2, 2, 2, 2, 2, 4 ),
 ( 0.000000000000000000, 0.0005391024520904662623, 0.001078204904180932525, 0.002156409808361806069, 0.002695512260452271030, 0.003234614712542735991, 0.003773717164633200519, 0.004312819616723665046 ),
 .UNSPECIFIED. ) ;
#14682=CARTESIAN_POINT ( 'NONE',  ( 85.15643035624999868, -33.77812499938548285, 101.5914258081833879 ) ) ;
#14683=CARTESIAN_POINT ( 'NONE',  ( 85.15643035625001289, -31.94062499938548427, -99.99999999999998579 ) ) ;
#14685=CARTESIAN_POINT ( 'NONE',  ( -85.40000000000000568, -34.05000000000000426, 99.99999999999998579 ) ) ;
#14688=LINE ( 'NONE', #17346, #15996 ) ;
#14691=CARTESIAN_POINT ( 'NONE',  ( -83.77821517812500929, -32.91562499938547859, 97.61286128772489690 ) ) ;
#14692=ORIENTED_EDGE ( 'NONE', *, *, #516, .T. ) ;
#14693=CARTESIAN_POINT ( 'NONE',  ( -83.43443729601585801, -35.00000000000000000, 102.5775038898421201 ) ) ;
#14697=( BOUNDED_CURVE ( )  B_SPLINE_CURVE ( 2, ( #10407, #7283, #11968, #13526, #17936 ),
 .UNSPECIFIED., .F., .T. ) 
 B_SPLINE_CURVE_WITH_KNOTS ( ( 3, 2, 3 ),
 ( 0.2975293541897522931, 0.3055555555555555802, 0.3125000000000001665 ),
 .UNSPECIFIED. ) 
 CURVE ( )  GEOMETRIC_REPRESENTATION_ITEM ( )  RATIONAL_B_SPLINE_CURVE ( ( 0.9346381638529801528, 0.9225778897267638001, 1.000000000000000000, 0.9330127018922177440, 0.9330127018922194093 ) ) 
 REPRESENTATION_ITEM ( '' )  );
#14698=CARTESIAN_POINT ( 'NONE',  ( -99.99999999999998579, -35.00000000000000000, 150.0000000000000000 ) ) ;
#14702=CARTESIAN_POINT ( 'NONE',  ( 82.39999999999999147, -33.29062499938549280, 96.81714838363319586 ) ) ;
#14703=DIRECTION ( 'NONE',  ( 1.000000000000000000, -0.000000000000000000, -2.407412430484046130E-31 ) ) ;
#14704=CARTESIAN_POINT ( 'NONE',  ( -79.39999999999999147, -32.43750000000000000, -101.7320508075688963 ) ) ;
#14705=CARTESIAN_POINT ( 'NONE',  ( 82.39999999999999147, -33.29062499938549280, -103.1828516163667899 ) ) ;
#14706=CARTESIAN_POINT ( 'NONE',  ( -85.15643035625001289, -30.25312499938548783, -99.99999999999998579 ) ) ;
#14708=CARTESIAN_POINT ( 'NONE',  ( 85.40000000000000568, -33.05624999877096570, 98.26794919243111792 ) ) ;
#14709=DIRECTION ( 'NONE',  ( -1.000000000000000000, 0.000000000000000000, 0.000000000000000000 ) ) ;
#14712=VECTOR ( 'NONE', #15040, 1000.000000000000000 ) ;
#14713=CARTESIAN_POINT ( 'NONE',  ( -82.39999999999999147, -30.36562499938549209, 96.81714838363319586 ) ) ;
#14714=CARTESIAN_POINT ( 'NONE',  ( 81.22643902601967625, -31.99999999999998579, 102.6636594982983155 ) ) ;
#14715=EDGE_LOOP ( 'NONE', ( #9655, #15231, #8065, #14161 ) ) ;
#14716=CARTESIAN_POINT ( 'NONE',  ( -79.64356964374999848, -33.51562499938548711, -99.99999999999998579 ) ) ;
#14720=CARTESIAN_POINT ( 'NONE',  ( 85.15643035625001289, -34.79062499938548569, 101.5914258081833879 ) ) ;
#14721=CARTESIAN_POINT ( 'NONE',  ( -81.02178482187500208, -34.45312499938548711, -102.3871387122750889 ) ) ;
#14722=DIRECTION ( 'NONE',  ( 0.000000000000000000, -0.000000000000000000, -1.000000000000000000 ) ) ;
#14723=CARTESIAN_POINT ( 'NONE',  ( -85.40000000000000568, -31.70624999877096784, -98.26794919243111792 ) ) ;
#14727=CARTESIAN_POINT ( 'NONE',  ( -85.15643035625001289, -34.19062499938548427, -99.99999999999998579 ) ) ;
#14732=CARTESIAN_POINT ( 'NONE',  ( 80.90000000000000568, -31.89374999877096784, -97.40192378864668399 ) ) ;
#14736=CARTESIAN_POINT ( 'NONE',  ( 82.39999999999999147, -34.30312499938548143, -96.81714838363319586 ) ) ;
#14739=ADVANCED_FACE ( 'NONE', ( #19142 ), #2524, .F. ) ;
#14742=ORIENTED_EDGE ( 'NONE', *, *, #1479, .T. ) ;
#14743=CARTESIAN_POINT ( 'NONE',  ( -84.11496519894868129, -32.00000000000000000, 97.81539907810714851 ) ) ;
#14746=CIRCLE ( 'NONE', #12257, 3.000000000000002665 ) ;
#14748=ORIENTED_EDGE ( 'NONE', *, *, #11514, .T. ) ;
#14749=CARTESIAN_POINT ( 'NONE',  ( -81.79008970393687150, -34.99999999999997868, 102.6939647107541873 ) ) ;
#14750=CARTESIAN_POINT ( 'NONE',  ( 82.40000000000000568, -30.00000000000000355, 99.99999999999998579 ) ) ;
#14752=CARTESIAN_POINT ( 'NONE',  ( -85.15643035624999868, -35.16562499938547859, 101.5914258081833879 ) ) ;
#14757=DIRECTION ( 'NONE',  ( 0.000000000000000000, 0.000000000000000000, -1.000000000000000000 ) ) ;
#14758=CARTESIAN_POINT ( 'NONE',  ( -82.39999999999999147, -34.75312499938549138, 96.81714838363319586 ) ) ;
#14759=VECTOR ( 'NONE', #17310, 1000.000000000000000 ) ;
#14763=CARTESIAN_POINT ( 'NONE',  ( -85.15643035624999868, -35.22676555956768141, -101.0032586025029815 ) ) ;
#14764=CARTESIAN_POINT ( 'NONE',  ( -82.40000000000000568, -33.71249999999998437, 96.99999999999998579 ) ) ;
#14769=EDGE_CURVE ( 'NONE', #14513, #10474, #9455, .T. ) ;
#14773=CARTESIAN_POINT ( 'NONE',  ( -84.69814068649969840, -35.00052333152936512, -101.9283540611242955 ) ) ;
#14775=CARTESIAN_POINT ( 'NONE',  ( -83.90000000000000568, -32.11874999877097281, 102.5980762113533018 ) ) ;
#14776=CARTESIAN_POINT ( 'NONE',  ( 83.90000000000000568, -30.07499999999999929, 102.5980762113533018 ) ) ;
#14782=CARTESIAN_POINT ( 'NONE',  ( 85.15643035624999868, -34.60312499938548569, 98.40857419181659793 ) ) ;
#14783=( BOUNDED_CURVE ( )  B_SPLINE_CURVE ( 2, ( #9444, #14222, #576, #18350, #14037, #5155, #12383, #11101, #8180 ),
 .UNSPECIFIED., .F., .F. ) 
 B_SPLINE_CURVE_WITH_KNOTS ( ( 3, 2, 2, 2, 3 ),
 ( 0.5625000000000000000, 0.5694444444444444198, 0.5833333333333333703, 0.5972222222222222099, 0.6041666666666666297 ),
 .UNSPECIFIED. ) 
 CURVE ( )  GEOMETRIC_REPRESENTATION_ITEM ( )  RATIONAL_B_SPLINE_CURVE ( ( 0.9330127018922194093, 0.9330127018922194093, 1.000000000000000000, 0.8660254037844387076, 1.000000000000000000, 0.8660254037844387076, 1.000000000000000000, 0.9330127018922198534, 0.9330127018922192983 ) ) 
 REPRESENTATION_ITEM ( '' )  );
#14784=CARTESIAN_POINT ( 'NONE',  ( 79.64356964375001269, -32.12812499938548427, -98.40857419181659793 ) ) ;
#14787=CARTESIAN_POINT ( 'NONE',  ( 85.15643035625001289, -32.84062499938548285, -99.99999999999998579 ) ) ;
#14792=CARTESIAN_POINT ( 'NONE',  ( -79.64356964375001269, -32.20312499938548001, 101.5914258081833879 ) ) ;
#14794=CARTESIAN_POINT ( 'NONE',  ( -82.40000000000001990, -33.88124999877096855, 103.0000000000000000 ) ) ;
#14796=CARTESIAN_POINT ( 'NONE',  ( 81.05805657947855991, -34.99999999999999289, -97.38506107425206437 ) ) ;
#14798=DIRECTION ( 'NONE',  ( -1.000000000000000000, -0.000000000000000000, -0.000000000000000000 ) ) ;
#14799=CARTESIAN_POINT ( 'NONE',  ( 84.70388354820684640, -35.00002705695777649, -98.07851859032987818 ) ) ;
#14801=CARTESIAN_POINT ( 'NONE',  ( 84.97866794691726966, -32.00000000000000000, 100.9899807706011927 ) ) ;
#14802=CARTESIAN_POINT ( 'NONE',  ( 82.39999999999999147, -31.71562499938548640, 103.1828516163667899 ) ) ;
#14803=FACE_OUTER_BOUND ( 'NONE', #10719, .T. ) ;
#14805=CARTESIAN_POINT ( 'NONE',  ( -79.64356964374999848, -32.72812499938548569, 99.99999999999998579 ) ) ;
#14806=CARTESIAN_POINT ( 'NONE',  ( -85.15643035624999868, -31.11562499938548854, -98.40857419181659793 ) ) ;
#14808=CARTESIAN_POINT ( 'NONE',  ( 83.90000000000000568, -34.06874999877096855, 102.5980762113533018 ) ) ;
#14809=CARTESIAN_POINT ( 'NONE',  ( -82.40000000000000568, -34.78124999877096712, 102.9999999999999858 ) ) ;
#14811=CARTESIAN_POINT ( 'NONE',  ( -83.77821517812500929, -31.22812499938548569, 97.61286128772489690 ) ) ;
#14812=CARTESIAN_POINT ( 'NONE',  ( 79.79868554281867432, -31.99999999999999289, 101.4716133421946012 ) ) ;
#14814=CARTESIAN_POINT ( 'NONE',  ( -82.39999999999999147, -34.52812499938548996, -96.81714838363319586 ) ) ;
#14818=CARTESIAN_POINT ( 'NONE',  ( -79.64356964375001269, -32.76562499938548711, -98.40857419181659793 ) ) ;
#14820=CARTESIAN_POINT ( 'NONE',  ( -85.40000000000000568, -30.80624999877096926, -98.26794919243111792 ) ) ;
#14825=CARTESIAN_POINT ( 'NONE',  ( -83.77821517812500929, -34.11562499938548854, -97.61286128772489690 ) ) ;
#14828=CARTESIAN_POINT ( 'NONE',  ( -82.40000000000000568, -30.00000000000000355, -99.99999999999998579 ) ) ;
#14829=CARTESIAN_POINT ( 'NONE',  ( 80.90000000000000568, -34.59374999877096712, -97.40192378864668399 ) ) ;
#14833=ORIENTED_EDGE ( 'NONE', *, *, #5799, .F. ) ;
#14834=CARTESIAN_POINT ( 'NONE',  ( 79.64356964374998427, -34.82812499938548711, -98.40857419181659793 ) ) ;
#14838=ORIENTED_EDGE ( 'NONE', *, *, #8397, .T. ) ;
#14839=ORIENTED_EDGE ( 'NONE', *, *, #8801, .F. ) ;
#14840=CARTESIAN_POINT ( 'NONE',  ( 80.90000000000000568, -34.35000000000000853, -102.5980762113533018 ) ) ;
#14841=VECTOR ( 'NONE', #14899, 1000.000000000000000 ) ;
#14844=ORIENTED_EDGE ( 'NONE', *, *, #15183, .F. ) ;
#14845=CARTESIAN_POINT ( 'NONE',  ( -82.85452780460292388, -35.00000000000000711, 102.7245357809972433 ) ) ;
#14848=CARTESIAN_POINT ( 'NONE',  ( -81.02178482187500208, -32.80312499938548854, 102.3871387122750889 ) ) ;
#14850=ADVANCED_FACE ( 'NONE', ( #1366 ), #9063, .F. ) ;
#14858=VERTEX_POINT ( 'NONE', #7311 ) ;
#14860=CARTESIAN_POINT ( 'NONE',  ( -82.39999999999999147, -34.07812499938548711, -96.81714838363319586 ) ) ;
#14862=PLANE ( 'NONE',  #17072 ) ;
#14868=VERTEX_POINT ( 'NONE', #13652 ) ;
#14870=CARTESIAN_POINT ( 'NONE',  ( -84.97866794691721282, -31.99999999999999289, 99.01001922939857991 ) ) ;
#14872=CARTESIAN_POINT ( 'NONE',  ( -83.90000000000000568, -32.26874999877097139, 97.40192378864668399 ) ) ;
#14873=CARTESIAN_POINT ( 'NONE',  ( 79.39999999999999147, -31.57499999999999929, 99.99999999999998579 ) ) ;
#14874=CARTESIAN_POINT ( 'NONE',  ( 83.20384757729335945, -33.45134618820330985, 96.99999999999998579 ) ) ;
#14878=VECTOR ( 'NONE', #5982, 1000.000000000000000 ) ;
#14879=CARTESIAN_POINT ( 'NONE',  ( 85.15643035625001289, -35.09062499938548285, 99.99999999999998579 ) ) ;
#14880=CARTESIAN_POINT ( 'NONE',  ( 79.64356964375001269, -30.32812499938548711, -98.40857419181659793 ) ) ;
#14884=CARTESIAN_POINT ( 'NONE',  ( 82.39999999999999147, -32.95312499938548711, -96.81714838363319586 ) ) ;
#14887=CYLINDRICAL_SURFACE ( 'NONE', #2882, 3.000000000000002665 ) ;
#14890=CARTESIAN_POINT ( 'NONE',  ( -79.39999999999999147, -31.16250000000000497, 101.7320508075688537 ) ) ;
#14892=CARTESIAN_POINT ( 'NONE',  ( -85.40000000000000568, -34.03124999877096712, 98.26794919243111792 ) ) ;
#14893=AXIS2_PLACEMENT_3D ( 'NONE', #6032, #19124, #10418 ) ;
#14895=CARTESIAN_POINT ( 'NONE',  ( 81.02178482187500208, -30.29062499938548569, 102.3871387122750889 ) ) ;
#14897=AXIS2_PLACEMENT_3D ( 'NONE', #8326, #12624, #2549 ) ;
#14899=DIRECTION ( 'NONE',  ( 0.000000000000000000, -1.000000000000000000, 0.000000000000000000 ) ) ;
#14901=CARTESIAN_POINT ( 'NONE',  ( -85.40000000000000568, -32.21250000000000568, 101.7320508075688821 ) ) ;
#14904=CARTESIAN_POINT ( 'NONE',  ( 82.39999999999999147, -33.06562499938548427, 103.1828516163667899 ) ) ;
#14907=FACE_OUTER_BOUND ( 'NONE', #8571, .T. ) ;
#14909=CARTESIAN_POINT ( 'NONE',  ( -79.64356964375001269, -31.34062499938548640, -101.5914258081833879 ) ) ;
#14911=CARTESIAN_POINT ( 'NONE',  ( 82.39999999999999147, -31.26562499938549067, 103.1828516163667899 ) ) ;
#14912=CARTESIAN_POINT ( 'NONE',  ( -94.79999999999999716, -29.80000000000000426, 150.0000000000000000 ) ) ;
#14916=AXIS2_PLACEMENT_3D ( 'NONE', #11658, #4237, #12929 ) ;
#14917=CARTESIAN_POINT ( 'NONE',  ( -82.39999999999999147, -31.71562499938548640, 96.81714838363319586 ) ) ;
#14918=CARTESIAN_POINT ( 'NONE',  ( 81.59615242270665192, -33.86115380933864571, -103.0000000000000000 ) ) ;
#14919=ORIENTED_EDGE ( 'NONE', *, *, #6263, .F. ) ;
#14920=CARTESIAN_POINT ( 'NONE',  ( -82.39999999999999147, -30.33750000000000213, -96.53589838486223584 ) ) ;
#14922=CARTESIAN_POINT ( 'NONE',  ( 85.15643035625001289, -34.75312499938548427, 99.99999999999998579 ) ) ;
#14924=CARTESIAN_POINT ( 'NONE',  ( -81.02178482187500208, -34.00312499938548427, -102.3871387122750889 ) ) ;
#14926=CARTESIAN_POINT ( 'NONE',  ( -83.90000000000000568, -32.26874999877097139, -102.5980762113533018 ) ) ;
#14929=ADVANCED_FACE ( 'NONE', ( #11998 ), #13267, .F. ) ;
#14933=CARTESIAN_POINT ( 'NONE',  ( 79.64356964374998427, -33.10312499938548569, 98.40857419181659793 ) ) ;
#14935=CARTESIAN_POINT ( 'NONE',  ( 85.40000000000000568, -33.99374999877097281, -99.99999999999998579 ) ) ;
#14945=CARTESIAN_POINT ( 'NONE',  ( -79.39999999999999147, -34.23750000000000426, -101.7320508075688963 ) ) ;
#14947=CARTESIAN_POINT ( 'NONE',  ( -81.59615242270665192, -34.81740381056767575, 103.0000000000000000 ) ) ;
#14949=CARTESIAN_POINT ( 'NONE',  ( -82.49978216248248941, -34.99999999999999289, 102.7603866155199199 ) ) ;
#14951=CARTESIAN_POINT ( 'NONE',  ( -79.64356964375001269, -33.14062499938548711, 98.40857419181659793 ) ) ;
#14957=CARTESIAN_POINT ( 'NONE',  ( -79.67114894419044901, -34.99999999999999289, -100.7768843408768760 ) ) ;
#14959=ORIENTED_EDGE ( 'NONE', *, *, #15807, .T. ) ;
#14961=CARTESIAN_POINT ( 'NONE',  ( -85.15643035624999868, -32.87812499938549138, -101.5914258081833879 ) ) ;
#14962=CARTESIAN_POINT ( 'NONE',  ( -83.90000000000000568, -33.67500000000000426, 97.40192378864668399 ) ) ;
#14963=EDGE_CURVE ( 'NONE', #13113, #13667, #3009, .T. ) ;
#14964=ADVANCED_FACE ( 'NONE', ( #16401 ), #4679, .F. ) ;
#14968=CARTESIAN_POINT ( 'NONE',  ( 85.40000000000000568, -33.14999999999999858, -99.99999999999998579 ) ) ;
#14972=DIRECTION ( 'NONE',  ( -4.625929269271494788E-16, -1.000000000000000000, 0.000000000000000000 ) ) ;
#14974=EDGE_CURVE ( 'NONE', #5649, #14237, #3200, .T. ) ;
#14975=CARTESIAN_POINT ( 'NONE',  ( -83.90000000000000568, -31.66874999877096997, 102.5980762113533018 ) ) ;
#14976=CARTESIAN_POINT ( 'NONE',  ( 82.39999999999999147, -31.91250000000000497, 103.4641016151377499 ) ) ;
#14977=LINE ( 'NONE', #10386, #4634 ) ;
#14980=CYLINDRICAL_SURFACE ( 'NONE', #7125, 3.000000000000002665 ) ;
#14981=CARTESIAN_POINT ( 'NONE',  ( 85.15643035624999868, -31.90312499938548285, -101.5914258081833879 ) ) ;
#14982=VERTEX_POINT ( 'NONE', #18159 ) ;
#14986=CARTESIAN_POINT ( 'NONE',  ( 85.15643035625001289, -32.39062499938548711, -99.99999999999998579 ) ) ;
#14987=EDGE_CURVE ( 'NONE', #13520, #13113, #855, .T. ) ;
#14989=CARTESIAN_POINT ( 'NONE',  ( 79.39999999999999147, -33.78750000000000853, -98.26794919243110371 ) ) ;
#14992=CARTESIAN_POINT ( 'NONE',  ( -85.15643035625001289, -34.64062499938548711, 99.99999999999998579 ) ) ;
#14997=DIRECTION ( 'NONE',  ( 1.000000000000000000, 0.000000000000000000, 0.000000000000000000 ) ) ;
#14999=CARTESIAN_POINT ( 'NONE',  ( -82.40000000000000568, -33.03750000000000142, -96.99999999999998579 ) ) ;
#15000=EDGE_CURVE ( 'NONE', #10326, #540, #1986, .T. ) ;
#15004=CARTESIAN_POINT ( 'NONE',  ( 85.15643035624999868, -31.56562499938548427, 98.40857419181659793 ) ) ;
#15005=CARTESIAN_POINT ( 'NONE',  ( -83.90000000000000568, -32.62500000000000000, 102.5980762113533018 ) ) ;
#15006=CARTESIAN_POINT ( 'NONE',  ( -80.90000000000000568, -32.55000000000000426, -97.40192378864668399 ) ) ;
#15007=CARTESIAN_POINT ( 'NONE',  ( -84.85729912020875076, -32.00000000000000000, -98.73859666561340021 ) ) ;
#15008=CARTESIAN_POINT ( 'NONE',  ( -85.15643035624999868, -30.66562499938548569, -98.40857419181659793 ) ) ;
#15010=CARTESIAN_POINT ( 'NONE',  ( 83.90000000000000568, -34.51874999877097139, 102.5980762113533018 ) ) ;
#15012=CARTESIAN_POINT ( 'NONE',  ( -79.68596062386970402, -32.00000000000002132, 101.2782762865727619 ) ) ;
#15013=CARTESIAN_POINT ( 'NONE',  ( -79.64356964375001269, -32.69062499938548427, 98.40857419181659793 ) ) ;
#15014=CARTESIAN_POINT ( 'NONE',  ( 81.44903907897412410, -31.99999999999999289, 102.7404298451301514 ) ) ;
#15017=CARTESIAN_POINT ( 'NONE',  ( -82.39999999999999147, -31.91250000000000497, -103.4641016151377499 ) ) ;
#15020=CARTESIAN_POINT ( 'NONE',  ( -79.64356964374999848, -34.07812499938548711, -99.99999999999998579 ) ) ;
#15025=CARTESIAN_POINT ( 'NONE',  ( -79.64356964374998427, -33.92812499938548854, -101.5914258081833879 ) ) ;
#15026=CARTESIAN_POINT ( 'NONE',  ( 79.64356964374998427, -33.47812499938547859, 101.5914258081833879 ) ) ;
#15028=CARTESIAN_POINT ( 'NONE',  ( 83.20384757729335945, -32.60759618943233562, -102.9999999999999858 ) ) ;
#15029=CARTESIAN_POINT ( 'NONE',  ( 83.90000000000000568, -33.46874999877096712, -102.5980762113533018 ) ) ;
#15040=DIRECTION ( 'NONE',  ( -0.000000000000000000, -1.000000000000000000, -0.000000000000000000 ) ) ;
#15045=CARTESIAN_POINT ( 'NONE',  ( -82.39999999999999147, -32.84062499938548996, 103.1828516163667899 ) ) ;
#15054=CARTESIAN_POINT ( 'NONE',  ( -79.64356964375001269, -34.37812499938548427, -101.5914258081833879 ) ) ;
#15059=CARTESIAN_POINT ( 'NONE',  ( -83.90000000000000568, -32.56874999877096855, 102.5980762113533018 ) ) ;
#15062=CYLINDRICAL_SURFACE ( 'NONE', #17886, 5.199999999999996625 ) ;
#15065=CARTESIAN_POINT ( 'NONE',  ( -84.93334430221554499, -32.00000000000000000, 101.1009827666099596 ) ) ;
#15067=CARTESIAN_POINT ( 'NONE',  ( -85.40000000000000568, -30.88124999877097210, 98.26794919243111792 ) ) ;
#15068=CARTESIAN_POINT ( 'NONE',  ( 82.39999999999999147, -31.01249999999999929, 103.4641016151377499 ) ) ;
#15070=AXIS2_PLACEMENT_3D ( 'NONE', #1596, #14972, #9012 ) ;
#15073=CARTESIAN_POINT ( 'NONE',  ( 81.44903907892005179, -31.99999999999999289, -97.25957015488572210 ) ) ;
#15075=CARTESIAN_POINT ( 'NONE',  ( 85.15643035625001289, -31.04062499938548569, -99.99999999999998579 ) ) ;
#15076=ORIENTED_EDGE ( 'NONE', *, *, #5603, .F. ) ;
#15078=CARTESIAN_POINT ( 'NONE',  ( -99.99999999999998579, -3.000000000000000000, 150.0000000000000000 ) ) ;
#15079=CARTESIAN_POINT ( 'NONE',  ( 81.02178482187500208, -32.99062499938548854, -97.61286128772489690 ) ) ;
#15081=ADVANCED_FACE ( 'NONE', ( #13839 ), #3486, .F. ) ;
#15085=CARTESIAN_POINT ( 'NONE',  ( -83.90000000000000568, -30.07499999999999929, 97.40192378864668399 ) ) ;
#15087=CARTESIAN_POINT ( 'NONE',  ( -84.85538848574861959, -34.99999999999998579, 98.27756861399178945 ) ) ;
#15089=CARTESIAN_POINT ( 'NONE',  ( 79.64356964374999848, -31.26562499938548356, 99.99999999999998579 ) ) ;
#15091=EDGE_CURVE ( 'NONE', #11038, #14982, #7971, .T. ) ;
#15093=EDGE_CURVE ( 'NONE', #17308, #8302, #9903, .T. ) ;
#15096=CARTESIAN_POINT ( 'NONE',  ( 85.15643035624999868, -34.71562499938548285, 98.40857419181659793 ) ) ;
#15097=EDGE_CURVE ( 'NONE', #10928, #15550, #12574, .T. ) ;
#15100=CARTESIAN_POINT ( 'NONE',  ( -84.93334430221560183, -32.00000000000000711, -98.89901723339004036 ) ) ;
#15102=ORIENTED_EDGE ( 'NONE', *, *, #17357, .T. ) ;
#15103=CARTESIAN_POINT ( 'NONE',  ( 85.40000000000000568, -34.40624999877096712, 98.26794919243111792 ) ) ;
#15104=CARTESIAN_POINT ( 'NONE',  ( 85.40000000000000568, -34.44374999877096855, 99.99999999999998579 ) ) ;
#15105=( BOUNDED_CURVE ( )  B_SPLINE_CURVE ( 2, ( #3638, #12915, #5211, #3926, #9600, #11158, #15564, #11353, #9794 ),
 .UNSPECIFIED., .F., .F. ) 
 B_SPLINE_CURVE_WITH_KNOTS ( ( 3, 2, 2, 2, 3 ),
 ( 0.6041666666666666297, 0.6111111111111111605, 0.6250000000000000000, 0.6388888888888888395, 0.6458333333333333703 ),
 .UNSPECIFIED. ) 
 CURVE ( )  GEOMETRIC_REPRESENTATION_ITEM ( )  RATIONAL_B_SPLINE_CURVE ( ( 0.9330127018922192983, 0.9330127018922187432, 1.000000000000000000, 0.8660254037844387076, 1.000000000000000000, 0.8660254037844387076, 1.000000000000000000, 0.9330127018922187432, 0.9330127018922192983 ) ) 
 REPRESENTATION_ITEM ( '' )  );
#15106=CARTESIAN_POINT ( 'NONE',  ( -82.39999999999999147, -30.81562499938548427, 96.81714838363319586 ) ) ;
#15107=DIRECTION ( 'NONE',  ( 0.000000000000000000, -1.000000000000000000, 0.000000000000000000 ) ) ;
#15108=VERTEX_POINT ( 'NONE', #9652 ) ;
#15109=CARTESIAN_POINT ( 'NONE',  ( -80.90000000000000568, -30.15000000000000213, -102.5980762113533018 ) ) ;
#15111=CARTESIAN_POINT ( 'NONE',  ( -85.40000000000000568, -34.85624999877096997, -98.26794919243111792 ) ) ;
#15112=CARTESIAN_POINT ( 'NONE',  ( -85.15643035625001289, -33.85312499938549280, -99.99999999999998579 ) ) ;
#15118=CARTESIAN_POINT ( 'NONE',  ( -83.20384757729335945, -33.45134618820330985, 102.9999999999999858 ) ) ;
#15119=CARTESIAN_POINT ( 'NONE',  ( 79.64356964374998427, -33.92812499938548854, 101.5914258081833879 ) ) ;
#15124=CARTESIAN_POINT ( 'NONE',  ( 85.40000000000000568, -34.44374999877096855, -99.99999999999998579 ) ) ;
#15131=CARTESIAN_POINT ( 'NONE',  ( -84.70388354820684640, -35.00002705695768412, 98.07851859032987818 ) ) ;
#15132=ORIENTED_EDGE ( 'NONE', *, *, #19273, .F. ) ;
#15135=CARTESIAN_POINT ( 'NONE',  ( -85.15643035625001289, -30.14062499938548711, -99.99999999999998579 ) ) ;
#15141=CARTESIAN_POINT ( 'NONE',  ( -83.77821517812500929, -34.82812499938548711, 97.61286128772489690 ) ) ;
#15150=CARTESIAN_POINT ( 'NONE',  ( -79.64356964374999848, -33.06562499938548427, -99.99999999999998579 ) ) ;
#15152=VECTOR ( 'NONE', #14798, 1000.000000000000000 ) ;
#15153=DIRECTION ( 'NONE',  ( 1.000000000000000000, 0.000000000000000000, -0.000000000000000000 ) ) ;
#15154=CARTESIAN_POINT ( 'NONE',  ( 82.39999999999999147, -33.20624999877097849, -97.00000000000000000 ) ) ;
#15159=CARTESIAN_POINT ( 'NONE',  ( 79.39999999999999147, -34.70624999877097139, 98.26794919243113213 ) ) ;
#15161=CARTESIAN_POINT ( 'NONE',  ( -80.90000000000000568, -32.49374999877097281, 102.5980762113533018 ) ) ;
#15162=CARTESIAN_POINT ( 'NONE',  ( 80.90000000000000568, -31.65000000000000568, 97.40192378864668399 ) ) ;
#15166=CARTESIAN_POINT ( 'NONE',  ( 79.64356964374999848, -33.62812499938548427, -99.99999999999998579 ) ) ;
#15168=DIRECTION ( 'NONE',  ( 0.000000000000000000, -1.000000000000000000, 0.000000000000000000 ) ) ;
#15169=CARTESIAN_POINT ( 'NONE',  ( 79.64356964375001269, -33.02812499938548285, -98.40857419181659793 ) ) ;
#15170=EDGE_LOOP ( 'NONE', ( #5349, #6148, #7700, #16358 ) ) ;
#15172=CARTESIAN_POINT ( 'NONE',  ( 82.39999999999999147, -34.07812499938548711, -103.1828516163667899 ) ) ;
#15173=CARTESIAN_POINT ( 'NONE',  ( 82.39999999999999147, -32.72812499938548569, -103.1828516163667899 ) ) ;
#15178=CARTESIAN_POINT ( 'NONE',  ( -82.39999999999999147, -34.97812499938547859, 103.1828516163667899 ) ) ;
#15181=CARTESIAN_POINT ( 'NONE',  ( 85.15643035625001289, -30.59062499938548285, 99.99999999999998579 ) ) ;
#15183=EDGE_CURVE ( 'NONE', #15647, #6543, #19116, .T. ) ;
#15186=AXIS2_PLACEMENT_3D ( 'NONE', #5953, #12190, #8967 ) ;
#15188=CARTESIAN_POINT ( 'NONE',  ( 85.15643035624999868, -35.22676555956768141, 101.0032586025029815 ) ) ;
#15189=CARTESIAN_POINT ( 'NONE',  ( 79.64356964375001269, -30.96562499938548640, -101.5914258081833879 ) ) ;
#15192=CARTESIAN_POINT ( 'NONE',  ( -85.15643035625001289, -32.50312499938548427, -99.99999999999998579 ) ) ;
#15193=ORIENTED_EDGE ( 'NONE', *, *, #695, .T. ) ;
#15194=CARTESIAN_POINT ( 'NONE',  ( 83.90000000000000568, -34.36874999877097281, 97.40192378864668399 ) ) ;
#15199=CARTESIAN_POINT ( 'NONE',  ( -82.39999999999999147, -32.39062499938548001, 103.1828516163667899 ) ) ;
#15200=CARTESIAN_POINT ( 'NONE',  ( 82.40000000000000568, -30.00000000000000355, -96.99999999999998579 ) ) ;
#15202=CARTESIAN_POINT ( 'NONE',  ( -80.90000000000000568, -32.10000000000000142, -97.40192378864668399 ) ) ;
#15204=COLOUR_RGB ( '',0.8941176470588234615, 0.8941176470588234615, 0.8941176470588234615 ) ;
#15205=CARTESIAN_POINT ( 'NONE',  ( 85.40000000000000568, -34.53750000000000142, -98.26794919243111792 ) ) ;
#15207=CARTESIAN_POINT ( 'NONE',  ( 79.68596062386910717, -31.99999999999998579, -101.2782762865714972 ) ) ;
#15212=( GEOMETRIC_REPRESENTATION_CONTEXT ( 3 ) GLOBAL_UNCERTAINTY_ASSIGNED_CONTEXT ( ( #14274 ) ) GLOBAL_UNIT_ASSIGNED_CONTEXT ( ( #533, #5319, #11259 ) ) REPRESENTATION_CONTEXT ( 'NONE', 'WORKASPACE' ) );
#15215=CARTESIAN_POINT ( 'NONE',  ( 85.40000000000000568, -32.28750000000000142, 101.7320508075688821 ) ) ;
#15216=CARTESIAN_POINT ( 'NONE',  ( 81.02178482187500208, -32.99062499938548854, 102.3871387122750889 ) ) ;
#15217=CARTESIAN_POINT ( 'NONE',  ( 82.40000000000000568, -34.55624999877097281, -97.00000000000000000 ) ) ;
#15219=CARTESIAN_POINT ( 'NONE',  ( 85.40000000000000568, -34.48124999877096997, -98.26794919243111792 ) ) ;
#15222=( BOUNDED_CURVE ( )  B_SPLINE_CURVE ( 2, ( #10398, #16557, #10210, #3158, #1700, #1416, #4250, #154, #6105 ),
 .UNSPECIFIED., .F., .F. ) 
 B_SPLINE_CURVE_WITH_KNOTS ( ( 3, 2, 2, 2, 3 ),
 ( 0.7708333333333331483, 0.7777777777777777901, 0.7916666666666666297, 0.8055555555555555802, 0.8125000000000001110 ),
 .UNSPECIFIED. ) 
 CURVE ( )  GEOMETRIC_REPRESENTATION_ITEM ( )  RATIONAL_B_SPLINE_CURVE ( ( 0.9330127018922194093, 0.9330127018922177440, 1.000000000000000000, 0.8660254037844387076, 1.000000000000000000, 0.8660254037844387076, 1.000000000000000000, 0.9330127018922182991, 0.9330127018922194093 ) ) 
 REPRESENTATION_ITEM ( '' )  );
#15224=ORIENTED_EDGE ( 'NONE', *, *, #17977, .T. ) ;
#15231=ORIENTED_EDGE ( 'NONE', *, *, #1234, .F. ) ;
#15233=CARTESIAN_POINT ( 'NONE',  ( -79.64356964374999848, -30.36562499938548498, -99.99999999999998579 ) ) ;
#15235=CARTESIAN_POINT ( 'NONE',  ( -83.20384757729335945, -34.14240381056767148, -102.9999999999999716 ) ) ;
#15236=EDGE_LOOP ( 'NONE', ( #7206, #13869, #19027, #2064 ) ) ;
#15239=AXIS2_PLACEMENT_3D ( 'NONE', #17675, #7982, #13938 ) ;
#15244=DIRECTION ( 'NONE',  ( -1.000000000000000000, 0.000000000000000000, 0.000000000000000000 ) ) ;
#15247=CARTESIAN_POINT ( 'NONE',  ( -80.90000000000000568, -33.30000000000000426, 97.40192378864668399 ) ) ;
#15252=CARTESIAN_POINT ( 'NONE',  ( -85.15643035625001289, -33.74062499938548854, -99.99999999999998579 ) ) ;
#15257=CARTESIAN_POINT ( 'NONE',  ( -94.79999999999999716, -29.80000000000000426, -150.0000000000000000 ) ) ;
#15259=ORIENTED_EDGE ( 'NONE', *, *, #4094, .T. ) ;
#15260=CARTESIAN_POINT ( 'NONE',  ( -83.52979456739217312, -32.00000000000000000, 102.5803447510192257 ) ) ;
#15261=CARTESIAN_POINT ( 'NONE',  ( 79.39999999999999147, -30.67500000000000071, -99.99999999999998579 ) ) ;
#15262=CARTESIAN_POINT ( 'NONE',  ( -79.39999999999999147, -33.73124999877096997, 98.26794919243110371 ) ) ;
#15264=CARTESIAN_POINT ( 'NONE',  ( -81.45486068924901701, -32.00000000000002132, -97.24663084804292623 ) ) ;
#15266=CARTESIAN_POINT ( 'NONE',  ( 83.77821517812500929, -33.32812499938548711, -102.3871387122750889 ) ) ;
#15267=CARTESIAN_POINT ( 'NONE',  ( 79.39999999999999147, -33.37500000000000000, -99.99999999999998579 ) ) ;
#15268=CARTESIAN_POINT ( 'NONE',  ( 79.64356964374999848, -33.06562499938548427, -99.99999999999998579 ) ) ;
#15269=ORIENTED_EDGE ( 'NONE', *, *, #11638, .T. ) ;
#15272=CARTESIAN_POINT ( 'NONE',  ( -79.39999999999999147, -34.76250000000000284, 101.7320508075688537 ) ) ;
#15274=UNCERTAINTY_MEASURE_WITH_UNIT (LENGTH_MEASURE( 1.000000000000000082E-05 ), #16243, 'distance_accuracy_value', 'NONE');
#15278=CARTESIAN_POINT ( 'NONE',  ( -79.39999999999999147, -30.18750000000000355, 98.26794919243110371 ) ) ;
#15279=EDGE_LOOP ( 'NONE', ( #1569, #4687, #17765, #15424 ) ) ;
#15286=CARTESIAN_POINT ( 'NONE',  ( 81.02178482187500208, -34.60312499938549280, 97.61286128772489690 ) ) ;
#15287=CARTESIAN_POINT ( 'NONE',  ( 82.39999999999999147, -31.71562499938548640, -96.81714838363319586 ) ) ;
#15289=CARTESIAN_POINT ( 'NONE',  ( -83.77821517812500929, -34.67812499938548854, 102.3871387122750889 ) ) ;
#15290=CARTESIAN_POINT ( 'NONE',  ( -83.77821517812500929, -33.92812499938548854, -102.3871387122750889 ) ) ;
#15292=ORIENTED_EDGE ( 'NONE', *, *, #4624, .F. ) ;
#15293=CARTESIAN_POINT ( 'NONE',  ( 79.64356964375001269, -33.21562499938548996, 98.40857419181659793 ) ) ;
#15295=CARTESIAN_POINT ( 'NONE',  ( 82.40000000000000568, -30.00000000000000355, -99.99999999999998579 ) ) ;
#15296=CARTESIAN_POINT ( 'NONE',  ( -83.77821517812500929, -33.32812499938548711, 102.3871387122750889 ) ) ;
#15297=( BOUNDED_CURVE ( )  B_SPLINE_CURVE ( 2, ( #12810, #5401, #8126, #11344, #8410, #12613, #18586 ),
 .UNSPECIFIED., .F., .F. ) 
 B_SPLINE_CURVE_WITH_KNOTS ( ( 3, 2, 2, 3 ),
 ( 0.3702305174533203069, 0.3750000000000000000, 0.3888888888888888951, 0.3958333333333334259 ),
 .UNSPECIFIED. ) 
 CURVE ( )  GEOMETRIC_REPRESENTATION_ITEM ( )  RATIONAL_B_SPLINE_CURVE ( ( 0.9395835397642939846, 0.9539927561189023297, 1.000000000000000000, 0.8660254037844387076, 1.000000000000000000, 0.9330127018922185211, 0.9330127018922192983 ) ) 
 REPRESENTATION_ITEM ( '' )  );
#15298=DIRECTION ( 'NONE',  ( 0.000000000000000000, 0.000000000000000000, -1.000000000000000000 ) ) ;
#15299=ORIENTED_EDGE ( 'NONE', *, *, #10593, .T. ) ;
#15300=CARTESIAN_POINT ( 'NONE',  ( -85.40000000000000568, -31.38749999999999574, -101.7320508075688679 ) ) ;
#15303=CARTESIAN_POINT ( 'NONE',  ( 82.40000000000000568, -30.00000000000000355, -99.99999999999998579 ) ) ;
#15307=VERTEX_POINT ( 'NONE', #962 ) ;
#15309=CARTESIAN_POINT ( 'NONE',  ( 82.40000000000000568, -34.38749999999999574, -102.9999999999999858 ) ) ;
#15311=DIRECTION ( 'NONE',  ( -1.000000000000000000, 0.000000000000000000, 0.000000000000000000 ) ) ;
#15312=CARTESIAN_POINT ( 'NONE',  ( 94.79999999999995453, -5.200000000000000178, 150.0000000000000000 ) ) ;
#15313=CARTESIAN_POINT ( 'NONE',  ( 82.39999999999999147, -30.81562499938548427, -96.81714838363319586 ) ) ;
#15314=CARTESIAN_POINT ( 'NONE',  ( -82.39999999999999147, -32.36250000000000426, 96.99999999999998579 ) ) ;
#15324=CARTESIAN_POINT ( 'NONE',  ( -79.68063642056705476, -32.00000000000000711, 98.73478688818576643 ) ) ;
#15325=CARTESIAN_POINT ( 'NONE',  ( -80.90000000000000568, -33.84374999877096712, -97.40192378864668399 ) ) ;
#15326=CARTESIAN_POINT ( 'NONE',  ( 82.40000000000000568, -30.00000000000000355, -96.99999999999998579 ) ) ;
#15327=VERTEX_POINT ( 'NONE', #4073 ) ;
#15329=CARTESIAN_POINT ( 'NONE',  ( -80.90000000000000568, -34.59374999877096712, -102.5980762113533018 ) ) ;
#15334=( BOUNDED_CURVE ( )  B_SPLINE_CURVE ( 2, ( #5064, #14038, #1736, #7887, #4974, #16881, #18158, #15509, #15217 ),
 .UNSPECIFIED., .F., .F. ) 
 B_SPLINE_CURVE_WITH_KNOTS ( ( 3, 2, 2, 2, 3 ),
 ( 0.7291666666666666297, 0.7361111111111111605, 0.7500000000000000000, 0.7638888888888888395, 0.7708333333333331483 ),
 .UNSPECIFIED. ) 
 CURVE ( )  GEOMETRIC_REPRESENTATION_ITEM ( )  RATIONAL_B_SPLINE_CURVE ( ( 0.9330127018922192983, 0.9330127018922187432, 1.000000000000000000, 0.8660254037844387076, 1.000000000000000000, 0.8660254037844387076, 1.000000000000000000, 0.9330127018922209636, 0.9330127018922194093 ) ) 
 REPRESENTATION_ITEM ( '' )  );
#15343=CARTESIAN_POINT ( 'NONE',  ( -83.77821517812500929, -35.01562499938548711, -97.61286128772489690 ) ) ;
#15348=CARTESIAN_POINT ( 'NONE',  ( 80.90000000000000568, -33.45000000000000284, 97.40192378864668399 ) ) ;
#15349=VERTEX_POINT ( 'NONE', #5551 ) ;
#15350=FACE_OUTER_BOUND ( 'NONE', #4329, .T. ) ;
#15351=AXIS2_PLACEMENT_3D ( 'NONE', #6546, #3503, #9462 ) ;
#15354=CARTESIAN_POINT ( 'NONE',  ( -81.45486068924900280, -32.00000000000002132, 102.7533691519570311 ) ) ;
#15355=EDGE_CURVE ( 'NONE', #17378, #10782, #14508, .T. ) ;
#15356=CARTESIAN_POINT ( 'NONE',  ( 85.40000000000000568, -30.45000000000000284, -99.99999999999998579 ) ) ;
#15357=DIRECTION ( 'NONE',  ( 0.000000000000000000, -1.000000000000000000, 0.000000000000000000 ) ) ;
#15358=CARTESIAN_POINT ( 'NONE',  ( -84.69813954184694182, -35.39427337414329600, 98.07164457472185859 ) ) ;
#15359=CARTESIAN_POINT ( 'NONE',  ( -94.79999999999999716, -29.80000000000000426, -150.0000000000000000 ) ) ;
#15361=CARTESIAN_POINT ( 'NONE',  ( 85.15643035625001289, -32.91562499938548569, -101.5914258081833879 ) ) ;
#15363=CARTESIAN_POINT ( 'NONE',  ( -81.02178482187500208, -33.44062499938548427, 97.61286128772489690 ) ) ;
#15366=CARTESIAN_POINT ( 'NONE',  ( 85.15643035624999868, -32.87812499938549138, -98.40857419181659793 ) ) ;
#15367=ORIENTED_EDGE ( 'NONE', *, *, #18843, .F. ) ;
#15370=CARTESIAN_POINT ( 'NONE',  ( -82.39999999999999147, -34.83749999999999858, 103.4641016151377499 ) ) ;
#15375=CARTESIAN_POINT ( 'NONE',  ( -85.40000000000000568, -32.66250000000000142, 101.7320508075688679 ) ) ;
#15381=CARTESIAN_POINT ( 'NONE',  ( 82.39999999999999147, -31.60312499938548569, 103.1828516163667899 ) ) ;
#15383=CARTESIAN_POINT ( 'NONE',  ( 85.40000000000000568, -32.68124999877097281, -98.26794919243111792 ) ) ;
#15386=CARTESIAN_POINT ( 'NONE',  ( -85.15643035624999868, -32.02817623523066004, -98.94122380911285575 ) ) ;
#15387=CARTESIAN_POINT ( 'NONE',  ( 81.02178482187500208, -35.05312499938548854, 97.61286128772489690 ) ) ;
#15389=CARTESIAN_POINT ( 'NONE',  ( 83.77821517812500929, -31.67812499938548498, -97.61286128772489690 ) ) ;
#15391=CARTESIAN_POINT ( 'NONE',  ( -83.77821517812500929, -33.47812499938548569, 97.61286128772489690 ) ) ;
#15392=CARTESIAN_POINT ( 'NONE',  ( -81.02178482187500208, -33.70312499938548711, -97.61286128772489690 ) ) ;
#15394=ORIENTED_EDGE ( 'NONE', *, *, #14987, .T. ) ;
#15395=CARTESIAN_POINT ( 'NONE',  ( 85.15643035624999868, -33.89062499938548711, 101.5914258081833879 ) ) ;
#15397=CARTESIAN_POINT ( 'NONE',  ( -83.77821517812500929, -31.11562499938548498, 97.61286128772489690 ) ) ;
#15398=CARTESIAN_POINT ( 'NONE',  ( -81.02178482187500208, -34.00312499938548427, 97.61286128772489690 ) ) ;
#15399=CARTESIAN_POINT ( 'NONE',  ( 85.40000000000000568, -33.13124999877096855, 101.7320508075688821 ) ) ;
#15400=EDGE_LOOP ( 'NONE', ( #1703, #13582, #468, #17593 ) ) ;
#15401=CARTESIAN_POINT ( 'NONE',  ( -79.39999999999999147, -34.68750000000000000, -101.7320508075688821 ) ) ;
#15404=CARTESIAN_POINT ( 'NONE',  ( -85.15643035625001289, -34.75312499938548427, -99.99999999999998579 ) ) ;
#15408=FACE_OUTER_BOUND ( 'NONE', #15236, .T. ) ;
#15409=CARTESIAN_POINT ( 'NONE',  ( 82.39999999999999147, -32.98124999877096286, -102.9999999999999858 ) ) ;
#15413=CARTESIAN_POINT ( 'NONE',  ( 82.39999999999999147, -32.39062499938548001, -103.1828516163667899 ) ) ;
#15416=ORIENTED_EDGE ( 'NONE', *, *, #11528, .T. ) ;
#15417=CARTESIAN_POINT ( 'NONE',  ( 83.90000000000000568, -30.76874999877097139, 97.40192378864668399 ) ) ;
#15423=ORIENTED_EDGE ( 'NONE', *, *, #17238, .T. ) ;
#15424=ORIENTED_EDGE ( 'NONE', *, *, #18568, .F. ) ;
#15426=CARTESIAN_POINT ( 'NONE',  ( -82.40000000000001990, -32.13750000000000284, -97.00000000000000000 ) ) ;
#15428=ORIENTED_EDGE ( 'NONE', *, *, #6731, .T. ) ;
#15429=CARTESIAN_POINT ( 'NONE',  ( 79.64356964374999848, -32.27812499938548996, 99.99999999999998579 ) ) ;
#15430=CARTESIAN_POINT ( 'NONE',  ( -85.40000000000000568, -34.89374999877097139, -99.99999999999998579 ) ) ;
#15435=EDGE_CURVE ( 'NONE', #5530, #7316, #1250, .T. ) ;
#15436=ADVANCED_FACE ( 'NONE', ( #14803 ), #17756, .F. ) ;
#15437=CARTESIAN_POINT ( 'NONE',  ( 79.39999999999999147, -34.18124999877097281, -98.26794919243110371 ) ) ;
#15441=CARTESIAN_POINT ( 'NONE',  ( -79.64356964375001269, -34.90312499938548285, -98.40857419181659793 ) ) ;
#15445=CARTESIAN_POINT ( 'NONE',  ( 82.39999999999999147, -33.48750000000000426, 97.00000000000000000 ) ) ;
#15449=DIRECTION ( 'NONE',  ( -0.000000000000000000, -0.000000000000000000, -1.000000000000000000 ) ) ;
#15450=EDGE_CURVE ( 'NONE', #16850, #13270, #3234, .T. ) ;
#15453=ADVANCED_FACE ( 'NONE', ( #5831 ), #16281, .F. ) ;
#15455=CARTESIAN_POINT ( 'NONE',  ( -79.93183330737464587, -32.00000000000002132, 101.6855250459192206 ) ) ;
#15456=CARTESIAN_POINT ( 'NONE',  ( 85.40000000000000568, -31.31250000000000000, -101.7320508075688679 ) ) ;
#15457=DIRECTION ( 'NONE',  ( -0.000000000000000000, -1.000000000000000000, -0.000000000000000000 ) ) ;
#15459=( BOUNDED_SURFACE ( )  B_SPLINE_SURFACE ( 1, 2, ( 
 ( #12957, #5261, #15611, #17461, #12865, #4072, #10032, #2595, #2309, #11207, #8273, #8555, #14223, #861, #5156, #11102, #17070, #2406, #14128, #9651, #8181, #18836, #6824, #766, #6719, #12664, #18739, #17268, #9837, #11301, #15801, #19115, #7482, #11781, #19317, #15004, #13438, #8650, #17841, #14802, #10320, #1532, #1429, #7382, #4455, #4550, #17755, #11684, #13342, #5928, #11874, #4360, #4264, #19022, #5735, #1622, #10223, #16280, #10410, #16374, #19213, #17554, #69, #10507, #2982, #8938, #2693, #17651, #13056, #13240, #6022, #16189, #5830, #2797, #11971, #14904, #17939, #3079, #5643, #8750, #11589, #14702, #2890, #16474, #9039, #8846, #4170, #10129, #16087, #14609, #1240, #7192, #1339, #13141, #7286, #549, #6219, #7769, #264, #13911, #12358, #7957, #16950, #4655, #10791, #7863, #13814, #1711, #18419, #12166, #3461, #18133, #18230, #4753, #6507, #10697, #15286, #4944, #6405, #15096, #15485, #1901, #9223, #16857, #166, #6311, #13528, #9420, #15387, #456, #16663, #13622, #3267, #15188, #1805 ),
 ( #2000, #12452, #18327, #5039, #7666, #7575, #3562, #10889, #10981, #9521, #6117, #12069, #18044, #10605, #16571, #3172, #9132, #13722, #363, #12265, #4846, #16753, #3370, #9322, #15682, #17339, #5134, #3848, #18517, #8252, #9814, #8439, #6698, #12642, #742, #15877, #2098, #6801, #18810, #8154, #11079, #11182, #5234, #14391, #17244, #18616, #1030, #14013, #2384, #9718, #17048, #8346, #17146, #649, #6982, #3660, #6892, #3949, #15586, #11473, #2196, #9625, #3752, #2288, #15776, #5435, #14106, #937, #9914, #14301, #2481, #14202, #839, #11372, #12842, #12934, #18904, #5525, #12748, #18715, #5338, #17440, #11275, #4051, #10010, #8058, #6598, #12546, #11569, #17820, #13032, #10299, #11664, #46, #4430, #5623, #2962, #14682, #1316, #17627, #14582, #2667, #10390, #7265, #2867, #17919, #16351, #17532, #1408, #17730, #13219, #8917, #4339, #16259, #7361, #7458, #19192, #1217, #8826, #14782, #13317, #5807, #7173, #2573, #8628, #4527, #13123, #11758, #19293, #5906, #2773, #1116, #14879, #13416, #11852 ) ),
 .UNSPECIFIED., .F., .F., .F. ) 
 B_SPLINE_SURFACE_WITH_KNOTS ( ( 2, 2 ),
 ( 3, 2, 2, 2, 2, 2, 2, 2, 2, 2, 2, 2, 2, 2, 2, 2, 2, 2, 2, 2, 2, 2, 2, 2, 2, 2, 2, 2, 2, 2, 2, 2, 2, 2, 2, 2, 2, 2, 2, 2, 2, 2, 2, 2, 2, 2, 2, 2, 2, 2, 2, 2, 2, 2, 2, 2, 2, 2, 2, 2, 2, 2, 2, 2, 2, 2, 2, 3 ),
 ( 0.000000000000000000, 1.000000000000000000 ),
 ( 0.000000000000000000, 0.01388888888888888812, 0.02777777777777777624, 0.04166666666666666435, 0.05555555555555555247, 0.06944444444444444753, 0.08333333333333332871, 0.09722222222222222376, 0.1111111111111111049, 0.1250000000000000000, 0.1388888888888888951, 0.1527777777777777901, 0.1666666666666666574, 0.1805555555555555525, 0.1944444444444444475, 0.2083333333333333426, 0.2222222222222222099, 0.2361111111111111049, 0.2500000000000000000, 0.2638888888888888951, 0.2777777777777777901, 0.2916666666666666852, 0.3055555555555555802, 0.3194444444444444198, 0.3333333333333333148, 0.3472222222222222099, 0.3611111111111111049, 0.3750000000000000000, 0.3888888888888888951, 0.4027777777777777901, 0.4166666666666666852, 0.4305555555555555802, 0.4444444444444444198, 0.4583333333333333148, 0.4722222222222222099, 0.4861111111111111049, 0.5000000000000000000, 0.5138888888888888395, 0.5277777777777777901, 0.5416666666666666297, 0.5555555555555555802, 0.5694444444444444198, 0.5833333333333333703, 0.5972222222222222099, 0.6111111111111111605, 0.6250000000000000000, 0.6388888888888888395, 0.6527777777777777901, 0.6666666666666666297, 0.6805555555555555802, 0.6944444444444444198, 0.7083333333333333703, 0.7222222222222222099, 0.7361111111111111605, 0.7500000000000000000, 0.7638888888888888395, 0.7777777777777777901, 0.7916666666666666297, 0.8055555555555555802, 0.8194444444444444198, 0.8333333333333333703, 0.8472222222222222099, 0.8611111111111111605, 0.8750000000000000000, 0.8888888888888888395, 0.9027777777777777901, 0.9166666666666666297, 0.9258785565094813652 ),
 .UNSPECIFIED. ) 
 GEOMETRIC_REPRESENTATION_ITEM ( )  RATIONAL_B_SPLINE_SURFACE ( (
 ( 1.000000000000000000, 0.8660254037844387076, 1.000000000000000000, 0.8660254037844387076, 1.000000000000000000, 0.8660254037844387076, 1.000000000000000000, 0.8660254037844387076, 1.000000000000000000, 0.8660254037844387076, 1.000000000000000000, 0.8660254037844387076, 1.000000000000000000, 0.8660254037844387076, 1.000000000000000000, 0.8660254037844387076, 1.000000000000000000, 0.8660254037844387076, 1.000000000000000000, 0.8660254037844387076, 1.000000000000000000, 0.8660254037844387076, 1.000000000000000000, 0.8660254037844387076, 1.000000000000000000, 0.8660254037844387076, 1.000000000000000000, 0.8660254037844387076, 1.000000000000000000, 0.8660254037844387076, 1.000000000000000000, 0.8660254037844387076, 1.000000000000000000, 0.8660254037844387076, 1.000000000000000000, 0.8660254037844387076, 1.000000000000000000, 0.8660254037844387076, 1.000000000000000000, 0.8660254037844387076, 1.000000000000000000, 0.8660254037844387076, 1.000000000000000000, 0.8660254037844387076, 1.000000000000000000, 0.8660254037844387076, 1.000000000000000000, 0.8660254037844387076, 1.000000000000000000, 0.8660254037844387076, 1.000000000000000000, 0.8660254037844387076, 1.000000000000000000, 0.8660254037844387076, 1.000000000000000000, 0.8660254037844387076, 1.000000000000000000, 0.8660254037844387076, 1.000000000000000000, 0.8660254037844387076, 1.000000000000000000, 0.8660254037844387076, 1.000000000000000000, 0.8660254037844387076, 1.000000000000000000, 0.8660254037844387076, 1.000000000000000000, 0.8660254037844387076, 1.000000000000000000, 0.8660254037844387076, 1.000000000000000000, 0.8660254037844387076, 1.000000000000000000, 0.8660254037844387076, 1.000000000000000000, 0.8660254037844387076, 1.000000000000000000, 0.8660254037844387076, 1.000000000000000000, 0.8660254037844387076, 1.000000000000000000, 0.8660254037844387076, 1.000000000000000000, 0.8660254037844387076, 1.000000000000000000, 0.8660254037844387076, 1.000000000000000000, 0.8660254037844387076, 1.000000000000000000, 0.8660254037844387076, 1.000000000000000000, 0.8660254037844387076, 1.000000000000000000, 0.8660254037844387076, 1.000000000000000000, 0.8660254037844387076, 1.000000000000000000, 0.8660254037844387076, 1.000000000000000000, 0.8660254037844387076, 1.000000000000000000, 0.8660254037844387076, 1.000000000000000000, 0.8660254037844387076, 1.000000000000000000, 0.8660254037844387076, 1.000000000000000000, 0.8660254037844387076, 1.000000000000000000, 0.8660254037844387076, 1.000000000000000000, 0.8660254037844387076, 1.000000000000000000, 0.8660254037844387076, 1.000000000000000000, 0.8660254037844387076, 1.000000000000000000, 0.8660254037844387076, 1.000000000000000000, 0.8660254037844387076, 1.000000000000000000, 0.8660254037844387076, 1.000000000000000000, 0.8660254037844387076, 1.000000000000000000, 0.8660254037844387076, 1.000000000000000000, 0.8660254037844387076, 1.000000000000000000, 0.8660254037844387076, 1.000000000000000000, 0.8660254037844387076, 1.000000000000000000, 0.9111405360107203144, 0.9401542295229963209),
 ( 1.000000000000000000, 0.8660254037844387076, 1.000000000000000000, 0.8660254037844387076, 1.000000000000000000, 0.8660254037844387076, 1.000000000000000000, 0.8660254037844387076, 1.000000000000000000, 0.8660254037844387076, 1.000000000000000000, 0.8660254037844387076, 1.000000000000000000, 0.8660254037844387076, 1.000000000000000000, 0.8660254037844387076, 1.000000000000000000, 0.8660254037844387076, 1.000000000000000000, 0.8660254037844387076, 1.000000000000000000, 0.8660254037844387076, 1.000000000000000000, 0.8660254037844387076, 1.000000000000000000, 0.8660254037844387076, 1.000000000000000000, 0.8660254037844387076, 1.000000000000000000, 0.8660254037844387076, 1.000000000000000000, 0.8660254037844387076, 1.000000000000000000, 0.8660254037844387076, 1.000000000000000000, 0.8660254037844387076, 1.000000000000000000, 0.8660254037844387076, 1.000000000000000000, 0.8660254037844387076, 1.000000000000000000, 0.8660254037844387076, 1.000000000000000000, 0.8660254037844387076, 1.000000000000000000, 0.8660254037844387076, 1.000000000000000000, 0.8660254037844387076, 1.000000000000000000, 0.8660254037844387076, 1.000000000000000000, 0.8660254037844387076, 1.000000000000000000, 0.8660254037844387076, 1.000000000000000000, 0.8660254037844387076, 1.000000000000000000, 0.8660254037844387076, 1.000000000000000000, 0.8660254037844387076, 1.000000000000000000, 0.8660254037844387076, 1.000000000000000000, 0.8660254037844387076, 1.000000000000000000, 0.8660254037844387076, 1.000000000000000000, 0.8660254037844387076, 1.000000000000000000, 0.8660254037844387076, 1.000000000000000000, 0.8660254037844387076, 1.000000000000000000, 0.8660254037844387076, 1.000000000000000000, 0.8660254037844387076, 1.000000000000000000, 0.8660254037844387076, 1.000000000000000000, 0.8660254037844387076, 1.000000000000000000, 0.8660254037844387076, 1.000000000000000000, 0.8660254037844387076, 1.000000000000000000, 0.8660254037844387076, 1.000000000000000000, 0.8660254037844387076, 1.000000000000000000, 0.8660254037844387076, 1.000000000000000000, 0.8660254037844387076, 1.000000000000000000, 0.8660254037844387076, 1.000000000000000000, 0.8660254037844387076, 1.000000000000000000, 0.8660254037844387076, 1.000000000000000000, 0.8660254037844387076, 1.000000000000000000, 0.8660254037844387076, 1.000000000000000000, 0.8660254037844387076, 1.000000000000000000, 0.8660254037844387076, 1.000000000000000000, 0.8660254037844387076, 1.000000000000000000, 0.8660254037844387076, 1.000000000000000000, 0.8660254037844387076, 1.000000000000000000, 0.8660254037844387076, 1.000000000000000000, 0.8660254037844387076, 1.000000000000000000, 0.8660254037844387076, 1.000000000000000000, 0.8660254037844387076, 1.000000000000000000, 0.8660254037844387076, 1.000000000000000000, 0.8660254037844387076, 1.000000000000000000, 0.8660254037844387076, 1.000000000000000000, 0.8660254037844387076, 1.000000000000000000, 0.8660254037844387076, 1.000000000000000000, 0.8660254037844387076, 1.000000000000000000, 0.9111405360107203144, 0.9401542295229963209) ) ) 
 REPRESENTATION_ITEM ( '' )  SURFACE ( )  );
#15460=CARTESIAN_POINT ( 'NONE',  ( -85.40000000000000568, -33.54374999877096286, 99.99999999999998579 ) ) ;
#15462=CARTESIAN_POINT ( 'NONE',  ( -82.40000000000000568, -32.08124999877097139, -97.00000000000000000 ) ) ;
#15463=DIRECTION ( 'NONE',  ( 0.000000000000000000, -1.000000000000000000, 0.000000000000000000 ) ) ;
#15464=CARTESIAN_POINT ( 'NONE',  ( 79.64356964374998427, -32.69062499938548427, -98.40857419181659793 ) ) ;
#15465=CARTESIAN_POINT ( 'NONE',  ( 79.39999999999999147, -33.78750000000000853, 101.7320508075688963 ) ) ;
#15466=CARTESIAN_POINT ( 'NONE',  ( -79.64356964375001269, -34.00312499938549138, 101.5914258081833879 ) ) ;
#15468=CARTESIAN_POINT ( 'NONE',  ( 85.15643035625001289, -33.29062499938547859, -99.99999999999998579 ) ) ;
#15471=CARTESIAN_POINT ( 'NONE',  ( -82.39999999999999147, -33.93750000000000000, 103.4641016151377499 ) ) ;
#15476=CARTESIAN_POINT ( 'NONE',  ( -85.40000000000000568, -31.76249999999999929, 101.7320508075688679 ) ) ;
#15477=ORIENTED_EDGE ( 'NONE', *, *, #8517, .F. ) ;
#15478=CARTESIAN_POINT ( 'NONE',  ( -79.77811200999879304, -35.00000000000000000, -99.14934632385212865 ) ) ;
#15481=CARTESIAN_POINT ( 'NONE',  ( 79.64356964375001269, -32.65312499938548285, 98.40857419181659793 ) ) ;
#15484=DIRECTION ( 'NONE',  ( 1.000000000000000000, 0.000000000000000000, 0.000000000000000000 ) ) ;
#15485=CARTESIAN_POINT ( 'NONE',  ( 85.15643035625001289, -34.75312499938548427, 99.99999999999998579 ) ) ;
#15487=CARTESIAN_POINT ( 'NONE',  ( 79.64356964375001269, -32.76562499938548711, -101.5914258081833879 ) ) ;
#15488=EDGE_CURVE ( 'NONE', #4491, #8584, #7383, .T. ) ;
#15490=CARTESIAN_POINT ( 'NONE',  ( -85.15643035625001289, -34.79062499938548569, 98.40857419181659793 ) ) ;
#15491=CARTESIAN_POINT ( 'NONE',  ( -81.02178482187500208, -33.55312499938548854, -102.3871387122750889 ) ) ;
#15493=CARTESIAN_POINT ( 'NONE',  ( 85.15643035625001289, -32.95312499938548711, 99.99999999999998579 ) ) ;
#15495=CARTESIAN_POINT ( 'NONE',  ( -83.77821517812500929, -30.51562499938548711, 102.3871387122750889 ) ) ;
#15496=CARTESIAN_POINT ( 'NONE',  ( -85.15643035624999868, -35.22676555956768141, 98.99674139749697588 ) ) ;
#15499=CARTESIAN_POINT ( 'NONE',  ( -83.90000000000000568, -33.07500000000000284, -97.40192378864668399 ) ) ;
#15503=CARTESIAN_POINT ( 'NONE',  ( -85.15643035625001289, -35.22676544108147567, -101.0032535741825654 ) ) ;
#15507=CARTESIAN_POINT ( 'NONE',  ( 99.99999999999994316, -32.00000000000000000, -150.0000000000000000 ) ) ;
#15509=CARTESIAN_POINT ( 'NONE',  ( 83.20384757729338787, -34.53615380933862866, -97.00000000000000000 ) ) ;
#15510=( BOUNDED_CURVE ( )  B_SPLINE_CURVE ( 2, ( #4190, #10150, #4000, #7214, #5576, #17293, #19139, #1267, #5380, #9767, #3798, #3897, #2720, #15825, #5668, #12982, #18761, #887, #14534, #16112, #7126, #2435, #12888, #13078, #15729, #18953, #14344, #1071, #982, #19044, #8680, #11523, #4093, #7028, #10055, #6937, #11425, #18859, #14632, #16015, #8480, #5479, #17386, #14248, #6847, #13168, #2523, #5756, #17194, #12792, #9964, #15918, #6141, #15025, #10626, #291, #17777, #7405, #14825, #10252, #14727, #8867, #5950, #1645, #16214, #1363, #11897, #13551, #17963, #19238, #11706, #191, #4573, #1452, #4384, #2915, #10341, #16305, #17674, #10531, #13368, #1734, #12092 ),
 .UNSPECIFIED., .F., .F. ) 
 B_SPLINE_CURVE_WITH_KNOTS ( ( 3, 2, 2, 2, 2, 2, 2, 2, 2, 2, 2, 2, 2, 2, 2, 2, 2, 2, 2, 2, 2, 2, 2, 2, 2, 2, 2, 2, 2, 2, 2, 2, 2, 2, 2, 2, 2, 2, 2, 2, 2, 3 ),
 ( 0.3716916592826018384, 0.3750191855951751640, 0.3900199530189821795, 0.4050207204427892504, 0.4200214878665962659, 0.4350222552904032813, 0.4500230227142102968, 0.4650237901380173122, 0.4800245575618242722, 0.4950253249856313431, 0.5100260924094384141, 0.5250268598332453740, 0.5400276272570523339, 0.5550283946808594049, 0.5700291621046664758, 0.5850299295284734358, 0.6000306969522805067, 0.6150314643760874667, 0.6300322317998945376, 0.6450329992237016086, 0.6600337666475086795, 0.6750345340713155284, 0.6900353014951225994, 0.7050360689189296703, 0.7200368363427366303, 0.7350376037665437012, 0.7500383711903506612, 0.7650391386141577321, 0.7800399060379648031, 0.7950406734617717630, 0.8100414408855787229, 0.8250422083093857939, 0.8400429757331928649, 0.8550437431569998248, 0.8700445105808067847, 0.8850452780046138557, 0.9000460454284209266, 0.9150468128522278866, 0.9300475802760349575, 0.9450483476998419174, 0.9600491151236488774, 0.9717223562348830113 ),
 .UNSPECIFIED. ) 
 CURVE ( )  GEOMETRIC_REPRESENTATION_ITEM ( )  RATIONAL_B_SPLINE_CURVE ( ( 0.9537471549767081447, 0.9702812541832923632, 1.000000000000000000, 0.8660254037844387076, 1.000000000000000000, 0.8660254037844387076, 1.000000000000000000, 0.8660254037844387076, 1.000000000000000000, 0.8660254037844387076, 1.000000000000000000, 0.8660254037844387076, 1.000000000000000000, 0.8660254037844387076, 1.000000000000000000, 0.8660254037844387076, 1.000000000000000000, 0.8660254037844387076, 1.000000000000000000, 0.8660254037844387076, 1.000000000000000000, 0.8660254037844387076, 1.000000000000000000, 0.8660254037844387076, 1.000000000000000000, 0.8660254037844387076, 1.000000000000000000, 0.8660254037844387076, 1.000000000000000000, 0.8660254037844387076, 1.000000000000000000, 0.8660254037844387076, 1.000000000000000000, 0.8660254037844387076, 1.000000000000000000, 0.8660254037844387076, 1.000000000000000000, 0.8660254037844387076, 1.000000000000000000, 0.8660254037844387076, 1.000000000000000000, 0.8660254037844387076, 1.000000000000000000, 0.8660254037844387076, 1.000000000000000000, 0.8660254037844387076, 1.000000000000000000, 0.8660254037844387076, 1.000000000000000000, 0.8660254037844387076, 1.000000000000000000, 0.8660254037844387076, 1.000000000000000000, 0.8660254037844387076, 1.000000000000000000, 0.8660254037844387076, 1.000000000000000000, 0.8660254037844387076, 1.000000000000000000, 0.8660254037844387076, 1.000000000000000000, 0.8660254037844387076, 1.000000000000000000, 0.8660254037844387076, 1.000000000000000000, 0.8660254037844387076, 1.000000000000000000, 0.8660254037844387076, 1.000000000000000000, 0.8660254037844387076, 1.000000000000000000, 0.8660254037844387076, 1.000000000000000000, 0.8660254037844387076, 1.000000000000000000, 0.8660254037844387076, 1.000000000000000000, 0.8660254037844387076, 1.000000000000000000, 0.8660254037844387076, 1.000000000000000000, 0.8957441496011429027, 0.9537471549767118084 ) ) 
 REPRESENTATION_ITEM ( '' )  );
#15511=DIRECTION ( 'NONE',  ( -0.000000000000000000, -1.000000000000000000, -0.000000000000000000 ) ) ;
#15513=CARTESIAN_POINT ( 'NONE',  ( 79.64356964375001269, -31.86562499938548143, -101.5914258081833879 ) ) ;
#15524=ORIENTED_EDGE ( 'NONE', *, *, #9846, .T. ) ;
#15525=CARTESIAN_POINT ( 'NONE',  ( -85.15643035624999868, -31.52812499938547930, -101.5914258081833879 ) ) ;
#15528=CARTESIAN_POINT ( 'NONE',  ( 81.02178482187500208, -34.60312499938549280, 97.61286128772489690 ) ) ;
#15530=CARTESIAN_POINT ( 'NONE',  ( -82.39999999999999147, -33.65624999877096712, -103.4641016151377499 ) ) ;
#15531=CARTESIAN_POINT ( 'NONE',  ( 80.90000000000000568, -32.85000000000000142, 102.5980762113533018 ) ) ;
#15536=CARTESIAN_POINT ( 'NONE',  ( 84.59935209580758908, -34.99999999999999289, -101.7928000422457728 ) ) ;
#15542=CARTESIAN_POINT ( 'NONE',  ( 84.05108659120821812, -32.00820041275123629, -97.77040367152264366 ) ) ;
#15544=CARTESIAN_POINT ( 'NONE',  ( -84.51154815724953551, -35.14114861271051637, -101.7717992799616553 ) ) ;
#15546=ORIENTED_EDGE ( 'NONE', *, *, #14987, .F. ) ;
#15549=PLANE ( 'NONE',  #2869 ) ;
#15550=VERTEX_POINT ( 'NONE', #4456 ) ;
#15552=AXIS2_PLACEMENT_3D ( 'NONE', #6528, #10030, #7001 ) ;
#15555=CARTESIAN_POINT ( 'NONE',  ( 80.90000000000000568, -33.24374999877097281, -97.40192378864668399 ) ) ;
#15556=CARTESIAN_POINT ( 'NONE',  ( 83.77821517812500929, -34.71562499938548285, -97.61286128772489690 ) ) ;
#15557=CYLINDRICAL_SURFACE ( 'NONE', #11103, 3.000000000000002665 ) ;
#15558=CARTESIAN_POINT ( 'NONE',  ( -82.39999999999999147, -30.36562499938549209, 96.81714838363319586 ) ) ;
#15561=DIRECTION ( 'NONE',  ( -0.000000000000000000, 1.000000000000000000, -0.000000000000000000 ) ) ;
#15562=CARTESIAN_POINT ( 'NONE',  ( 85.15643035625001289, -32.54062499938548569, -98.40857419181659793 ) ) ;
#15563=AXIS2_PLACEMENT_3D ( 'NONE', #11499, #10034, #1430 ) ;
#15564=CARTESIAN_POINT ( 'NONE',  ( -80.90000000000000568, -33.84374999877096712, 102.5980762113533018 ) ) ;
#15565=CARTESIAN_POINT ( 'NONE',  ( -83.77821517812500929, -34.26562499938548711, 97.61286128772489690 ) ) ;
#15567=DIRECTION ( 'NONE',  ( 0.000000000000000000, 0.000000000000000000, 1.000000000000000000 ) ) ;
#15570=CARTESIAN_POINT ( 'NONE',  ( -85.40000000000000568, -33.63750000000000284, 98.26794919243111792 ) ) ;
#15575=CARTESIAN_POINT ( 'NONE',  ( -80.90000000000000568, -32.40000000000000568, 97.40192378864668399 ) ) ;
#15577=VERTEX_POINT ( 'NONE', #12070 ) ;
#15580=CARTESIAN_POINT ( 'NONE',  ( 82.85452780460276756, -34.99999999999997868, 97.27546421900271412 ) ) ;
#15581=CARTESIAN_POINT ( 'NONE',  ( 79.64356964375001269, -31.30312499938548854, 98.40857419181659793 ) ) ;
#15583=EDGE_CURVE ( 'NONE', #11146, #5933, #9133, .T. ) ;
#15586=CARTESIAN_POINT ( 'NONE',  ( 83.77821517812500929, -32.31562499938548427, 97.61286128772489690 ) ) ;
#15587=ADVANCED_FACE ( 'NONE', ( #7577 ), #124, .F. ) ;
#15588=CARTESIAN_POINT ( 'NONE',  ( 83.77821517812500929, -32.12812499938548427, -97.61286128772489690 ) ) ;
#15590=CARTESIAN_POINT ( 'NONE',  ( -79.64356964374998427, -34.04062499938549280, 98.40857419181659793 ) ) ;
#15591=CARTESIAN_POINT ( 'NONE',  ( -79.64356964375001269, -31.30312499938548854, -98.40857419181659793 ) ) ;
#15592=ADVANCED_FACE ( 'NONE', ( #11454 ), #6778, .F. ) ;
#15593=ORIENTED_EDGE ( 'NONE', *, *, #3547, .F. ) ;
#15594=CARTESIAN_POINT ( 'NONE',  ( 82.39999999999999147, -33.06562499938548427, 103.1828516163667899 ) ) ;
#15596=CARTESIAN_POINT ( 'NONE',  ( -85.15643035624999868, -31.97812499938548925, 98.40857419181659793 ) ) ;
#15597=CARTESIAN_POINT ( 'NONE',  ( -79.64356964374999848, -34.97812499938548569, 99.99999999999998579 ) ) ;
#15598=CARTESIAN_POINT ( 'NONE',  ( 83.20384757729335945, -34.85759618943233562, 96.99999999999998579 ) ) ;
#15600=CARTESIAN_POINT ( 'NONE',  ( -79.39999999999999147, -33.33749999999999858, -101.7320508075688821 ) ) ;
#15602=FACE_OUTER_BOUND ( 'NONE', #17744, .T. ) ;
#15608=DIRECTION ( 'NONE',  ( 0.000000000000000000, -1.000000000000000000, 0.000000000000000000 ) ) ;
#15609=CARTESIAN_POINT ( 'NONE',  ( -69.99999999999998579, -32.00000000000000000, 150.0000000000000000 ) ) ;
#15611=CARTESIAN_POINT ( 'NONE',  ( 83.77821517812500929, -30.32812499938548711, 102.3871387122750889 ) ) ;
#15613=CARTESIAN_POINT ( 'NONE',  ( 83.77821517812500929, -31.52812499938548996, -102.3871387122750889 ) ) ;
#15616=CARTESIAN_POINT ( 'NONE',  ( 79.39999999999999147, -31.55624999877096926, 98.26794919243113213 ) ) ;
#15621=CARTESIAN_POINT ( 'NONE',  ( 85.40000000000000568, -34.01250000000000284, 98.26794919243111792 ) ) ;
#15624=CARTESIAN_POINT ( 'NONE',  ( -83.77821517812500929, -30.51562499938548711, -97.61286128772489690 ) ) ;
#15625=PLANE ( 'NONE',  #7552 ) ;
#15626=ORIENTED_EDGE ( 'NONE', *, *, #15093, .F. ) ;
#15627=CARTESIAN_POINT ( 'NONE',  ( 79.64356964374998427, -33.59062499938548285, 101.5914258081833879 ) ) ;
#15628=CARTESIAN_POINT ( 'NONE',  ( -85.40000000000000568, -33.09374999877096712, -99.99999999999998579 ) ) ;
#15630=CARTESIAN_POINT ( 'NONE',  ( 80.90000000000000568, -33.45000000000000284, 97.40192378864668399 ) ) ;
#15636=CARTESIAN_POINT ( 'NONE',  ( -82.40000000000000568, -34.10624999877096997, 96.99999999999998579 ) ) ;
#15639=CARTESIAN_POINT ( 'NONE',  ( 82.39999999999999147, -33.17812499938548854, -103.1828516163667899 ) ) ;
#15641=CARTESIAN_POINT ( 'NONE',  ( -79.64356964374999848, -34.86562499938548143, -99.99999999999998579 ) ) ;
#15647=VERTEX_POINT ( 'NONE', #5606 ) ;
#15651=DIRECTION ( 'NONE',  ( 1.000000000000000000, 0.000000000000000000, 0.000000000000000000 ) ) ;
#15652=CARTESIAN_POINT ( 'NONE',  ( 83.90000000000000568, -33.67500000000000426, -97.40192378864668399 ) ) ;
#15653=CYLINDRICAL_SURFACE ( 'NONE', #16107, 3.000000000000002665 ) ;
#15654=CARTESIAN_POINT ( 'NONE',  ( -83.90000000000000568, -34.06874999877096855, 97.40192378864668399 ) ) ;
#15658=CARTESIAN_POINT ( 'NONE',  ( 81.02178482187500208, -34.60312499938549280, -102.3871387122750889 ) ) ;
#15660=CARTESIAN_POINT ( 'NONE',  ( -79.64356964375001269, -33.10312499938549280, 101.5914258081833879 ) ) ;
#15662=ORIENTED_EDGE ( 'NONE', *, *, #5299, .T. ) ;
#15664=CARTESIAN_POINT ( 'NONE',  ( -79.39999999999999147, -33.41250000000000142, 101.7320508075688537 ) ) ;
#15667=CARTESIAN_POINT ( 'NONE',  ( 85.40000000000000568, -33.63750000000000284, 101.7320508075688821 ) ) ;
#15672=CARTESIAN_POINT ( 'NONE',  ( -81.96801452314034009, -35.00000000000001421, -97.27181766474433289 ) ) ;
#15674=CARTESIAN_POINT ( 'NONE',  ( 82.39999999999999147, -33.40312499938548285, 103.1828516163667899 ) ) ;
#15676=EDGE_CURVE ( 'NONE', #9425, #12925, #6875, .T. ) ;
#15677=VECTOR ( 'NONE', #4187, 1000.000000000000000 ) ;
#15679=DIRECTION ( 'NONE',  ( 0.000000000000000000, -1.000000000000000000, 0.000000000000000000 ) ) ;
#15681=CARTESIAN_POINT ( 'NONE',  ( -83.77821517812500929, -32.12812499938548427, -102.3871387122750889 ) ) ;
#15682=CARTESIAN_POINT ( 'NONE',  ( 85.15643035625001289, -31.04062499938548569, 99.99999999999998579 ) ) ;
#15684=ADVANCED_FACE ( 'NONE', ( #8236 ), #1010, .T. ) ;
#15685=CARTESIAN_POINT ( 'NONE',  ( 82.39999999999999147, -34.19062499938548427, -103.1828516163667899 ) ) ;
#15687=CARTESIAN_POINT ( 'NONE',  ( -85.15643035625001289, -33.40312499938548285, 99.99999999999998579 ) ) ;
#15689=CARTESIAN_POINT ( 'NONE',  ( 85.15643035624999868, -32.99062499938548854, 101.5914258081833879 ) ) ;
#15692=VECTOR ( 'NONE', #1163, 1000.000000000000000 ) ;
#15693=CARTESIAN_POINT ( 'NONE',  ( -82.39999999999999147, -34.19062499938548427, 103.1828516163667899 ) ) ;
#15696=CARTESIAN_POINT ( 'NONE',  ( -83.90000000000000568, -34.12500000000000000, -102.5980762113533018 ) ) ;
#15701=EDGE_CURVE ( 'NONE', #17884, #422, #4032, .T. ) ;
#15702=ADVANCED_FACE ( 'NONE', ( #15948 ), #18886, .T. ) ;
#15704=CARTESIAN_POINT ( 'NONE',  ( 82.40000000000000568, -34.10624999877096997, -96.99999999999998579 ) ) ;
#15705=CARTESIAN_POINT ( 'NONE',  ( -82.39999999999999147, -33.43124999877097281, -96.99999999999998579 ) ) ;
#15706=FACE_OUTER_BOUND ( 'NONE', #15400, .T. ) ;
#15707=AXIS2_PLACEMENT_3D ( 'NONE', #428, #1872, #18198 ) ;
#15710=CARTESIAN_POINT ( 'NONE',  ( 85.15643035625001289, -32.05312499938548854, -99.99999999999998579 ) ) ;
#15712=EDGE_LOOP ( 'NONE', ( #8634, #8851, #16541, #18126 ) ) ;
#15718=VERTEX_POINT ( 'NONE', #18597 ) ;
#15719=CARTESIAN_POINT ( 'NONE',  ( -81.02178482187500208, -32.54062499938548569, -102.3871387122750889 ) ) ;
#15721=ORIENTED_EDGE ( 'NONE', *, *, #6998, .T. ) ;
#15722=CARTESIAN_POINT ( 'NONE',  ( 85.15643035625001289, -33.44062499938548427, 101.5914258081833879 ) ) ;
#15723=CARTESIAN_POINT ( 'NONE',  ( -82.39999999999999147, -33.20624999877097139, -103.4641016151377499 ) ) ;
#15724=CARTESIAN_POINT ( 'NONE',  ( 80.90000000000000568, -34.35000000000000853, 97.40192378864668399 ) ) ;
#15725=CARTESIAN_POINT ( 'NONE',  ( -99.99999999999998579, 0.000000000000000000, 150.0000000000000000 ) ) ;
#15729=CARTESIAN_POINT ( 'NONE',  ( -85.15643035625001289, -32.84062499938548285, -99.99999999999998579 ) ) ;
#15730=CARTESIAN_POINT ( 'NONE',  ( 69.99999999999998579, -31.99999999999998579, 150.0000000000000000 ) ) ;
#15738=LINE ( 'NONE', #1078, #2428 ) ;
#15740=CARTESIAN_POINT ( 'NONE',  ( 83.90000000000000568, -32.62500000000000000, 97.40192378864668399 ) ) ;
#15743=VERTEX_POINT ( 'NONE', #5413 ) ;
#15748=CARTESIAN_POINT ( 'NONE',  ( 80.90000000000000568, -32.10000000000000142, -102.5980762113533018 ) ) ;
#15750=CARTESIAN_POINT ( 'NONE',  ( -79.64356964375001269, -30.44062499938548783, 98.40857419181659793 ) ) ;
#15752=CARTESIAN_POINT ( 'NONE',  ( -85.40000000000000568, -32.19374999877096855, -99.99999999999998579 ) ) ;
#15754=CARTESIAN_POINT ( 'NONE',  ( 82.39999999999999147, -34.41562499938548569, -96.81714838363319586 ) ) ;
#15756=CARTESIAN_POINT ( 'NONE',  ( -81.02178482187500208, -32.69062499938548427, 102.3871387122750889 ) ) ;
#15758=VERTEX_POINT ( 'NONE', #15858 ) ;
#15762=CARTESIAN_POINT ( 'NONE',  ( 83.20384757729337366, -34.80134618820331127, 97.00000000000000000 ) ) ;
#15770=CARTESIAN_POINT ( 'NONE',  ( 85.15643035625001289, -32.84062499938548285, 99.99999999999998579 ) ) ;
#15775=CARTESIAN_POINT ( 'NONE',  ( -81.02178482187500208, -33.10312499938548569, -102.3871387122750889 ) ) ;
#15776=CARTESIAN_POINT ( 'NONE',  ( 81.02178482187500208, -32.54062499938548569, 102.3871387122750889 ) ) ;
#15777=CARTESIAN_POINT ( 'NONE',  ( 81.02178482187500208, -33.70312499938548711, -102.3871387122750889 ) ) ;
#15779=CARTESIAN_POINT ( 'NONE',  ( -79.64356964374999848, -33.06562499938548427, 99.99999999999998579 ) ) ;
#15780=CARTESIAN_POINT ( 'NONE',  ( 79.64356964374999848, -31.26562499938548356, -99.99999999999998579 ) ) ;
#15782=CARTESIAN_POINT ( 'NONE',  ( 79.64356964374999848, -34.97812499938548569, 99.99999999999998579 ) ) ;
#15786=VECTOR ( 'NONE', #452, 1000.000000000000000 ) ;
#15787=CARTESIAN_POINT ( 'NONE',  ( 99.99999999999994316, -29.80000000000000782, -150.0000000000000000 ) ) ;
#15788=CARTESIAN_POINT ( 'NONE',  ( -81.02178482187500208, -30.29062499938548569, 97.61286128772489690 ) ) ;
#15791=CARTESIAN_POINT ( 'NONE',  ( -82.39999999999999147, -34.16250000000000142, -103.4641016151377499 ) ) ;
#15793=CARTESIAN_POINT ( 'NONE',  ( 82.39999999999999147, -32.81250000000000000, -97.00000000000000000 ) ) ;
#15798=CARTESIAN_POINT ( 'NONE',  ( 82.40000000000001990, -33.88124999877096855, -103.0000000000000000 ) ) ;
#15799=LINE ( 'NONE', #12662, #16639 ) ;
#15800=CARTESIAN_POINT ( 'NONE',  ( -80.90000000000000568, -32.34374999877096712, -102.5980762113533018 ) ) ;
#15801=CARTESIAN_POINT ( 'NONE',  ( 79.64356964374999848, -31.37812499938548427, 99.99999999999998579 ) ) ;
#15805=CARTESIAN_POINT ( 'NONE',  ( 79.64356964375001269, -34.56562499938549138, -101.5914258081833879 ) ) ;
#15806=DIRECTION ( 'NONE',  ( -0.000000000000000000, -1.000000000000000000, -0.000000000000000000 ) ) ;
#15807=EDGE_CURVE ( 'NONE', #16790, #893, #14584, .T. ) ;
#15808=EDGE_LOOP ( 'NONE', ( #15477, #9307, #7448, #15224 ) ) ;
#15812=CARTESIAN_POINT ( 'NONE',  ( -81.02178482187500208, -30.40312499938548640, 97.61286128772489690 ) ) ;
#15815=CARTESIAN_POINT ( 'NONE',  ( -79.64356964374999848, -31.26562499938548356, -99.99999999999998579 ) ) ;
#15817=EDGE_CURVE ( 'NONE', #10474, #13089, #16710, .T. ) ;
#15819=CARTESIAN_POINT ( 'NONE',  ( 79.64356964374999848, -33.62812499938548427, 99.99999999999998579 ) ) ;
#15820=CARTESIAN_POINT ( 'NONE',  ( -79.64356964374999848, -31.82812499938548356, -99.99999999999998579 ) ) ;
#15825=CARTESIAN_POINT ( 'NONE',  ( -85.15643035625001289, -32.42812499938548854, -101.5914258081833879 ) ) ;
#15826=CARTESIAN_POINT ( 'NONE',  ( -79.39999999999999147, -34.21874999877096712, -99.99999999999998579 ) ) ;
#15828=AXIS2_PLACEMENT_3D ( 'NONE', #5157, #15511, #14132 ) ;
#15831=ORIENTED_EDGE ( 'NONE', *, *, #15355, .T. ) ;
#15832=CARTESIAN_POINT ( 'NONE',  ( 81.02178482187500208, -33.89062499938548711, -97.61286128772489690 ) ) ;
#15840=ORIENTED_EDGE ( 'NONE', *, *, #10457, .T. ) ;
#15843=EDGE_LOOP ( 'NONE', ( #2345, #12878, #2201, #5726 ) ) ;
#15845=CARTESIAN_POINT ( 'NONE',  ( 79.39999999999999147, -33.37500000000000000, -99.99999999999998579 ) ) ;
#15849=CARTESIAN_POINT ( 'NONE',  ( -85.15643035624999868, -31.64062499938548356, 98.40857419181659793 ) ) ;
#15856=CARTESIAN_POINT ( 'NONE',  ( 79.39999999999999147, -33.86250000000000426, 98.26794919243113213 ) ) ;
#15858=CARTESIAN_POINT ( 'NONE',  ( 82.40000000000000568, -34.10624999877096997, -96.99999999999998579 ) ) ;
#15871=CARTESIAN_POINT ( 'NONE',  ( 79.39999999999999147, -30.71250000000000568, 98.26794919243113213 ) ) ;
#15876=CARTESIAN_POINT ( 'NONE',  ( -82.39999999999999147, -33.29062499938548569, -96.81714838363319586 ) ) ;
#15877=CARTESIAN_POINT ( 'NONE',  ( 85.15643035624999868, -31.45312499938548356, 98.40857419181659793 ) ) ;
#15878=CARTESIAN_POINT ( 'NONE',  ( 79.64356964374999848, -34.07812499938548711, -99.99999999999998579 ) ) ;
#15880=CARTESIAN_POINT ( 'NONE',  ( -83.77821517812500929, -32.46562499938548285, 97.61286128772489690 ) ) ;
#15881=CARTESIAN_POINT ( 'NONE',  ( 83.77821517812500929, -31.56562499938548427, -97.61286128772489690 ) ) ;
#15883=CARTESIAN_POINT ( 'NONE',  ( 83.77821517812500929, -34.22812499938549280, 97.61286128772489690 ) ) ;
#15886=CARTESIAN_POINT ( 'NONE',  ( -81.02178482187500208, -32.54062499938548569, 97.61286128772489690 ) ) ;
#15887=CARTESIAN_POINT ( 'NONE',  ( -81.02178482187500208, -30.89062499938548711, 102.3871387122750889 ) ) ;
#15888=CARTESIAN_POINT ( 'NONE',  ( -82.40000000000000568, -30.00000000000000355, 96.99999999999998579 ) ) ;
#15892=CARTESIAN_POINT ( 'NONE',  ( -79.39999999999999147, -32.90624999877096712, 101.7320508075688537 ) ) ;
#15898=CARTESIAN_POINT ( 'NONE',  ( 79.64356964374999848, -34.97812499938548569, -99.99999999999998579 ) ) ;
#15901=( BOUNDED_CURVE ( )  B_SPLINE_CURVE ( 2, ( #1572, #1664, #6065, #12011, #6448, #4594, #10932, #10552, #12399 ),
 .UNSPECIFIED., .F., .F. ) 
 B_SPLINE_CURVE_WITH_KNOTS ( ( 3, 2, 2, 2, 3 ),
 ( 0.6458333333333332593, 0.6527777777777777901, 0.6666666666666666297, 0.6805555555555555802, 0.6875000000000000000 ),
 .UNSPECIFIED. ) 
 CURVE ( )  GEOMETRIC_REPRESENTATION_ITEM ( )  RATIONAL_B_SPLINE_CURVE ( ( 0.9330127018922192983, 0.9330127018922187432, 1.000000000000000000, 0.8660254037844387076, 1.000000000000000000, 0.8660254037844387076, 1.000000000000000000, 0.9330127018922194093, 0.9330127018922194093 ) ) 
 REPRESENTATION_ITEM ( '' )  );
#15902=CARTESIAN_POINT ( 'NONE',  ( 79.39999999999999147, -32.45624999877097139, 98.26794919243113213 ) ) ;
#15906=CARTESIAN_POINT ( 'NONE',  ( -79.77811200999887831, -35.00000000000000000, 100.8506536761481414 ) ) ;
#15909=CARTESIAN_POINT ( 'NONE',  ( -83.77821517812500929, -32.91562499938547859, -102.3871387122750889 ) ) ;
#15910=CARTESIAN_POINT ( 'NONE',  ( -94.79999999999999716, -3.000000000000000000, -150.0000000000000000 ) ) ;
#15911=ORIENTED_EDGE ( 'NONE', *, *, #3153, .T. ) ;
#15912=CARTESIAN_POINT ( 'NONE',  ( 83.77821517812500929, -34.22812499938549280, 97.61286128772489690 ) ) ;
#15913=CARTESIAN_POINT ( 'NONE',  ( -85.15643035625001289, -31.15312499938548996, -99.99999999999998579 ) ) ;
#15914=CARTESIAN_POINT ( 'NONE',  ( 85.40000000000000568, -33.56250000000000000, 98.26794919243111792 ) ) ;
#15915=CARTESIAN_POINT ( 'NONE',  ( -79.59365286754820090, -34.99999999999999289, 99.92898555286045337 ) ) ;
#15918=CARTESIAN_POINT ( 'NONE',  ( -82.39999999999999147, -33.85312499938548569, -103.1828516163667899 ) ) ;
#15919=EDGE_CURVE ( 'NONE', #518, #4595, #11463, .T. ) ;
#15922=CARTESIAN_POINT ( 'NONE',  ( 85.40000000000000568, -31.33124999877096428, -98.26794919243111792 ) ) ;
#15925=ORIENTED_EDGE ( 'NONE', *, *, #10908, .T. ) ;
#15930=EDGE_LOOP ( 'NONE', ( #16900, #12609, #12995, #2780 ) ) ;
#15931=VERTEX_POINT ( 'NONE', #9255 ) ;
#15936=DIRECTION ( 'NONE',  ( -0.000000000000000000, -0.000000000000000000, -1.000000000000000000 ) ) ;
#15937=CARTESIAN_POINT ( 'NONE',  ( 80.90000000000000568, -32.85000000000000142, -97.40192378864668399 ) ) ;
#15938=CARTESIAN_POINT ( 'NONE',  ( 82.86160995759659897, -32.00000000000000000, -102.8104067583495578 ) ) ;
#15940=CARTESIAN_POINT ( 'NONE',  ( -79.64356964374999848, -31.82812499938548356, 99.99999999999998579 ) ) ;
#15947=CARTESIAN_POINT ( 'NONE',  ( -85.15643035624999868, -35.05312499938548143, 101.5914258081833879 ) ) ;
#15948=FACE_OUTER_BOUND ( 'NONE', #10074, .T. ) ;
#15951=CARTESIAN_POINT ( 'NONE',  ( -84.51154815724953551, -35.25364861271051353, -101.7717992799616553 ) ) ;
#15952=DIRECTION ( 'NONE',  ( -0.000000000000000000, -1.000000000000000000, -0.000000000000000000 ) ) ;
#15953=CARTESIAN_POINT ( 'NONE',  ( -82.39999999999999147, -34.83749999999999858, -97.00000000000000000 ) ) ;
#15958=CARTESIAN_POINT ( 'NONE',  ( -82.39999999999999147, -30.50624999877097210, 96.53589838486223584 ) ) ;
#15959=CARTESIAN_POINT ( 'NONE',  ( 85.15643035625001289, -35.09062499938548285, 99.99999999999998579 ) ) ;
#15960=LINE ( 'NONE', #2566, #1201 ) ;
#15963=EDGE_CURVE ( 'NONE', #18433, #2579, #8184, .T. ) ;
#15965=CARTESIAN_POINT ( 'NONE',  ( -83.77821517812500929, -33.47812499938548569, -102.3871387122750889 ) ) ;
#15966=CARTESIAN_POINT ( 'NONE',  ( 83.90000000000000568, -33.16874999877096286, -97.40192378864668399 ) ) ;
#15968=B_SPLINE_CURVE_WITH_KNOTS ( 'NONE', 3,
 ( #17016, #5108, #15455, #12232, #5014, #10954, #9389, #15354, #16831, #3438, #18201, #13592, #9196, #15260, #232, #4914, #6285, #621 ),
 .UNSPECIFIED., .F., .F.,
 ( 4, 2, 2, 2, 2, 2, 2, 2, 4 ),
 ( 0.000000000000000000, 0.0007106627595359156415, 0.001421325519071831283, 0.002131988278607746708, 0.002842651038143662566, 0.003553313797679578424, 0.004263976557215493415, 0.004974639316751409274, 0.005685302076287325132 ),
 .UNSPECIFIED. ) ;
#15969=CARTESIAN_POINT ( 'NONE',  ( 82.39999999999999147, -35.09062499938548285, -103.1828516163667899 ) ) ;
#15971=CARTESIAN_POINT ( 'NONE',  ( -85.15643035625001289, -33.70312499938548711, 101.5914258081833879 ) ) ;
#15972=CARTESIAN_POINT ( 'NONE',  ( 83.77821517812500929, -30.96562499938548640, -102.3871387122750889 ) ) ;
#15973=EDGE_LOOP ( 'NONE', ( #6326, #6467, #10575, #7183 ) ) ;
#15974=CARTESIAN_POINT ( 'NONE',  ( 83.77821517812500929, -35.12812499938548427, 97.61286128772489690 ) ) ;
#15979=CARTESIAN_POINT ( 'NONE',  ( -85.15643035624999868, -34.15312499938548285, 101.5914258081833879 ) ) ;
#15980=CARTESIAN_POINT ( 'NONE',  ( -85.15643035625001289, -31.04062499938548569, 99.99999999999998579 ) ) ;
#15986=CYLINDRICAL_SURFACE ( 'NONE', #9216, 3.000000000000002665 ) ;
#15987=CARTESIAN_POINT ( 'NONE',  ( -84.42750213138106119, -35.00000000000000711, 97.77995849557629526 ) ) ;
#15988=DIRECTION ( 'NONE',  ( 0.000000000000000000, -1.000000000000000000, 0.000000000000000000 ) ) ;
#15989=CARTESIAN_POINT ( 'NONE',  ( 84.44763168836732348, -32.00000000000002132, 98.15470523285560489 ) ) ;
#15990=DIRECTION ( 'NONE',  ( -1.000000000000000000, 0.000000000000000000, 0.000000000000000000 ) ) ;
#15992=CARTESIAN_POINT ( 'NONE',  ( -82.39999999999999147, -32.58749999999999858, -96.99999999999998579 ) ) ;
#15993=CARTESIAN_POINT ( 'NONE',  ( 81.02178482187500208, -34.15312499938548285, -102.3871387122750889 ) ) ;
#15996=VECTOR ( 'NONE', #6990, 1000.000000000000000 ) ;
#15998=CARTESIAN_POINT ( 'NONE',  ( 79.39999999999999147, -32.00624999877096855, 98.26794919243113213 ) ) ;
#16002=CARTESIAN_POINT ( 'NONE',  ( 85.40000000000000568, -34.08749999999999858, 101.7320508075688821 ) ) ;
#16004=CARTESIAN_POINT ( 'NONE',  ( -79.64356964375001269, -34.00312499938549138, -98.40857419181659793 ) ) ;
#16006=VERTEX_POINT ( 'NONE', #15314 ) ;
#16007=CARTESIAN_POINT ( 'NONE',  ( -83.20384757729337366, -34.80134618820331127, -97.00000000000000000 ) ) ;
#16008=CARTESIAN_POINT ( 'NONE',  ( -85.15643035624999868, -32.09062499938548996, -101.5914258081833879 ) ) ;
#16010=CARTESIAN_POINT ( 'NONE',  ( 80.90000000000000568, -34.80000000000000426, 97.40192378864668399 ) ) ;
#16015=CARTESIAN_POINT ( 'NONE',  ( -82.39999999999999147, -33.40312499938548285, -103.1828516163667899 ) ) ;
#16018=CARTESIAN_POINT ( 'NONE',  ( 79.39999999999999147, -31.48124999877097352, -98.26794919243110371 ) ) ;
#16024=DIRECTION ( 'NONE',  ( -1.000000000000000000, 0.000000000000000000, 0.000000000000000000 ) ) ;
#16029=CARTESIAN_POINT ( 'NONE',  ( -79.58826230849687988, -32.00000000000094502, 98.95399275615287138 ) ) ;
#16032=CARTESIAN_POINT ( 'NONE',  ( 85.40000000000000568, -32.70000000000000284, -99.99999999999998579 ) ) ;
#16034=ADVANCED_FACE ( 'NONE', ( #17074 ), #388, .F. ) ;
#16036=CARTESIAN_POINT ( 'NONE',  ( -85.15643035625001289, -31.60312499938548569, 99.99999999999998579 ) ) ;
#16039=CARTESIAN_POINT ( 'NONE',  ( 79.64356964374999848, -34.52812499938548285, -99.99999999999998579 ) ) ;
#16041=FACE_OUTER_BOUND ( 'NONE', #1245, .T. ) ;
#16042=CARTESIAN_POINT ( 'NONE',  ( -83.20384757729335945, -34.40759618943233988, -96.99999999999998579 ) ) ;
#16044=CARTESIAN_POINT ( 'NONE',  ( -79.64356964374999848, -31.26562499938548356, -99.99999999999998579 ) ) ;
#16045=DIRECTION ( 'NONE',  ( -0.000000000000000000, -1.000000000000000000, -0.000000000000000000 ) ) ;
#16047=( BOUNDED_CURVE ( )  B_SPLINE_CURVE ( 2, ( #14999, #10693, #1620, #16660, #13236, #7572, #6216, #10603, #1335 ),
 .UNSPECIFIED., .F., .F. ) 
 B_SPLINE_CURVE_WITH_KNOTS ( ( 3, 2, 2, 2, 3 ),
 ( 0.5625000000000000000, 0.5694444444444444198, 0.5833333333333333703, 0.5972222222222222099, 0.6041666666666666297 ),
 .UNSPECIFIED. ) 
 CURVE ( )  GEOMETRIC_REPRESENTATION_ITEM ( )  RATIONAL_B_SPLINE_CURVE ( ( 0.9330127018922194093, 0.9330127018922194093, 1.000000000000000000, 0.8660254037844387076, 1.000000000000000000, 0.8660254037844387076, 1.000000000000000000, 0.9330127018922198534, 0.9330127018922192983 ) ) 
 REPRESENTATION_ITEM ( '' )  );
#16048=CARTESIAN_POINT ( 'NONE',  ( 83.90000000000000568, -34.96874999877096712, 102.5980762113533018 ) ) ;
#16051=CARTESIAN_POINT ( 'NONE',  ( 80.90000000000000568, -32.55000000000000426, 97.40192378864668399 ) ) ;
#16057=CARTESIAN_POINT ( 'NONE',  ( 81.02178482187500208, -33.89062499938548711, 102.3871387122750889 ) ) ;
#16060=LINE ( 'NONE', #11566, #7041 ) ;
#16062=CARTESIAN_POINT ( 'NONE',  ( -82.39999999999999147, -33.51562499938548711, -103.1828516163667899 ) ) ;
#16064=CARTESIAN_POINT ( 'NONE',  ( 81.02178482187500208, -33.55312499938548854, -97.61286128772489690 ) ) ;
#16066=CARTESIAN_POINT ( 'NONE',  ( -82.39999999999999147, -32.72812499938548569, 103.1828516163667899 ) ) ;
#16067=CARTESIAN_POINT ( 'NONE',  ( 85.15643035624999868, -30.62812499938548427, -98.40857419181659793 ) ) ;
#16072=CARTESIAN_POINT ( 'NONE',  ( -85.15643035624999868, -33.25312499938548427, 101.5914258081833879 ) ) ;
#16073=CARTESIAN_POINT ( 'NONE',  ( -81.02178482187500208, -31.79062499938548925, 102.3871387122750889 ) ) ;
#16078=CARTESIAN_POINT ( 'NONE',  ( 82.17437583783166133, -34.99999999999999289, -97.01974242045223207 ) ) ;
#16079=DIRECTION ( 'NONE',  ( 0.000000000000000000, 0.000000000000000000, -1.000000000000000000 ) ) ;
#16081=CARTESIAN_POINT ( 'NONE',  ( -85.40000000000000568, -34.46249999999999858, 101.7320508075688821 ) ) ;
#16083=EDGE_CURVE ( 'NONE', #7832, #17884, #10095, .T. ) ;
#16084=CARTESIAN_POINT ( 'NONE',  ( -79.39999999999999147, -32.83124999877097139, 98.26794919243110371 ) ) ;
#16086=CARTESIAN_POINT ( 'NONE',  ( -82.40000000000000568, -32.30624999877097281, -102.9999999999999858 ) ) ;
#16087=CARTESIAN_POINT ( 'NONE',  ( 81.02178482187500208, -33.55312499938548854, 102.3871387122750889 ) ) ;
#16089=CARTESIAN_POINT ( 'NONE',  ( -83.20384757729337366, -32.79240381056766296, -103.0000000000000000 ) ) ;
#16090=CARTESIAN_POINT ( 'NONE',  ( 79.64356964375001269, -32.69062499938548427, -98.40857419181659793 ) ) ;
#16094=CARTESIAN_POINT ( 'NONE',  ( 85.40000000000000568, -33.50624999877096855, 98.26794919243111792 ) ) ;
#16101=CARTESIAN_POINT ( 'NONE',  ( -79.64356964375001269, -34.82812499938548711, -101.5914258081833879 ) ) ;
#16102=CARTESIAN_POINT ( 'NONE',  ( 79.39999999999999147, -32.45624999877097139, 98.26794919243113213 ) ) ;
#16104=EDGE_CURVE ( 'NONE', #5607, #17007, #9984, .T. ) ;
#16106=CARTESIAN_POINT ( 'NONE',  ( -81.02178482187500208, -30.85312499938548569, -102.3871387122750889 ) ) ;
#16107=AXIS2_PLACEMENT_3D ( 'NONE', #9490, #12715, #18689 ) ;
#16108=CARTESIAN_POINT ( 'NONE',  ( -80.90000000000000568, -32.49374999877097281, -97.40192378864668399 ) ) ;
#16109=CARTESIAN_POINT ( 'NONE',  ( -81.05805657947830412, -35.00000000000002842, 97.38506107425214964 ) ) ;
#16112=CARTESIAN_POINT ( 'NONE',  ( -79.64356964374998427, -32.65312499938548285, -98.40857419181659793 ) ) ;
#16113=FACE_OUTER_BOUND ( 'NONE', #12329, .T. ) ;
#16114=CARTESIAN_POINT ( 'NONE',  ( 79.58826230851033756, -31.99999999999998579, 101.0460072438832952 ) ) ;
#16115=CARTESIAN_POINT ( 'NONE',  ( 82.39999999999999147, -32.30624999877097281, -96.53589838486223584 ) ) ;
#16118=VERTEX_POINT ( 'NONE', #9746 ) ;
#16119=CARTESIAN_POINT ( 'NONE',  ( 81.02178482187500208, -34.49062499938548854, -102.3871387122750889 ) ) ;
#16131=CARTESIAN_POINT ( 'NONE',  ( 80.90000000000000568, -34.35000000000000853, -102.5980762113533018 ) ) ;
#16132=CARTESIAN_POINT ( 'NONE',  ( 80.42036527867307427, -31.99999999999999289, -102.1983759483902645 ) ) ;
#16133=CARTESIAN_POINT ( 'NONE',  ( -79.64356964375001269, -30.51562499938548711, 101.5914258081833879 ) ) ;
#16136=AXIS2_PLACEMENT_3D ( 'NONE', #17487, #2722, #8484 ) ;
#16139=CARTESIAN_POINT ( 'NONE',  ( -79.64356964374999848, -34.86562499938548143, 99.99999999999998579 ) ) ;
#16141=CARTESIAN_POINT ( 'NONE',  ( -83.20384757729338787, -34.53615380933862866, -102.9999999999999858 ) ) ;
#16143=CARTESIAN_POINT ( 'NONE',  ( -82.39999999999999147, -30.25312499938548783, -103.1828516163667899 ) ) ;
#16152=FACE_BOUND ( 'NONE', #18107, .T. ) ;
#16154=CARTESIAN_POINT ( 'NONE',  ( -82.65333140691201663, -34.99995246259153703, -102.9892844631211943 ) ) ;
#16155=CARTESIAN_POINT ( 'NONE',  ( 81.02178482187500208, -34.79062499938548569, 102.3871387122750889 ) ) ;
#16156=AXIS2_PLACEMENT_3D ( 'NONE', #6371, #5008, #16721 ) ;
#16157=CARTESIAN_POINT ( 'NONE',  ( 83.90000000000000568, -33.97500000000000853, -102.5980762113533018 ) ) ;
#16158=EDGE_CURVE ( 'NONE', #10474, #16790, #5647, .T. ) ;
#16164=AXIS2_PLACEMENT_3D ( 'NONE', #5547, #8456, #12766 ) ;
#16165=CARTESIAN_POINT ( 'NONE',  ( 83.77821517812500929, -30.96562499938548640, -102.3871387122750889 ) ) ;
#16167=CARTESIAN_POINT ( 'NONE',  ( -79.64356964374999848, -34.41562499938548569, 99.99999999999998579 ) ) ;
#16168=CARTESIAN_POINT ( 'NONE',  ( 79.64356964375001269, -31.67812499938548143, -98.40857419181659793 ) ) ;
#16175=CARTESIAN_POINT ( 'NONE',  ( -81.02178482187500208, -32.24062499938548854, 102.3871387122750889 ) ) ;
#16176=ORIENTED_EDGE ( 'NONE', *, *, #6023, .F. ) ;
#16177=CARTESIAN_POINT ( 'NONE',  ( -79.39999999999999147, -32.88750000000000284, 98.26794919243110371 ) ) ;
#16178=AXIS2_PLACEMENT_3D ( 'NONE', #12384, #18351, #15311 ) ;
#16181=CARTESIAN_POINT ( 'NONE',  ( 69.99999999999998579, -34.99999999999999289, 150.0000000000000000 ) ) ;
#16186=CARTESIAN_POINT ( 'NONE',  ( -85.40000000000000568, -32.28750000000000142, 98.26794919243111792 ) ) ;
#16189=CARTESIAN_POINT ( 'NONE',  ( 85.15643035624999868, -32.91562499938549280, 98.40857419181659793 ) ) ;
#16193=CARTESIAN_POINT ( 'NONE',  ( 81.02178482187500208, -33.25312499938548427, -102.3871387122750889 ) ) ;
#16194=VECTOR ( 'NONE', #3877, 1000.000000000000000 ) ;
#16195=CARTESIAN_POINT ( 'NONE',  ( -79.64356964374999848, -31.37812499938548427, -99.99999999999998579 ) ) ;
#16196=EDGE_LOOP ( 'NONE', ( #17031, #9784, #3273, #9549 ) ) ;
#16197=CARTESIAN_POINT ( 'NONE',  ( 85.40000000000000568, -32.60624999877097707, 98.26794919243111792 ) ) ;
#16198=LINE ( 'NONE', #273, #6170 ) ;
#16200=FACE_OUTER_BOUND ( 'NONE', #13977, .T. ) ;
#16201=CARTESIAN_POINT ( 'NONE',  ( 82.85293433259542439, -31.99999999999999289, 102.8010948079569005 ) ) ;
#16204=CARTESIAN_POINT ( 'NONE',  ( -79.64356964374999848, -33.96562499938548285, -99.99999999999998579 ) ) ;
#16206=ORIENTED_EDGE ( 'NONE', *, *, #10017, .F. ) ;
#16207=CARTESIAN_POINT ( 'NONE',  ( 79.64356964374999848, -34.98839802032724577, 99.56403331587401340 ) ) ;
#16208=CARTESIAN_POINT ( 'NONE',  ( -85.15643035624999868, -34.34062499938548285, -101.5914258081833879 ) ) ;
#16209=CARTESIAN_POINT ( 'NONE',  ( -80.24181665639368077, -31.99999999999999289, -102.0230471653775766 ) ) ;
#16210=CARTESIAN_POINT ( 'NONE',  ( -80.90000000000000568, -32.04374999877096997, -97.40192378864668399 ) ) ;
#16214=CARTESIAN_POINT ( 'NONE',  ( -81.02178482187500208, -34.34062499938548285, -102.3871387122750889 ) ) ;
#16216=CARTESIAN_POINT ( 'NONE',  ( -82.39999999999999147, -34.33124999877097139, -97.00000000000000000 ) ) ;
#16217=ADVANCED_FACE ( 'NONE', ( #4267 ), #13964, .F. ) ;
#16218=CARTESIAN_POINT ( 'NONE',  ( 85.40000000000000568, -30.88124999877097210, -98.26794919243111792 ) ) ;
#16221=FACE_BOUND ( 'NONE', #1122, .T. ) ;
#16228=CARTESIAN_POINT ( 'NONE',  ( -81.59615242270665192, -34.18259618943233136, -103.0000000000000000 ) ) ;
#16231=VERTEX_POINT ( 'NONE', #9775 ) ;
#16233=CARTESIAN_POINT ( 'NONE',  ( 80.90000000000000568, -34.80000000000000426, -102.5980762113533018 ) ) ;
#16234=CARTESIAN_POINT ( 'NONE',  ( 81.68701737470168212, -31.99999999999999289, -102.8119722220549619 ) ) ;
#16235=CARTESIAN_POINT ( 'NONE',  ( -79.64356964374999848, -34.97812499938548569, 99.99999999999998579 ) ) ;
#16237=CARTESIAN_POINT ( 'NONE',  ( -94.79999999999999716, 0.000000000000000000, 150.0000000000000000 ) ) ;
#16239=CARTESIAN_POINT ( 'NONE',  ( 79.59365286754817248, -35.00000000000000711, 100.0710144471396319 ) ) ;
#16240=CARTESIAN_POINT ( 'NONE',  ( 85.10336890117790176, -35.00000000000000000, 99.00607337841680078 ) ) ;
#16241=CARTESIAN_POINT ( 'NONE',  ( -82.40000000000000568, -34.61250000000001137, -102.9999999999999858 ) ) ;
#16243=( LENGTH_UNIT ( ) NAMED_UNIT ( * ) SI_UNIT ( .MILLI., .METRE. ) );
#16244=CARTESIAN_POINT ( 'NONE',  ( -81.02178482187500208, -30.29062499938548569, -102.3871387122750889 ) ) ;
#16247=CARTESIAN_POINT ( 'NONE',  ( 80.90000000000000568, -32.40000000000000568, 102.5980762113533018 ) ) ;
#16251=CARTESIAN_POINT ( 'NONE',  ( -79.39999999999999147, -34.76250000000000284, -98.26794919243113213 ) ) ;
#16253=CARTESIAN_POINT ( 'NONE',  ( -82.39999999999999147, -30.95624999877097139, 96.53589838486223584 ) ) ;
#16254=CARTESIAN_POINT ( 'NONE',  ( 84.51155491706698797, -35.14114833091483803, 101.7717912238936719 ) ) ;
#16259=CARTESIAN_POINT ( 'NONE',  ( 79.64356964375001269, -34.37812499938548427, 101.5914258081833879 ) ) ;
#16260=CARTESIAN_POINT ( 'NONE',  ( 79.64356964374999848, -31.71562499938548285, -99.99999999999998579 ) ) ;
#16262=CARTESIAN_POINT ( 'NONE',  ( 82.39999999999999147, -33.62812499938549138, -103.1828516163667899 ) ) ;
#16266=LINE ( 'NONE', #16558, #8218 ) ;
#16267=CARTESIAN_POINT ( 'NONE',  ( -82.39999999999999147, -32.50312499938548427, 96.81714838363319586 ) ) ;
#16270=EDGE_CURVE ( 'NONE', #6543, #14497, #1171, .T. ) ;
#16277=CARTESIAN_POINT ( 'NONE',  ( -83.20384757729337366, -32.15759618943233278, 103.0000000000000000 ) ) ;
#16280=CARTESIAN_POINT ( 'NONE',  ( 82.39999999999999147, -32.39062499938548001, 96.81714838363319586 ) ) ;
#16281=CYLINDRICAL_SURFACE ( 'NONE', #6487, 3.000000000000002665 ) ;
#16284=CARTESIAN_POINT ( 'NONE',  ( -85.15643035625001289, -31.60312499938548569, -99.99999999999998579 ) ) ;
#16286=CARTESIAN_POINT ( 'NONE',  ( 79.39999999999999147, -34.21874999877096712, 99.99999999999998579 ) ) ;
#16291=CARTESIAN_POINT ( 'NONE',  ( -83.77821517812500929, -30.77812499938548640, 97.61286128772489690 ) ) ;
#16292=CARTESIAN_POINT ( 'NONE',  ( -94.79999999999999716, -3.000000000000000000, 150.0000000000000000 ) ) ;
#16295=CARTESIAN_POINT ( 'NONE',  ( -85.15643035624999868, -33.32812499938548001, -101.5914258081833879 ) ) ;
#16296=CARTESIAN_POINT ( 'NONE',  ( 81.59615242270663771, -32.51115380933863008, 96.99999999999998579 ) ) ;
#16297=ORIENTED_EDGE ( 'NONE', *, *, #17417, .F. ) ;
#16299=CARTESIAN_POINT ( 'NONE',  ( -79.64356964374999848, -32.27812499938548996, -99.99999999999998579 ) ) ;
#16301=CARTESIAN_POINT ( 'NONE',  ( -85.40000000000000568, -32.15624999877096712, -98.26794919243111792 ) ) ;
#16305=CARTESIAN_POINT ( 'NONE',  ( -79.64356964374998427, -34.82812499938548711, -101.5914258081833879 ) ) ;
#16310=CARTESIAN_POINT ( 'NONE',  ( 79.39999999999999147, -32.83124999877097139, -98.26794919243110371 ) ) ;
#16318=ORIENTED_EDGE ( 'NONE', *, *, #323, .T. ) ;
#16319=CARTESIAN_POINT ( 'NONE',  ( -80.90000000000000568, -34.35000000000000853, -97.40192378864668399 ) ) ;
#16324=CARTESIAN_POINT ( 'NONE',  ( -79.90595866893275456, -34.99999999999999289, 101.1871036926522720 ) ) ;
#16326=CARTESIAN_POINT ( 'NONE',  ( -85.15643035624999868, -33.36562499938548854, 101.5914258081833879 ) ) ;
#16332=CARTESIAN_POINT ( 'NONE',  ( -81.70916641599839636, -35.00000000000000000, -102.8868501612597726 ) ) ;
#16335=CARTESIAN_POINT ( 'NONE',  ( -82.39999999999999147, -33.17812499938548854, -96.81714838363319586 ) ) ;
#16343=ORIENTED_EDGE ( 'NONE', *, *, #15676, .F. ) ;
#16344=CARTESIAN_POINT ( 'NONE',  ( 69.99999999999998579, -34.99999999999999289, 150.0000000000000000 ) ) ;
#16346=CARTESIAN_POINT ( 'NONE',  ( -82.39999999999999147, -32.08124999877097139, 103.4641016151377499 ) ) ;
#16347=CARTESIAN_POINT ( 'NONE',  ( 83.90000000000000568, -32.77499999999999858, 102.5980762113533018 ) ) ;
#16351=CARTESIAN_POINT ( 'NONE',  ( 83.77821517812500929, -34.11562499938548854, 97.61286128772489690 ) ) ;
#16352=CARTESIAN_POINT ( 'NONE',  ( 83.77821517812500929, -32.46562499938548285, -97.61286128772489690 ) ) ;
#16354=B_SPLINE_CURVE_WITH_KNOTS ( 'NONE', 3,
 ( #7493, #13448, #5744, #8762, #10238, #16201, #85, #2902, #8857, #15014, #14714, #7295, #19225, #5841, #11794, #14812, #1439, #13003 ),
 .UNSPECIFIED., .F., .F.,
 ( 4, 2, 2, 2, 2, 2, 2, 2, 4 ),
 ( 0.000000000000000000, 0.0007089252359835869531, 0.001417850471967173906, 0.002126775707950760968, 0.002835700943934347813, 0.003544626179917934657, 0.004253551415901521936, 0.004962476651885108780, 0.005671401887868695625 ),
 .UNSPECIFIED. ) ;
#16356=CARTESIAN_POINT ( 'NONE',  ( -83.77821517812500929, -34.56562499938548427, 102.3871387122750889 ) ) ;
#16357=CARTESIAN_POINT ( 'NONE',  ( 79.64356964375001269, -33.02812499938548285, -98.40857419181659793 ) ) ;
#16358=ORIENTED_EDGE ( 'NONE', *, *, #9468, .T. ) ;
#16359=DIRECTION ( 'NONE',  ( 0.000000000000000000, 0.000000000000000000, 1.000000000000000000 ) ) ;
#16362=CARTESIAN_POINT ( 'NONE',  ( -82.39999999999999147, -30.11250000000000426, 96.53589838486223584 ) ) ;
#16363=ORIENTED_EDGE ( 'NONE', *, *, #15963, .F. ) ;
#16365=EDGE_CURVE ( 'NONE', #6865, #5861, #6031, .T. ) ;
#16371=CARTESIAN_POINT ( 'NONE',  ( -80.90000000000000568, -32.49374999877097281, 102.5980762113533018 ) ) ;
#16374=CARTESIAN_POINT ( 'NONE',  ( 85.15643035624999868, -32.46562499938548996, 98.40857419181659793 ) ) ;
#16376=CARTESIAN_POINT ( 'NONE',  ( -81.02178482187500208, -32.35312499938548569, 102.3871387122750889 ) ) ;
#16377=CARTESIAN_POINT ( 'NONE',  ( -79.64356964374999848, -32.27812499938548996, -99.99999999999998579 ) ) ;
#16379=CARTESIAN_POINT ( 'NONE',  ( 79.64356964375001269, -31.34062499938548640, 101.5914258081833879 ) ) ;
#16384=CARTESIAN_POINT ( 'NONE',  ( -79.64356964375001269, -31.41562499938548569, 101.5914258081833879 ) ) ;
#16386=CARTESIAN_POINT ( 'NONE',  ( -83.90000000000000568, -31.42500000000000071, -102.5980762113533018 ) ) ;
#16389=CARTESIAN_POINT ( 'NONE',  ( -82.39999999999999147, -33.74062499938548854, -96.81714838363319586 ) ) ;
#16391=CARTESIAN_POINT ( 'NONE',  ( -84.11496519894568280, -32.00000000000000000, -102.1846009218959210 ) ) ;
#16392=CARTESIAN_POINT ( 'NONE',  ( -80.90000000000000568, -30.69374999877097210, -97.40192378864668399 ) ) ;
#16397=CARTESIAN_POINT ( 'NONE',  ( 83.77821517812500929, -32.76562499938548711, 97.61286128772489690 ) ) ;
#16401=FACE_OUTER_BOUND ( 'NONE', #1381, .T. ) ;
#16402=CARTESIAN_POINT ( 'NONE',  ( 82.39999999999999147, -35.00624999877097565, -96.53589838486223584 ) ) ;
#16404=ORIENTED_EDGE ( 'NONE', *, *, #12618, .T. ) ;
#16410=ORIENTED_EDGE ( 'NONE', *, *, #14974, .F. ) ;
#16416=ORIENTED_EDGE ( 'NONE', *, *, #4504, .T. ) ;
#16418=DIRECTION ( 'NONE',  ( -1.000000000000000000, 0.000000000000000000, 0.000000000000000000 ) ) ;
#16419=CARTESIAN_POINT ( 'NONE',  ( -79.64356964375001269, -34.49062499938548854, 98.40857419181659793 ) ) ;
#16422=DIRECTION ( 'NONE',  ( -0.000000000000000000, 0.000000000000000000, -1.000000000000000000 ) ) ;
#16431=CARTESIAN_POINT ( 'NONE',  ( -79.64356964375001269, -32.65312499938548285, -98.40857419181659793 ) ) ;
#16434=CARTESIAN_POINT ( 'NONE',  ( 81.28488860390724824, -34.99999999999997868, -102.5271494742948164 ) ) ;
#16438=ORIENTED_EDGE ( 'NONE', *, *, #14974, .T. ) ;
#16441=ADVANCED_FACE ( 'NONE', ( #17761 ), #2899, .F. ) ;
#16443=CARTESIAN_POINT ( 'NONE',  ( -83.90000000000000568, -33.01874999877097139, 102.5980762113533018 ) ) ;
#16444=CARTESIAN_POINT ( 'NONE',  ( 79.39999999999999147, -31.98750000000000071, 101.7320508075688821 ) ) ;
#16445=CARTESIAN_POINT ( 'NONE',  ( -79.93183330737464587, -32.00000000000002132, -98.31447495408076520 ) ) ;
#16449=CARTESIAN_POINT ( 'NONE',  ( -82.40000000000000568, -32.08124999877097139, -97.00000000000000000 ) ) ;
#16450=CARTESIAN_POINT ( 'NONE',  ( 85.15643035624999868, -30.62812499938548427, -98.40857419181659793 ) ) ;
#16451=VERTEX_POINT ( 'NONE', #12174 ) ;
#16453=EDGE_CURVE ( 'NONE', #592, #6950, #18716, .T. ) ;
#16454=CARTESIAN_POINT ( 'NONE',  ( 80.90000000000000568, -34.29374999877096997, 97.40192378864668399 ) ) ;
#16455=CARTESIAN_POINT ( 'NONE',  ( 83.77821517812500929, -33.21562499938548285, -102.3871387122750889 ) ) ;
#16458=CYLINDRICAL_SURFACE ( 'NONE', #9763, 3.000000000000002665 ) ;
#16461=CARTESIAN_POINT ( 'NONE',  ( -80.90000000000000568, -31.50000000000000000, 97.40192378864668399 ) ) ;
#16462=VERTEX_POINT ( 'NONE', #4662 ) ;
#16466=CARTESIAN_POINT ( 'NONE',  ( 79.64356964374999848, -30.36562499938548498, 99.99999999999998579 ) ) ;
#16468=VECTOR ( 'NONE', #19239, 1000.000000000000000 ) ;
#16474=CARTESIAN_POINT ( 'NONE',  ( 85.15643035624999868, -33.36562499938548854, 98.40857419181659793 ) ) ;
#16477=DIRECTION ( 'NONE',  ( 0.000000000000000000, -0.000000000000000000, -1.000000000000000000 ) ) ;
#16478=CARTESIAN_POINT ( 'NONE',  ( -85.15643035625001289, -32.05312499938548854, 99.99999999999998579 ) ) ;
#16479=CARTESIAN_POINT ( 'NONE',  ( -79.64356964374999848, -30.47812499938548569, -99.99999999999998579 ) ) ;
#16480=ORIENTED_EDGE ( 'NONE', *, *, #11264, .F. ) ;
#16481=CARTESIAN_POINT ( 'NONE',  ( 85.40000000000000568, -34.89374999877097139, 99.99999999999998579 ) ) ;
#16484=( BOUNDED_CURVE ( )  B_SPLINE_CURVE ( 2, ( #18303, #10672, #12433, #147, #15267, #4923, #3149, #241, #1603 ),
 .UNSPECIFIED., .F., .F. ) 
 B_SPLINE_CURVE_WITH_KNOTS ( ( 3, 2, 2, 2, 3 ),
 ( 0.6041666666666666297, 0.6111111111111111605, 0.6250000000000000000, 0.6388888888888888395, 0.6458333333333332593 ),
 .UNSPECIFIED. ) 
 CURVE ( )  GEOMETRIC_REPRESENTATION_ITEM ( )  RATIONAL_B_SPLINE_CURVE ( ( 0.9330127018922192983, 0.9330127018922187432, 1.000000000000000000, 0.8660254037844387076, 1.000000000000000000, 0.8660254037844387076, 1.000000000000000000, 0.9330127018922198534, 0.9330127018922192983 ) ) 
 REPRESENTATION_ITEM ( '' )  );
#16486=CARTESIAN_POINT ( 'NONE',  ( -83.77821517812500929, -32.12812499938548427, 97.61286128772489690 ) ) ;
#16487=CARTESIAN_POINT ( 'NONE',  ( 80.90000000000000568, -33.69374999877096855, -97.40192378864668399 ) ) ;
#16489=CARTESIAN_POINT ( 'NONE',  ( -79.39999999999999147, -31.08750000000000213, -101.7320508075688821 ) ) ;
#16491=CARTESIAN_POINT ( 'NONE',  ( 79.39999999999999147, -33.73124999877096997, 101.7320508075688963 ) ) ;
#16492=CARTESIAN_POINT ( 'NONE',  ( -81.02178482187500208, -33.70312499938548711, -97.61286128772489690 ) ) ;
#16494=EDGE_CURVE ( 'NONE', #14497, #6753, #16198, .T. ) ;
#16498=VECTOR ( 'NONE', #18095, 1000.000000000000000 ) ;
#16500=CARTESIAN_POINT ( 'NONE',  ( 79.64356964374998427, -33.02812499938548285, 101.5914258081833879 ) ) ;
#16503=CARTESIAN_POINT ( 'NONE',  ( 85.40000000000000568, -34.93124999877096570, -98.26794919243111792 ) ) ;
#16511=EDGE_LOOP ( 'NONE', ( #2859, #11317, #14662, #11618 ) ) ;
#16512=CARTESIAN_POINT ( 'NONE',  ( -79.58826230849687988, -32.00000000000094502, 98.95399275615287138 ) ) ;
#16515=VERTEX_POINT ( 'NONE', #14809 ) ;
#16519=CARTESIAN_POINT ( 'NONE',  ( -81.02178482187500208, -33.10312499938548569, 97.61286128772489690 ) ) ;
#16524=CARTESIAN_POINT ( 'NONE',  ( -80.90000000000000568, -33.89999999999999858, 102.5980762113533018 ) ) ;
#16525=CARTESIAN_POINT ( 'NONE',  ( 80.90000000000000568, -34.64999999999999858, -97.40192378864668399 ) ) ;
#16526=DIRECTION ( 'NONE',  ( 0.000000000000000000, -1.000000000000000000, 0.000000000000000000 ) ) ;
#16527=CARTESIAN_POINT ( 'NONE',  ( -79.73531137350346398, -35.00000000000000000, -101.0054374292560908 ) ) ;
#16529=ORIENTED_EDGE ( 'NONE', *, *, #1284, .T. ) ;
#16531=CARTESIAN_POINT ( 'NONE',  ( -79.64356964374999848, -33.96562499938548285, -99.99999999999998579 ) ) ;
#16535=CARTESIAN_POINT ( 'NONE',  ( -84.70388354820684640, -35.00002705695768412, -101.9214814096701076 ) ) ;
#16537=CARTESIAN_POINT ( 'NONE',  ( 85.40000000000000568, -33.18750000000000000, -98.26794919243111792 ) ) ;
#16539=VERTEX_POINT ( 'NONE', #8946 ) ;
#16540=ADVANCED_FACE ( 'NONE', ( #6226 ), #2805, .T. ) ;
#16541=ORIENTED_EDGE ( 'NONE', *, *, #430, .T. ) ;
#16545=CARTESIAN_POINT ( 'NONE',  ( -79.39999999999999147, -31.93124999877096926, 98.26794919243110371 ) ) ;
#16546=CARTESIAN_POINT ( 'NONE',  ( 82.39999999999999147, -31.23750000000000071, 96.53589838486223584 ) ) ;
#16550=CARTESIAN_POINT ( 'NONE',  ( 80.60346964438562622, -31.99999999999999289, -97.67482724156225515 ) ) ;
#16551=CARTESIAN_POINT ( 'NONE',  ( 82.39999999999999147, -32.27812499938548285, -103.1828516163667899 ) ) ;
#16552=EDGE_LOOP ( 'NONE', ( #14263, #12775, #18896, #778 ) ) ;
#16554=CARTESIAN_POINT ( 'NONE',  ( 85.40000000000000568, -34.95000000000000284, -99.99999999999998579 ) ) ;
#16555=CARTESIAN_POINT ( 'NONE',  ( 79.64356964375001269, -32.20312499938548001, -101.5914258081833879 ) ) ;
#16556=FACE_OUTER_BOUND ( 'NONE', #1920, .T. ) ;
#16557=CARTESIAN_POINT ( 'NONE',  ( -81.59615242270662350, -34.57634618820329564, 96.99999999999997158 ) ) ;
#16558=CARTESIAN_POINT ( 'NONE',  ( 99.99999999999994316, -35.00000000000000000, 150.0000000000000000 ) ) ;
#16559=CARTESIAN_POINT ( 'NONE',  ( -79.39999999999999147, -30.71250000000000568, 101.7320508075688537 ) ) ;
#16564=CARTESIAN_POINT ( 'NONE',  ( 81.02178482187500208, -31.19062499938548427, 102.3871387122750889 ) ) ;
#16571=CARTESIAN_POINT ( 'NONE',  ( 83.77821517812500929, -30.66562499938548569, 102.3871387122750889 ) ) ;
#16575=CARTESIAN_POINT ( 'NONE',  ( -99.99999999999998579, -5.200000000000000178, -150.0000000000000000 ) ) ;
#16576=CARTESIAN_POINT ( 'NONE',  ( -83.77821517812500929, -31.97812499938548925, -97.61286128772489690 ) ) ;
#16578=CARTESIAN_POINT ( 'NONE',  ( 83.77821517812500929, -30.62812499938548783, 97.61286128772489690 ) ) ;
#16580=CARTESIAN_POINT ( 'NONE',  ( -79.64356964374999848, -32.72812499938548569, 99.99999999999998579 ) ) ;
#16582=EDGE_LOOP ( 'NONE', ( #3332, #11748, #7920, #494, #2228, #3626, #12589, #271, #2340, #7589, #5370, #8639, #6790, #12172, #13892, #19197, #13695 ) ) ;
#16583=CARTESIAN_POINT ( 'NONE',  ( -85.40000000000000568, -32.28750000000000142, -101.7320508075688679 ) ) ;
#16585=CARTESIAN_POINT ( 'NONE',  ( 85.40000000000000568, -34.89374999877097139, -99.99999999999998579 ) ) ;
#16586=CARTESIAN_POINT ( 'NONE',  ( -85.15643035624999868, -33.44062499938548427, -101.5914258081833879 ) ) ;
#16592=CARTESIAN_POINT ( 'NONE',  ( 83.77821517812500929, -33.36562499938548854, 102.3871387122750889 ) ) ;
#16593=CARTESIAN_POINT ( 'NONE',  ( 82.39999999999999147, -32.98124999877096286, 96.99999999999998579 ) ) ;
#16594=CARTESIAN_POINT ( 'NONE',  ( 85.40000000000000568, -32.70000000000000284, -99.99999999999998579 ) ) ;
#16595=CARTESIAN_POINT ( 'NONE',  ( 79.39999999999999147, -33.28124999877096712, -98.26794919243110371 ) ) ;
#16597=( BOUNDED_CURVE ( )  B_SPLINE_CURVE ( 2, ( #8935, #16277, #4548, #14901, #8843, #16186, #12066, #3076, #1529 ),
 .UNSPECIFIED., .F., .F. ) 
 B_SPLINE_CURVE_WITH_KNOTS ( ( 3, 2, 2, 2, 3 ),
 ( 0.3958333333333334259, 0.4027777777777777901, 0.4166666666666666852, 0.4305555555555555802, 0.4375000000000000555 ),
 .UNSPECIFIED. ) 
 CURVE ( )  GEOMETRIC_REPRESENTATION_ITEM ( )  RATIONAL_B_SPLINE_CURVE ( ( 0.9330127018922192983, 0.9330127018922200755, 1.000000000000000000, 0.8660254037844387076, 1.000000000000000000, 0.8660254037844387076, 1.000000000000000000, 0.9330127018922187432, 0.9330127018922192983 ) ) 
 REPRESENTATION_ITEM ( '' )  );
#16613=CARTESIAN_POINT ( 'NONE',  ( -85.15643035625001289, -34.75312499938548427, 99.99999999999998579 ) ) ;
#16616=CARTESIAN_POINT ( 'NONE',  ( -82.40000000000001990, -33.88124999877096855, 103.0000000000000000 ) ) ;
#16619=DIRECTION ( 'NONE',  ( 0.000000000000000000, -1.000000000000000000, 0.000000000000000000 ) ) ;
#16620=CARTESIAN_POINT ( 'NONE',  ( -79.60045861139946055, -34.99999999999998579, -100.3117415790902101 ) ) ;
#16623=CARTESIAN_POINT ( 'NONE',  ( -79.64356964375001269, -32.57812499938548001, -101.5914258081833879 ) ) ;
#16625=VECTOR ( 'NONE', #15561, 1000.000000000000000 ) ;
#16628=CARTESIAN_POINT ( 'NONE',  ( 99.99999999999994316, -21.80000000000003268, -139.9999999999999716 ) ) ;
#16636=CARTESIAN_POINT ( 'NONE',  ( -85.40000000000000568, -31.78124999877096712, 98.26794919243111792 ) ) ;
#16637=CARTESIAN_POINT ( 'NONE',  ( 83.90000000000000568, -30.82500000000000284, 97.40192378864668399 ) ) ;
#16638=CARTESIAN_POINT ( 'NONE',  ( 82.39999999999999147, -33.65624999877097423, 103.0000000000000000 ) ) ;
#16639=VECTOR ( 'NONE', #17266, 1000.000000000000000 ) ;
#16641=CARTESIAN_POINT ( 'NONE',  ( 85.15643035625001289, -32.09062499938548996, -98.40857419181659793 ) ) ;
#16642=CARTESIAN_POINT ( 'NONE',  ( 82.14831453747926560, -31.99999999999997868, -97.14155664246067090 ) ) ;
#16644=CARTESIAN_POINT ( 'NONE',  ( 82.39999999999999147, -34.30312499938548143, -96.81714838363319586 ) ) ;
#16648=CARTESIAN_POINT ( 'NONE',  ( -83.20395887649198130, -35.00000000000002842, 102.6365808225363025 ) ) ;
#16649=CARTESIAN_POINT ( 'NONE',  ( 79.64356964374999848, -32.61562499938548854, -99.99999999999998579 ) ) ;
#16653=CARTESIAN_POINT ( 'NONE',  ( -82.39999999999999147, -30.56250000000000355, 96.53589838486223584 ) ) ;
#16660=CARTESIAN_POINT ( 'NONE',  ( -85.40000000000000568, -33.11250000000000426, -98.26794919243111792 ) ) ;
#16663=CARTESIAN_POINT ( 'NONE',  ( 83.77821517812500929, -35.12812499938548427, 97.61286128772489690 ) ) ;
#16664=CARTESIAN_POINT ( 'NONE',  ( 85.15643035624999868, -32.91562499938549280, -101.5914258081833879 ) ) ;
#16666=CARTESIAN_POINT ( 'NONE',  ( -83.77821517812500929, -32.57812499938548711, 97.61286128772489690 ) ) ;
#16667=CARTESIAN_POINT ( 'NONE',  ( -79.64356964375001269, -33.14062499938548711, -101.5914258081833879 ) ) ;
#16669=CARTESIAN_POINT ( 'NONE',  ( 82.39999999999999147, -35.00624999877097565, 103.4641016151377499 ) ) ;
#16672=CARTESIAN_POINT ( 'NONE',  ( -79.64356964374999848, -30.92812499938548498, 99.99999999999998579 ) ) ;
#16673=( BOUNDED_SURFACE ( )  B_SPLINE_SURFACE ( 1, 2, ( 
 ( #15135, #7709, #9266, #4793, #13668, #12202, #15233, #1848, #12783, #18555, #15624, #5371, #6544, #11021, #2231, #3887, #8287, #9559, #2036, #9853, #14238, #5170, #8100, #12587, #14053, #687, #9954, #876, #3697, #11117, #15815, #17085, #18752, #3598, #2424, #12876, #7996, #15525, #8196, #11220, #6639, #6839, #8384, #973, #18848, #13953, #14335, #12489, #9664, #17375, #18459, #2142, #5470, #14146, #17185, #11415, #12681, #5080, #780, #17284, #3988, #6736, #9756, #594, #15719, #16986, #18655, #5274, #2324, #6928, #3789, #11318, #8765, #8859, #15909, #1256, #13254, #2609, #9256, #12972, #4276, #11512, #4084, #14622, #17475, #16295, #10240, #18942, #7115, #10046, #14716, #17858, #5565, #11888, #19227, #7203, #8569, #13070, #2904, #10332, #2708, #5940, #16204, #16004, #4470, #2514, #14523, #8471, #14428, #1157, #1441, #19034, #4374, #11695, #5658, #11601, #7297, #14814, #5843, #11796, #17569, #5746, #13157, #4181, #10141, #16101, #17766, #1062, #19128, #2810, #7395, #7018, #17664, #8668, #1354, #13358, #13736 ),
 ( #13540, #8952, #13450, #4860, #15109, #7496, #18147, #1636, #16769, #14920, #7782, #12179, #12081, #6418, #375, #9145, #1913, #1547, #3385, #7876, #3091, #13827, #87, #280, #469, #10804, #10711, #6231, #10521, #16489, #18339, #12373, #6327, #12279, #9334, #4769, #10423, #15300, #16386, #3282, #2996, #7681, #16676, #6038, #11987, #17954, #9239, #4564, #13635, #9052, #1724, #15017, #10617, #18243, #7590, #182, #15202, #6131, #1820, #18058, #4668, #16583, #3187, #11290, #6710, #662, #17161, #17260, #4960, #9641, #2300, #10997, #8360, #2011, #12657, #564, #12463, #3674, #6521, #5350, #18629, #7970, #15499, #18434, #3767, #6907, #13927, #952, #8265, #15600, #16963, #2113, #3865, #18729, #11092, #14314, #5246, #5052, #12854, #10903, #3574, #16869, #3475, #9534, #9827, #8073, #12761, #755, #14027, #6611, #15696, #15791, #14214, #851, #12560, #14118, #2208, #18530, #5146, #17061, #6814, #9435, #8169, #11196, #2398, #15401, #9732, #16251, #4518, #13501, #3050, #18010, #7638, #5797, #14773, #2860, #17352 ) ),
 .UNSPECIFIED., .F., .F., .F. ) 
 B_SPLINE_SURFACE_WITH_KNOTS ( ( 2, 2 ),
 ( 3, 2, 2, 2, 2, 2, 2, 2, 2, 2, 2, 2, 2, 2, 2, 2, 2, 2, 2, 2, 2, 2, 2, 2, 2, 2, 2, 2, 2, 2, 2, 2, 2, 2, 2, 2, 2, 2, 2, 2, 2, 2, 2, 2, 2, 2, 2, 2, 2, 2, 2, 2, 2, 2, 2, 2, 2, 2, 2, 2, 2, 2, 2, 2, 2, 2, 2, 2, 3 ),
 ( 0.000000000000000000, 1.000000000000000000 ),
 ( 0.000000000000000000, 0.01388888888888888812, 0.02777777777777777624, 0.04166666666666666435, 0.05555555555555555247, 0.06944444444444444753, 0.08333333333333332871, 0.09722222222222222376, 0.1111111111111111049, 0.1250000000000000000, 0.1388888888888888951, 0.1527777777777777901, 0.1666666666666666574, 0.1805555555555555525, 0.1944444444444444475, 0.2083333333333333426, 0.2222222222222222099, 0.2361111111111111049, 0.2500000000000000000, 0.2638888888888888951, 0.2777777777777777901, 0.2916666666666666852, 0.3055555555555555802, 0.3194444444444444198, 0.3333333333333333148, 0.3472222222222222099, 0.3611111111111111049, 0.3750000000000000000, 0.3888888888888888951, 0.4027777777777777901, 0.4166666666666666852, 0.4305555555555555802, 0.4444444444444444198, 0.4583333333333333148, 0.4722222222222222099, 0.4861111111111111049, 0.5000000000000000000, 0.5138888888888888395, 0.5277777777777777901, 0.5416666666666666297, 0.5555555555555555802, 0.5694444444444444198, 0.5833333333333333703, 0.5972222222222222099, 0.6111111111111111605, 0.6250000000000000000, 0.6388888888888888395, 0.6527777777777777901, 0.6666666666666666297, 0.6805555555555555802, 0.6944444444444444198, 0.7083333333333333703, 0.7222222222222222099, 0.7361111111111111605, 0.7500000000000000000, 0.7638888888888888395, 0.7777777777777777901, 0.7916666666666666297, 0.8055555555555555802, 0.8194444444444444198, 0.8333333333333333703, 0.8472222222222222099, 0.8611111111111111605, 0.8750000000000000000, 0.8888888888888888395, 0.9027777777777777901, 0.9166666666666666297, 0.9258785066912882389, 0.9351372917582011501 ),
 .UNSPECIFIED. ) 
 GEOMETRIC_REPRESENTATION_ITEM ( )  RATIONAL_B_SPLINE_SURFACE ( (
 ( 1.000000000000000000, 0.8660254037844387076, 1.000000000000000000, 0.8660254037844387076, 1.000000000000000000, 0.8660254037844387076, 1.000000000000000000, 0.8660254037844387076, 1.000000000000000000, 0.8660254037844387076, 1.000000000000000000, 0.8660254037844387076, 1.000000000000000000, 0.8660254037844387076, 1.000000000000000000, 0.8660254037844387076, 1.000000000000000000, 0.8660254037844387076, 1.000000000000000000, 0.8660254037844387076, 1.000000000000000000, 0.8660254037844387076, 1.000000000000000000, 0.8660254037844387076, 1.000000000000000000, 0.8660254037844387076, 1.000000000000000000, 0.8660254037844387076, 1.000000000000000000, 0.8660254037844387076, 1.000000000000000000, 0.8660254037844387076, 1.000000000000000000, 0.8660254037844387076, 1.000000000000000000, 0.8660254037844387076, 1.000000000000000000, 0.8660254037844387076, 1.000000000000000000, 0.8660254037844387076, 1.000000000000000000, 0.8660254037844387076, 1.000000000000000000, 0.8660254037844387076, 1.000000000000000000, 0.8660254037844387076, 1.000000000000000000, 0.8660254037844387076, 1.000000000000000000, 0.8660254037844387076, 1.000000000000000000, 0.8660254037844387076, 1.000000000000000000, 0.8660254037844387076, 1.000000000000000000, 0.8660254037844387076, 1.000000000000000000, 0.8660254037844387076, 1.000000000000000000, 0.8660254037844387076, 1.000000000000000000, 0.8660254037844387076, 1.000000000000000000, 0.8660254037844387076, 1.000000000000000000, 0.8660254037844387076, 1.000000000000000000, 0.8660254037844387076, 1.000000000000000000, 0.8660254037844387076, 1.000000000000000000, 0.8660254037844387076, 1.000000000000000000, 0.8660254037844387076, 1.000000000000000000, 0.8660254037844387076, 1.000000000000000000, 0.8660254037844387076, 1.000000000000000000, 0.8660254037844387076, 1.000000000000000000, 0.8660254037844387076, 1.000000000000000000, 0.8660254037844387076, 1.000000000000000000, 0.8660254037844387076, 1.000000000000000000, 0.8660254037844387076, 1.000000000000000000, 0.8660254037844387076, 1.000000000000000000, 0.8660254037844387076, 1.000000000000000000, 0.8660254037844387076, 1.000000000000000000, 0.8660254037844387076, 1.000000000000000000, 0.8660254037844387076, 1.000000000000000000, 0.8660254037844387076, 1.000000000000000000, 0.8660254037844387076, 1.000000000000000000, 0.8660254037844387076, 1.000000000000000000, 0.8660254037844387076, 1.000000000000000000, 0.8660254037844387076, 1.000000000000000000, 0.8660254037844387076, 1.000000000000000000, 0.8660254037844387076, 1.000000000000000000, 0.8660254037844387076, 1.000000000000000000, 0.8660254037844387076, 1.000000000000000000, 0.8660254037844387076, 1.000000000000000000, 0.8660254037844387076, 1.000000000000000000, 0.8660254037844387076, 1.000000000000000000, 0.8660254037844387076, 1.000000000000000000, 0.8660254037844387076, 1.000000000000000000, 0.8660254037844387076, 1.000000000000000000, 0.8660254037844387076, 1.000000000000000000, 0.8660254037844387076, 1.000000000000000000, 0.9111410165655264848, 0.9401539157124900736, 0.9401539157124900736, 0.9401539157124900736),
 ( 1.000000000000000000, 0.8660254037844387076, 1.000000000000000000, 0.8660254037844387076, 1.000000000000000000, 0.8660254037844387076, 1.000000000000000000, 0.8660254037844387076, 1.000000000000000000, 0.8660254037844387076, 1.000000000000000000, 0.8660254037844387076, 1.000000000000000000, 0.8660254037844387076, 1.000000000000000000, 0.8660254037844387076, 1.000000000000000000, 0.8660254037844387076, 1.000000000000000000, 0.8660254037844387076, 1.000000000000000000, 0.8660254037844387076, 1.000000000000000000, 0.8660254037844387076, 1.000000000000000000, 0.8660254037844387076, 1.000000000000000000, 0.8660254037844387076, 1.000000000000000000, 0.8660254037844387076, 1.000000000000000000, 0.8660254037844387076, 1.000000000000000000, 0.8660254037844387076, 1.000000000000000000, 0.8660254037844387076, 1.000000000000000000, 0.8660254037844387076, 1.000000000000000000, 0.8660254037844387076, 1.000000000000000000, 0.8660254037844387076, 1.000000000000000000, 0.8660254037844387076, 1.000000000000000000, 0.8660254037844387076, 1.000000000000000000, 0.8660254037844387076, 1.000000000000000000, 0.8660254037844387076, 1.000000000000000000, 0.8660254037844387076, 1.000000000000000000, 0.8660254037844387076, 1.000000000000000000, 0.8660254037844387076, 1.000000000000000000, 0.8660254037844387076, 1.000000000000000000, 0.8660254037844387076, 1.000000000000000000, 0.8660254037844387076, 1.000000000000000000, 0.8660254037844387076, 1.000000000000000000, 0.8660254037844387076, 1.000000000000000000, 0.8660254037844387076, 1.000000000000000000, 0.8660254037844387076, 1.000000000000000000, 0.8660254037844387076, 1.000000000000000000, 0.8660254037844387076, 1.000000000000000000, 0.8660254037844387076, 1.000000000000000000, 0.8660254037844387076, 1.000000000000000000, 0.8660254037844387076, 1.000000000000000000, 0.8660254037844387076, 1.000000000000000000, 0.8660254037844387076, 1.000000000000000000, 0.8660254037844387076, 1.000000000000000000, 0.8660254037844387076, 1.000000000000000000, 0.8660254037844387076, 1.000000000000000000, 0.8660254037844387076, 1.000000000000000000, 0.8660254037844387076, 1.000000000000000000, 0.8660254037844387076, 1.000000000000000000, 0.8660254037844387076, 1.000000000000000000, 0.8660254037844387076, 1.000000000000000000, 0.8660254037844387076, 1.000000000000000000, 0.8660254037844387076, 1.000000000000000000, 0.8660254037844387076, 1.000000000000000000, 0.8660254037844387076, 1.000000000000000000, 0.8660254037844387076, 1.000000000000000000, 0.8660254037844387076, 1.000000000000000000, 0.8660254037844387076, 1.000000000000000000, 0.8660254037844387076, 1.000000000000000000, 0.8660254037844387076, 1.000000000000000000, 0.8660254037844387076, 1.000000000000000000, 0.8660254037844387076, 1.000000000000000000, 0.8660254037844387076, 1.000000000000000000, 0.8660254037844387076, 1.000000000000000000, 0.8660254037844387076, 1.000000000000000000, 0.8660254037844387076, 1.000000000000000000, 0.8660254037844387076, 1.000000000000000000, 0.9111410165655264848, 0.9401539157124900736, 0.9401539157124900736, 0.9401539157124900736) ) ) 
 REPRESENTATION_ITEM ( '' )  SURFACE ( )  );
#16674=CARTESIAN_POINT ( 'NONE',  ( 82.39999999999999147, -33.20624999877097849, 102.9999999999999858 ) ) ;
#16676=CARTESIAN_POINT ( 'NONE',  ( -79.39999999999999147, -31.57499999999999929, -99.99999999999998579 ) ) ;
#16684=LINE ( 'NONE', #4869, #12423 ) ;
#16685=CARTESIAN_POINT ( 'NONE',  ( 79.39999999999999147, -32.86874999877097281, -99.99999999999998579 ) ) ;
#16686=CARTESIAN_POINT ( 'NONE',  ( 79.64356964374998427, -34.45312499938548711, 98.40857419181659793 ) ) ;
#16688=CARTESIAN_POINT ( 'NONE',  ( 82.39999999999999147, -33.20624999877097139, -96.53589838486223584 ) ) ;
#16701=ORIENTED_EDGE ( 'NONE', *, *, #13311, .F. ) ;
#16705=CIRCLE ( 'NONE', #2025, 5.199999999999996625 ) ;
#16710=( BOUNDED_CURVE ( )  B_SPLINE_CURVE ( 2, ( #13199, #1582, #10086, #13487, #17997, #1483, #17702, #16141, #4507 ),
 .UNSPECIFIED., .F., .F. ) 
 B_SPLINE_CURVE_WITH_KNOTS ( ( 3, 2, 2, 2, 3 ),
 ( 0.7291666666666666297, 0.7361111111111111605, 0.7500000000000000000, 0.7638888888888888395, 0.7708333333333331483 ),
 .UNSPECIFIED. ) 
 CURVE ( )  GEOMETRIC_REPRESENTATION_ITEM ( )  RATIONAL_B_SPLINE_CURVE ( ( 0.9330127018922192983, 0.9330127018922187432, 1.000000000000000000, 0.8660254037844387076, 1.000000000000000000, 0.8660254037844387076, 1.000000000000000000, 0.9330127018922209636, 0.9330127018922194093 ) ) 
 REPRESENTATION_ITEM ( '' )  );
#16716=CARTESIAN_POINT ( 'NONE',  ( -83.77821517812500929, -33.66562499938548569, -97.61286128772489690 ) ) ;
#16717=CARTESIAN_POINT ( 'NONE',  ( -81.59615242270665192, -32.77634618820330559, -103.0000000000000000 ) ) ;
#16719=VECTOR ( 'NONE', #15679, 1000.000000000000000 ) ;
#16721=DIRECTION ( 'NONE',  ( 0.000000000000000000, 0.000000000000000000, 1.000000000000000000 ) ) ;
#16723=ORIENTED_EDGE ( 'NONE', *, *, #7315, .T. ) ;
#16726=CARTESIAN_POINT ( 'NONE',  ( 79.39999999999999147, -31.16250000000000497, -101.7320508075688537 ) ) ;
#16728=CARTESIAN_POINT ( 'NONE',  ( -83.90000000000000568, -35.26874999877097139, 102.5980762113533018 ) ) ;
#16729=CARTESIAN_POINT ( 'NONE',  ( 79.39999999999999147, -32.43750000000000000, 101.7320508075688821 ) ) ;
#16733=CARTESIAN_POINT ( 'NONE',  ( 84.44763168836730927, -32.00000000000000711, -101.8452947671444093 ) ) ;
#16736=CARTESIAN_POINT ( 'NONE',  ( 85.15643035625001289, -32.84062499938548285, -99.99999999999998579 ) ) ;
#16739=CARTESIAN_POINT ( 'NONE',  ( -80.90000000000000568, -33.75000000000000000, 97.40192378864668399 ) ) ;
#16744=CARTESIAN_POINT ( 'NONE',  ( -82.39999999999999147, -31.01249999999999929, 96.53589838486223584 ) ) ;
#16748=CARTESIAN_POINT ( 'NONE',  ( 82.39999999999999147, -31.15312499938548640, 103.1828516163667899 ) ) ;
#16749=CARTESIAN_POINT ( 'NONE',  ( 85.16931825408417467, -32.00000000000002132, -100.2387112178441555 ) ) ;
#16753=CARTESIAN_POINT ( 'NONE',  ( 82.39999999999999147, -30.92812499938548143, 96.81714838363319586 ) ) ;
#16755=CARTESIAN_POINT ( 'NONE',  ( 79.64356964375001269, -30.89062499938548711, -98.40857419181659793 ) ) ;
#16757=CARTESIAN_POINT ( 'NONE',  ( -85.15643035625001289, -34.26562499938548711, 101.5914258081833879 ) ) ;
#16758=CARTESIAN_POINT ( 'NONE',  ( -81.02178482187500208, -32.65312499938548996, -102.3871387122750889 ) ) ;
#16760=ORIENTED_EDGE ( 'NONE', *, *, #6014, .T. ) ;
#16761=CARTESIAN_POINT ( 'NONE',  ( 85.15643035625001289, -30.70312499938548711, 99.99999999999998579 ) ) ;
#16762=VECTOR ( 'NONE', #6517, 1000.000000000000000 ) ;
#16765=CARTESIAN_POINT ( 'NONE',  ( -83.77821517812500929, -34.67812499938548854, 102.3871387122750889 ) ) ;
#16769=CARTESIAN_POINT ( 'NONE',  ( -80.90000000000000568, -30.30000000000000426, -97.40192378864668399 ) ) ;
#16771=CARTESIAN_POINT ( 'NONE',  ( 94.79999999999995453, -35.00000000000000000, 150.0000000000000000 ) ) ;
#16782=CARTESIAN_POINT ( 'NONE',  ( 82.39999999999999147, -34.52812499938548285, 96.81714838363319586 ) ) ;
#16785=CARTESIAN_POINT ( 'NONE',  ( 83.90000000000000568, -34.96874999877096712, -97.40192378864668399 ) ) ;
#16789=( BOUNDED_CURVE ( )  B_SPLINE_CURVE ( 2, ( #15705, #6622, #12571, #11004, #7981, #18443, #6430, #18738, #17069 ),
 .UNSPECIFIED., .F., .F. ) 
 B_SPLINE_CURVE_WITH_KNOTS ( ( 3, 2, 2, 2, 3 ),
 ( 0.5625000000000000000, 0.5694444444444444198, 0.5833333333333333703, 0.5972222222222222099, 0.6041666666666666297 ),
 .UNSPECIFIED. ) 
 CURVE ( )  GEOMETRIC_REPRESENTATION_ITEM ( )  RATIONAL_B_SPLINE_CURVE ( ( 0.9330127018922194093, 0.9330127018922194093, 1.000000000000000000, 0.8660254037844387076, 1.000000000000000000, 0.8660254037844387076, 1.000000000000000000, 0.9330127018922198534, 0.9330127018922192983 ) ) 
 REPRESENTATION_ITEM ( '' )  );
#16790=VERTEX_POINT ( 'NONE', #8446 ) ;
#16793=ADVANCED_FACE ( 'NONE', ( #10115, #8636 ), #11481, .T. ) ;
#16799=VERTEX_POINT ( 'NONE', #13039 ) ;
#16801=LINE ( 'NONE', #10831, #10976 ) ;
#16802=CARTESIAN_POINT ( 'NONE',  ( -83.90000000000000568, -34.12500000000000000, -102.5980762113533018 ) ) ;
#16805=CARTESIAN_POINT ( 'NONE',  ( -83.90000000000000568, -34.36874999877097281, -97.40192378864668399 ) ) ;
#16807=CARTESIAN_POINT ( 'NONE',  ( 82.40000000000000568, -30.00000000000000355, -103.0000000000000000 ) ) ;
#16811=DIRECTION ( 'NONE',  ( 0.000000000000000000, -1.000000000000000000, 0.000000000000000000 ) ) ;
#16824=FACE_BOUND ( 'NONE', #17286, .T. ) ;
#16826=CARTESIAN_POINT ( 'NONE',  ( 84.28136653320187577, -32.00000000000000000, -97.98546077809228905 ) ) ;
#16827=ORIENTED_EDGE ( 'NONE', *, *, #11389, .F. ) ;
#16829=ORIENTED_EDGE ( 'NONE', *, *, #14963, .F. ) ;
#16831=CARTESIAN_POINT ( 'NONE',  ( -81.68701737470171054, -32.00000000000000000, 102.8119722220549903 ) ) ;
#16832=CARTESIAN_POINT ( 'NONE',  ( 79.64356964375001269, -34.90312499938548285, -101.5914258081833879 ) ) ;
#16833=CARTESIAN_POINT ( 'NONE',  ( 69.99999999999998579, -34.99999999999999289, -150.0000000000000000 ) ) ;
#16835=CARTESIAN_POINT ( 'NONE',  ( -79.39999999999999147, -33.31874999877096855, 99.99999999999998579 ) ) ;
#16838=CARTESIAN_POINT ( 'NONE',  ( 85.15643035625001289, -32.50312499938548427, -99.99999999999998579 ) ) ;
#16839=CARTESIAN_POINT ( 'NONE',  ( 79.68063642052044315, -32.00000000000000711, -98.73478688827491112 ) ) ;
#16840=CARTESIAN_POINT ( 'NONE',  ( -81.02178482187500208, -33.59062499938548285, 102.3871387122750889 ) ) ;
#16841=CARTESIAN_POINT ( 'NONE',  ( 83.77821517812500929, -34.26562499938548711, -97.61286128772489690 ) ) ;
#16849=CARTESIAN_POINT ( 'NONE',  ( -85.40000000000000568, -33.11250000000000426, 101.7320508075688679 ) ) ;
#16850=VERTEX_POINT ( 'NONE', #14493 ) ;
#16852=CARTESIAN_POINT ( 'NONE',  ( 81.28488860390720561, -34.99999999999999289, 97.47285052570519781 ) ) ;
#16853=CARTESIAN_POINT ( 'NONE',  ( 81.02178482187500208, -32.69062499938548427, 97.61286128772489690 ) ) ;
#16857=CARTESIAN_POINT ( 'NONE',  ( 82.39999999999999147, -34.86562499938548854, 103.1828516163667899 ) ) ;
#16858=CARTESIAN_POINT ( 'NONE',  ( 83.77821517812500929, -30.77812499938548640, -97.61286128772489690 ) ) ;
#16860=CARTESIAN_POINT ( 'NONE',  ( -83.77821517812500929, -33.02812499938548285, 97.61286128772489690 ) ) ;
#16861=CARTESIAN_POINT ( 'NONE',  ( -79.64356964375001269, -34.56562499938549138, -98.40857419181659793 ) ) ;
#16863=CARTESIAN_POINT ( 'NONE',  ( 85.15643035625001289, -33.40312499938548285, 99.99999999999998579 ) ) ;
#16865=CARTESIAN_POINT ( 'NONE',  ( -83.77821517812500929, -32.01562499938548001, 97.61286128772489690 ) ) ;
#16866=CARTESIAN_POINT ( 'NONE',  ( -83.77821517812500929, -33.47812499938548569, 97.61286128772489690 ) ) ;
#16867=CARTESIAN_POINT ( 'NONE',  ( 83.90000000000000568, -33.16874999877096286, 102.5980762113533018 ) ) ;
#16868=ORIENTED_EDGE ( 'NONE', *, *, #18852, .T. ) ;
#16869=CARTESIAN_POINT ( 'NONE',  ( -79.39999999999999147, -33.78750000000000142, -101.7320508075688821 ) ) ;
#16872=CYLINDRICAL_SURFACE ( 'NONE', #2254, 3.000000000000002665 ) ;
#16873=CARTESIAN_POINT ( 'NONE',  ( 83.20384757729337366, -34.80134618820331127, -103.0000000000000000 ) ) ;
#16881=CARTESIAN_POINT ( 'NONE',  ( 85.40000000000000568, -34.48124999877096997, -98.26794919243111792 ) ) ;
#16884=CARTESIAN_POINT ( 'NONE',  ( 85.15643035625001289, -32.50312499938548427, -99.99999999999998579 ) ) ;
#16894=CARTESIAN_POINT ( 'NONE',  ( -82.40000000000000568, -33.03750000000000142, 102.9999999999999858 ) ) ;
#16897=CARTESIAN_POINT ( 'NONE',  ( -79.79868554281844695, -32.00000000000000711, 98.52838665780579674 ) ) ;
#16898=CARTESIAN_POINT ( 'NONE',  ( -80.90000000000000568, -33.69374999877096855, -102.5980762113533018 ) ) ;
#16900=ORIENTED_EDGE ( 'NONE', *, *, #1156, .F. ) ;
#16901=CARTESIAN_POINT ( 'NONE',  ( 79.64356964374998427, -32.24062499938548854, 101.5914258081833879 ) ) ;
#16902=CARTESIAN_POINT ( 'NONE',  ( -85.40000000000000568, -33.13124999877096855, -101.7320508075688679 ) ) ;
#16909=ORIENTED_EDGE ( 'NONE', *, *, #10312, .T. ) ;
#16912=CARTESIAN_POINT ( 'NONE',  ( -79.39999999999999147, -32.86874999877097281, -99.99999999999998579 ) ) ;
#16918=CARTESIAN_POINT ( 'NONE',  ( 94.79999999999995453, -5.200000000000000178, 150.0000000000000000 ) ) ;
#16919=AXIS2_PLACEMENT_3D ( 'NONE', #9757, #2710, #2326 ) ;
#16923=CARTESIAN_POINT ( 'NONE',  ( 79.39999999999999147, -33.35624999877096997, -101.7320508075688537 ) ) ;
#16924=CARTESIAN_POINT ( 'NONE',  ( 80.90000000000000568, -30.15000000000000213, -97.40192378864668399 ) ) ;
#16925=FACE_OUTER_BOUND ( 'NONE', #6703, .T. ) ;
#16926=CARTESIAN_POINT ( 'NONE',  ( -83.90000000000000568, -34.96874999877096712, 97.40192378864668399 ) ) ;
#16927=EDGE_CURVE ( 'NONE', #7532, #16539, #5367, .T. ) ;
#16928=CARTESIAN_POINT ( 'NONE',  ( -79.39999999999999147, -33.31874999877096855, 99.99999999999998579 ) ) ;
#16930=CARTESIAN_POINT ( 'NONE',  ( 82.39999999999999147, -33.96562499938548285, -96.81714838363319586 ) ) ;
#16931=CARTESIAN_POINT ( 'NONE',  ( -79.64356964375001269, -33.55312499938548854, 101.5914258081833879 ) ) ;
#16932=VECTOR ( 'NONE', #2236, 1000.000000000000000 ) ;
#16934=CARTESIAN_POINT ( 'NONE',  ( 83.77821517812500929, -34.56562499938548427, -102.3871387122750889 ) ) ;
#16935=ORIENTED_EDGE ( 'NONE', *, *, #19056, .F. ) ;
#16937=CARTESIAN_POINT ( 'NONE',  ( -85.40000000000000568, -34.46249999999999858, 101.7320508075688679 ) ) ;
#16941=CARTESIAN_POINT ( 'NONE',  ( -79.39999999999999147, -32.96250000000000568, 101.7320508075688537 ) ) ;
#16946=CARTESIAN_POINT ( 'NONE',  ( 79.64356964374999848, -32.61562499938548854, 99.99999999999998579 ) ) ;
#16947=CARTESIAN_POINT ( 'NONE',  ( 84.41281071784439405, -31.99999999999999289, -98.10821574224553387 ) ) ;
#16950=CARTESIAN_POINT ( 'NONE',  ( 79.64356964374999848, -34.07812499938548711, 99.99999999999998579 ) ) ;
#16951=CARTESIAN_POINT ( 'NONE',  ( 79.64356964374999848, -32.72812499938548569, -99.99999999999998579 ) ) ;
#16953=CARTESIAN_POINT ( 'NONE',  ( -81.02178482187500208, -33.55312499938548854, 97.61286128772489690 ) ) ;
#16954=CARTESIAN_POINT ( 'NONE',  ( -85.15643035625001289, -34.75312499938548427, -99.99999999999998579 ) ) ;
#16956=CARTESIAN_POINT ( 'NONE',  ( 83.77821517812500929, -32.57812499938548711, 102.3871387122750889 ) ) ;
#16959=CARTESIAN_POINT ( 'NONE',  ( -83.77821517812500929, -31.41562499938548569, 102.3871387122750889 ) ) ;
#16960=CARTESIAN_POINT ( 'NONE',  ( -81.02178482187500208, -34.60312499938549280, 102.3871387122750889 ) ) ;
#16962=ORIENTED_EDGE ( 'NONE', *, *, #7911, .F. ) ;
#16963=CARTESIAN_POINT ( 'NONE',  ( -79.39999999999999147, -33.37500000000000000, -99.99999999999998579 ) ) ;
#16965=LINE ( 'NONE', #3577, #13890 ) ;
#16966=DIRECTION ( 'NONE',  ( -1.000000000000000000, 4.625929269271494788E-16, 0.000000000000000000 ) ) ;
#16971=DIRECTION ( 'NONE',  ( -0.000000000000000000, -0.000000000000000000, -1.000000000000000000 ) ) ;
#16973=CARTESIAN_POINT ( 'NONE',  ( -82.40000000000000568, -30.00000000000000355, -103.0000000000000000 ) ) ;
#16975=CARTESIAN_POINT ( 'NONE',  ( 81.02178482187500208, -31.75312499938548427, -97.61286128772489690 ) ) ;
#16978=CARTESIAN_POINT ( 'NONE',  ( 79.39999999999999147, -31.51874999877096784, 99.99999999999998579 ) ) ;
#16986=CARTESIAN_POINT ( 'NONE',  ( -79.64356964375001269, -32.57812499938548001, -101.5914258081833879 ) ) ;
#16989=CARTESIAN_POINT ( 'NONE',  ( 83.77821517812500929, -33.92812499938548854, 102.3871387122750889 ) ) ;
#16990=CARTESIAN_POINT ( 'NONE',  ( -82.39999999999999147, -32.98124999877096997, -96.53589838486223584 ) ) ;
#16999=CARTESIAN_POINT ( 'NONE',  ( -81.59615242270662350, -34.12634618820329990, 96.99999999999998579 ) ) ;
#17002=ORIENTED_EDGE ( 'NONE', *, *, #8633, .T. ) ;
#17003=CARTESIAN_POINT ( 'NONE',  ( 79.64356964374999848, -33.06562499938548427, -99.99999999999998579 ) ) ;
#17007=VERTEX_POINT ( 'NONE', #11956 ) ;
#17008=CARTESIAN_POINT ( 'NONE',  ( 99.99999999999994316, -35.00000000000000000, 150.0000000000000000 ) ) ;
#17011=DIRECTION ( 'NONE',  ( -1.000000000000000000, 0.000000000000000000, 0.000000000000000000 ) ) ;
#17013=DIRECTION ( 'NONE',  ( -1.000000000000000000, 1.586032892321652285E-15, -0.000000000000000000 ) ) ;
#17016=CARTESIAN_POINT ( 'NONE',  ( -79.68596062386970402, -32.00000000000002132, 101.2782762865727619 ) ) ;
#17017=EDGE_CURVE ( 'NONE', #14982, #16515, #15222, .T. ) ;
#17018=CARTESIAN_POINT ( 'NONE',  ( 85.40000000000000568, -31.38749999999999574, -98.26794919243111792 ) ) ;
#17021=CARTESIAN_POINT ( 'NONE',  ( -83.90000000000000568, -34.51874999877097139, 97.40192378864668399 ) ) ;
#17023=CARTESIAN_POINT ( 'NONE',  ( 83.90000000000000568, -32.17500000000000426, -102.5980762113533018 ) ) ;
#17026=CARTESIAN_POINT ( 'NONE',  ( 83.77821517812500929, -32.57812499938548711, -97.61286128772489690 ) ) ;
#17027=CARTESIAN_POINT ( 'NONE',  ( 81.59615242270662350, -33.73259618943233562, 102.9999999999999858 ) ) ;
#17028=CARTESIAN_POINT ( 'NONE',  ( -85.15643035624999868, -34.15312499938548285, 101.5914258081833879 ) ) ;
#17030=CARTESIAN_POINT ( 'NONE',  ( 82.39999999999999147, -34.75312499938549138, -96.81714838363319586 ) ) ;
#17031=ORIENTED_EDGE ( 'NONE', *, *, #6014, .F. ) ;
#17032=CARTESIAN_POINT ( 'NONE',  ( 80.90000000000000568, -33.00000000000000000, 97.40192378864668399 ) ) ;
#17033=CARTESIAN_POINT ( 'NONE',  ( -80.90000000000000568, -33.30000000000000426, 97.40192378864668399 ) ) ;
#17037=EDGE_CURVE ( 'NONE', #11539, #518, #7464, .T. ) ;
#17039=CARTESIAN_POINT ( 'NONE',  ( -79.39999999999999147, -32.47500000000000142, 99.99999999999998579 ) ) ;
#17040=ORIENTED_EDGE ( 'NONE', *, *, #15091, .F. ) ;
#17043=CARTESIAN_POINT ( 'NONE',  ( 82.39999999999999147, -32.95312499938548711, 103.1828516163667899 ) ) ;
#17047=CARTESIAN_POINT ( 'NONE',  ( -81.02178482187500208, -32.80312499938548854, -97.61286128772489690 ) ) ;
#17048=CARTESIAN_POINT ( 'NONE',  ( 83.77821517812500929, -32.01562499938548001, 102.3871387122750889 ) ) ;
#17050=CARTESIAN_POINT ( 'NONE',  ( 82.39999999999999147, -31.26562499938549067, -96.81714838363319586 ) ) ;
#17052=CARTESIAN_POINT ( 'NONE',  ( -82.39999999999999147, -33.74062499938548854, 103.1828516163667899 ) ) ;
#17053=CARTESIAN_POINT ( 'NONE',  ( -85.15643035625001289, -34.30312499938548854, -99.99999999999998579 ) ) ;
#17054=VERTEX_POINT ( 'NONE', #15906 ) ;
#17055=CARTESIAN_POINT ( 'NONE',  ( 79.64356964375001269, -32.69062499938548427, 101.5914258081833879 ) ) ;
#17057=CARTESIAN_POINT ( 'NONE',  ( -85.15643035624999868, -31.90312499938548285, 101.5914258081833879 ) ) ;
#17058=CARTESIAN_POINT ( 'NONE',  ( -79.64356964375001269, -34.56562499938549138, 101.5914258081833879 ) ) ;
#17059=CARTESIAN_POINT ( 'NONE',  ( 82.39999999999999147, -34.83749999999999858, 97.00000000000000000 ) ) ;
#17061=CARTESIAN_POINT ( 'NONE',  ( -85.40000000000000568, -34.46249999999999858, -98.26794919243111792 ) ) ;
#17064=FACE_OUTER_BOUND ( 'NONE', #19230, .T. ) ;
#17068=CARTESIAN_POINT ( 'NONE',  ( 80.90000000000000568, -32.94374999877096855, -102.5980762113533018 ) ) ;
#17069=CARTESIAN_POINT ( 'NONE',  ( -82.39999999999999147, -33.65624999877097423, -103.0000000000000000 ) ) ;
#17070=CARTESIAN_POINT ( 'NONE',  ( 81.02178482187500208, -30.85312499938548569, 102.3871387122750889 ) ) ;
#17072=AXIS2_PLACEMENT_3D ( 'NONE', #1489, #10658, #15153 ) ;
#17073=CARTESIAN_POINT ( 'NONE',  ( 85.15643035625001289, -31.15312499938548996, -99.99999999999998579 ) ) ;
#17074=FACE_OUTER_BOUND ( 'NONE', #17430, .T. ) ;
#17076=CARTESIAN_POINT ( 'NONE',  ( 82.39999999999999147, -31.85624999877097352, 103.4641016151377499 ) ) ;
#17084=ORIENTED_EDGE ( 'NONE', *, *, #13639, .F. ) ;
#17085=CARTESIAN_POINT ( 'NONE',  ( -79.64356964375001269, -31.30312499938548854, -98.40857419181659793 ) ) ;
#17088=CARTESIAN_POINT ( 'NONE',  ( 79.64356964374998427, -32.76562499938548711, 98.40857419181659793 ) ) ;
#17090=CARTESIAN_POINT ( 'NONE',  ( -85.40000000000000568, -32.64374999877097139, -99.99999999999998579 ) ) ;
#17091=CARTESIAN_POINT ( 'NONE',  ( 85.40000000000000568, -34.08749999999999858, 101.7320508075688679 ) ) ;
#17095=CARTESIAN_POINT ( 'NONE',  ( 83.20395887649171129, -35.00000000000000711, -102.6365808225363878 ) ) ;
#17098=CARTESIAN_POINT ( 'NONE',  ( 79.39999999999999147, -30.58124999877096784, -98.26794919243110371 ) ) ;
#17101=CARTESIAN_POINT ( 'NONE',  ( 85.15643035625001289, -33.77812499938548285, -98.40857419181659793 ) ) ;
#17104=CARTESIAN_POINT ( 'NONE',  ( 84.44763168836730927, -32.00000000000000711, -101.8452947671444093 ) ) ;
#17105=ORIENTED_EDGE ( 'NONE', *, *, #8093, .T. ) ;
#17109=ORIENTED_EDGE ( 'NONE', *, *, #4755, .T. ) ;
#17112=ADVANCED_FACE ( 'NONE', ( #18939 ), #970, .F. ) ;
#17116=ORIENTED_EDGE ( 'NONE', *, *, #3753, .F. ) ;
#17117=CARTESIAN_POINT ( 'NONE',  ( 85.40000000000000568, -30.90000000000000213, -99.99999999999998579 ) ) ;
#17120=EDGE_CURVE ( 'NONE', #2466, #9248, #2705, .T. ) ;
#17121=CARTESIAN_POINT ( 'NONE',  ( -80.90000000000000568, -33.69374999877096855, 97.40192378864668399 ) ) ;
#17125=PLANE ( 'NONE',  #8307 ) ;
#17127=LINE ( 'NONE', #8134, #18053 ) ;
#17128=CARTESIAN_POINT ( 'NONE',  ( -81.02178482187500208, -32.09062499938548285, 97.61286128772489690 ) ) ;
#17131=CARTESIAN_POINT ( 'NONE',  ( -82.39999999999999147, -33.71249999999999858, 96.53589838486223584 ) ) ;
#17137=ADVANCED_FACE ( 'NONE', ( #16200 ), #9336, .F. ) ;
#17141=CARTESIAN_POINT ( 'NONE',  ( 81.02178482187500208, -32.54062499938548569, 102.3871387122750889 ) ) ;
#17146=CARTESIAN_POINT ( 'NONE',  ( 81.02178482187500208, -32.09062499938548285, 102.3871387122750889 ) ) ;
#17147=CARTESIAN_POINT ( 'NONE',  ( 84.51154815724953551, -35.25364861271051353, -98.22820072003833047 ) ) ;
#17149=CARTESIAN_POINT ( 'NONE',  ( -85.15643035625001289, -33.36562499938548854, 101.5914258081833879 ) ) ;
#17150=CARTESIAN_POINT ( 'NONE',  ( -81.02178482187500208, -31.79062499938548925, -97.61286128772489690 ) ) ;
#17152=CARTESIAN_POINT ( 'NONE',  ( 79.64356964374999848, -31.82812499938548356, 99.99999999999998579 ) ) ;
#17155=CARTESIAN_POINT ( 'NONE',  ( -85.15643035624999868, -31.52812499938547930, 98.40857419181659793 ) ) ;
#17156=CARTESIAN_POINT ( 'NONE',  ( -85.15643035624999868, -34.71562499938548285, 101.5914258081833879 ) ) ;
#17160=EDGE_CURVE ( 'NONE', #16515, #12559, #2749, .T. ) ;
#17161=CARTESIAN_POINT ( 'NONE',  ( -79.39999999999999147, -32.47500000000000142, -99.99999999999998579 ) ) ;
#17168=EDGE_CURVE ( 'NONE', #8568, #6753, #8510, .T. ) ;
#17169=CARTESIAN_POINT ( 'NONE',  ( 83.20384757729335945, -33.90134618820329848, -102.9999999999999716 ) ) ;
#17172=CARTESIAN_POINT ( 'NONE',  ( -99.99999999999998579, -29.80000000000000426, 150.0000000000000000 ) ) ;
#17175=CARTESIAN_POINT ( 'NONE',  ( 81.02178482187500208, -31.00312499938548783, -102.3871387122750889 ) ) ;
#17183=CARTESIAN_POINT ( 'NONE',  ( 82.40000000000000568, -33.93750000000000711, 97.00000000000000000 ) ) ;
#17184=ORIENTED_EDGE ( 'NONE', *, *, #5306, .T. ) ;
#17185=CARTESIAN_POINT ( 'NONE',  ( -79.64356964374999848, -32.16562499938548569, -99.99999999999998579 ) ) ;
#17186=DIRECTION ( 'NONE',  ( 0.000000000000000000, -1.000000000000000000, 0.000000000000000000 ) ) ;
#17187=ORIENTED_EDGE ( 'NONE', *, *, #15963, .T. ) ;
#17188=CARTESIAN_POINT ( 'NONE',  ( 81.02178482187500208, -34.45312499938548711, 102.3871387122750889 ) ) ;
#17189=CARTESIAN_POINT ( 'NONE',  ( -80.90000000000000568, -32.94374999877096855, -97.40192378864668399 ) ) ;
#17190=CARTESIAN_POINT ( 'NONE',  ( 79.39999999999999147, -34.27499999999999858, 99.99999999999998579 ) ) ;
#17194=CARTESIAN_POINT ( 'NONE',  ( -85.15643035625001289, -33.74062499938548854, -99.99999999999998579 ) ) ;
#17195=CARTESIAN_POINT ( 'NONE',  ( 82.40000000000000568, -34.10624999877096997, -96.99999999999998579 ) ) ;
#17196=CARTESIAN_POINT ( 'NONE',  ( -79.39999999999999147, -34.21874999877096712, 99.99999999999998579 ) ) ;
#17198=ORIENTED_EDGE ( 'NONE', *, *, #2420, .T. ) ;
#17199=CARTESIAN_POINT ( 'NONE',  ( 83.77821517812500929, -32.76562499938548711, -102.3871387122750889 ) ) ;
#17200=CARTESIAN_POINT ( 'NONE',  ( -85.15643035624999868, -35.05312499938548143, -98.40857419181659793 ) ) ;
#17206=CARTESIAN_POINT ( 'NONE',  ( 79.39999999999999147, -32.02500000000000568, 99.99999999999998579 ) ) ;
#17207=ORIENTED_EDGE ( 'NONE', *, *, #19070, .F. ) ;
#17210=ORIENTED_EDGE ( 'NONE', *, *, #12360, .T. ) ;
#17212=CARTESIAN_POINT ( 'NONE',  ( 85.40000000000000568, -32.21249999999999858, -101.7320508075688679 ) ) ;
#17214=CARTESIAN_POINT ( 'NONE',  ( -82.39999999999999147, -30.81562499938548427, 96.81714838363319586 ) ) ;
#17217=CARTESIAN_POINT ( 'NONE',  ( -83.90000000000000568, -32.11874999877097281, -97.40192378864668399 ) ) ;
#17220=CARTESIAN_POINT ( 'NONE',  ( -82.39999999999999147, -33.17812499938548854, 103.1828516163667899 ) ) ;
#17221=CARTESIAN_POINT ( 'NONE',  ( 82.39999999999999147, -34.97812499938547859, -103.1828516163667899 ) ) ;
#17224=CARTESIAN_POINT ( 'NONE',  ( 82.40000000000000568, -30.00000000000000355, -96.99999999999998579 ) ) ;
#17225=ADVANCED_FACE ( 'NONE', ( #1094 ), #4217, .T. ) ;
#17233=CARTESIAN_POINT ( 'NONE',  ( -80.80861089413674847, -34.99999999999999289, -97.72105564972109448 ) ) ;
#17235=CARTESIAN_POINT ( 'NONE',  ( 79.77811200999867935, -34.99999999999999289, 99.14934632385235602 ) ) ;
#17236=CARTESIAN_POINT ( 'NONE',  ( 82.39999999999999147, -32.50312499938548427, 103.1828516163667899 ) ) ;
#17238=EDGE_CURVE ( 'NONE', #9425, #2466, #8708, .T. ) ;
#17240=EDGE_CURVE ( 'NONE', #10655, #10520, #11412, .T. ) ;
#17243=CARTESIAN_POINT ( 'NONE',  ( -83.77821517812500929, -34.22812499938549280, -97.61286128772489690 ) ) ;
#17244=CARTESIAN_POINT ( 'NONE',  ( 81.02178482187500208, -31.79062499938548925, 97.61286128772489690 ) ) ;
#17245=CARTESIAN_POINT ( 'NONE',  ( 85.15643035624999868, -33.81562499938549138, -101.5914258081833879 ) ) ;
#17247=CARTESIAN_POINT ( 'NONE',  ( -81.02178482187500208, -33.59062499938548285, 102.3871387122750889 ) ) ;
#17248=CARTESIAN_POINT ( 'NONE',  ( -96.99999999999998579, -5.200000000000000178, 150.0000000000000000 ) ) ;
#17249=ADVANCED_FACE ( 'NONE', ( #16041 ), #1009, .F. ) ;
#17251=CARTESIAN_POINT ( 'NONE',  ( 82.39999999999999147, -32.84062499938548996, 96.81714838363319586 ) ) ;
#17255=CARTESIAN_POINT ( 'NONE',  ( -79.64356964375001269, -30.77812499938548285, 98.40857419181659793 ) ) ;
#17256=AXIS2_PLACEMENT_3D ( 'NONE', #4736, #4534, #10682 ) ;
#17257=CARTESIAN_POINT ( 'NONE',  ( -79.64356964375001269, -30.85312499938548569, 101.5914258081833879 ) ) ;
#17258=CARTESIAN_POINT ( 'NONE',  ( 85.40000000000000568, -34.91250000000000142, 98.26794919243111792 ) ) ;
#17260=CARTESIAN_POINT ( 'NONE',  ( -79.39999999999999147, -32.51250000000000284, -98.26794919243113213 ) ) ;
#17262=CARTESIAN_POINT ( 'NONE',  ( 94.79999999999995453, -29.80000000000000071, 150.0000000000000000 ) ) ;
#17263=CARTESIAN_POINT ( 'NONE',  ( 80.90000000000000568, -32.04374999877096997, -102.5980762113533018 ) ) ;
#17265=CARTESIAN_POINT ( 'NONE',  ( -84.12112955302457351, -35.00000000000000000, 97.53419980903896658 ) ) ;
#17266=DIRECTION ( 'NONE',  ( 0.000000000000000000, -1.000000000000000000, 0.000000000000000000 ) ) ;
#17267=CARTESIAN_POINT ( 'NONE',  ( 82.05869624310412291, -34.96883842999723413, 97.01420019955246232 ) ) ;
#17268=CARTESIAN_POINT ( 'NONE',  ( 82.39999999999999147, -31.26562499938549067, 103.1828516163667899 ) ) ;
#17272=DIRECTION ( 'NONE',  ( 0.000000000000000000, -1.000000000000000000, 0.000000000000000000 ) ) ;
#17273=CARTESIAN_POINT ( 'NONE',  ( 85.15643035624999868, -32.99062499938548854, -98.40857419181659793 ) ) ;
#17274=CARTESIAN_POINT ( 'NONE',  ( 81.59615242270665192, -32.77634618820330559, 103.0000000000000000 ) ) ;
#17275=ORIENTED_EDGE ( 'NONE', *, *, #9967, .F. ) ;
#17276=( BOUNDED_SURFACE ( )  B_SPLINE_SURFACE ( 1, 2, ( 
 ( #6654, #5091, #699, #5183, #9675, #17098, #8686, #17677, #14348, #8582, #4291, #13268, #18861, #16218, #1073, #1170, #6940, #19241, #7312, #9968, #17581, #10060, #13173, #10256, #4096, #15922, #1270, #8779, #2823, #16018, #10154, #984, #5482, #2620, #14536, #11428, #4003, #7031, #7128, #14636, #14732, #1367, #7217, #10344, #13080, #12985, #17390, #5858, #2723, #14440, #5579, #16115, #11812, #17780, #18955, #19143, #19048, #2525, #11526, #4388, #5671, #11614, #8485, #5759, #4192, #16310, #11710, #12890, #2918, #17489, #4680, #4783, #7697, #1739, #13554, #16688, #5, #16595, #13464, #6052, #6341, #196, #15029, #18258, #11999, #3201, #18069, #3297, #9160, #12191, #8871, #3106, #18160, #7795, #13372, #10725, #14935, #1651, #1456, #13749, #1835, #4483, #12096, #4580, #13653, #9254, #17968, #10436, #15124, #15219, #387, #296, #14829, #1560, #5954, #7409, #12292, #11903, #17874, #4875, #10818, #16503, #16785, #16402, #10630, #10536, #3010, #8968, #6244, #7507, #102, #9064, #7603, #6145, #7985 ),
 ( #11105, #13941, #9745, #5065, #2129, #579, #6625, #18742, #768, #8088, #14226, #12773, #675, #12479, #3778, #15313, #3687, #3587, #12386, #9448, #17175, #14040, #18447, #482, #17073, #12575, #865, #11008, #1926, #9547, #3399, #18542, #18641, #2218, #15613, #5158, #11210, #13840, #9653, #6533, #16975, #6828, #8183, #15513, #5361, #14133, #6722, #12668, #15710, #5264, #2312, #9350, #8276, #11304, #7890, #6434, #18353, #15413, #4976, #10917, #16884, #3487, #2023, #1146, #12961, #16090, #1243, #7007, #18839, #4172, #11686, #19118, #5646, #17273, #9940, #8373, #9840, #8753, #14326, #964, #16193, #14705, #5553, #5737, #7289, #7104, #14416, #7195, #17654, #8655, #2801, #13059, #8462, #13144, #1342, #2505, #19025, #18932, #1053, #6919, #11592, #11500, #4266, #17464, #15993, #4075, #17558, #13244, #14613, #2598, #19216, #5833, #14510, #10035, #10227, #15805, #10132, #8558, #2696, #3878, #2410, #12867, #5461, #11403, #17365, #3975, #15898, #11974, #6120, #1715, #7669, #12072, #7772, #17942, #17846 ) ),
 .UNSPECIFIED., .F., .F., .F. ) 
 B_SPLINE_SURFACE_WITH_KNOTS ( ( 2, 2 ),
 ( 3, 2, 2, 2, 2, 2, 2, 2, 2, 2, 2, 2, 2, 2, 2, 2, 2, 2, 2, 2, 2, 2, 2, 2, 2, 2, 2, 2, 2, 2, 2, 2, 2, 2, 2, 2, 2, 2, 2, 2, 2, 2, 2, 2, 2, 2, 2, 2, 2, 2, 2, 2, 2, 2, 2, 2, 2, 2, 2, 2, 2, 2, 2, 2, 2, 2, 2, 3 ),
 ( 0.000000000000000000, 1.000000000000000000 ),
 ( 0.000000000000000000, 0.01388888888888888812, 0.02777777777777777624, 0.04166666666666666435, 0.05555555555555555247, 0.06944444444444444753, 0.08333333333333332871, 0.09722222222222222376, 0.1111111111111111049, 0.1250000000000000000, 0.1388888888888888951, 0.1527777777777777901, 0.1666666666666666574, 0.1805555555555555525, 0.1944444444444444475, 0.2083333333333333426, 0.2222222222222222099, 0.2361111111111111049, 0.2500000000000000000, 0.2638888888888888951, 0.2777777777777777901, 0.2916666666666666852, 0.3055555555555555802, 0.3194444444444444198, 0.3333333333333333148, 0.3472222222222222099, 0.3611111111111111049, 0.3750000000000000000, 0.3888888888888888951, 0.4027777777777777901, 0.4166666666666666852, 0.4305555555555555802, 0.4444444444444444198, 0.4583333333333333148, 0.4722222222222222099, 0.4861111111111111049, 0.5000000000000000000, 0.5138888888888888395, 0.5277777777777777901, 0.5416666666666666297, 0.5555555555555555802, 0.5694444444444444198, 0.5833333333333333703, 0.5972222222222222099, 0.6111111111111111605, 0.6250000000000000000, 0.6388888888888888395, 0.6527777777777777901, 0.6666666666666666297, 0.6805555555555555802, 0.6944444444444444198, 0.7083333333333333703, 0.7222222222222222099, 0.7361111111111111605, 0.7500000000000000000, 0.7638888888888888395, 0.7777777777777777901, 0.7916666666666666297, 0.8055555555555555802, 0.8194444444444444198, 0.8333333333333333703, 0.8472222222222222099, 0.8611111111111111605, 0.8750000000000000000, 0.8888888888888888395, 0.9027777777777777901, 0.9166666666666666297, 0.9258785144422092550 ),
 .UNSPECIFIED. ) 
 GEOMETRIC_REPRESENTATION_ITEM ( )  RATIONAL_B_SPLINE_SURFACE ( (
 ( 1.000000000000000000, 0.8660254037844387076, 1.000000000000000000, 0.8660254037844387076, 1.000000000000000000, 0.8660254037844387076, 1.000000000000000000, 0.8660254037844387076, 1.000000000000000000, 0.8660254037844387076, 1.000000000000000000, 0.8660254037844387076, 1.000000000000000000, 0.8660254037844387076, 1.000000000000000000, 0.8660254037844387076, 1.000000000000000000, 0.8660254037844387076, 1.000000000000000000, 0.8660254037844387076, 1.000000000000000000, 0.8660254037844387076, 1.000000000000000000, 0.8660254037844387076, 1.000000000000000000, 0.8660254037844387076, 1.000000000000000000, 0.8660254037844387076, 1.000000000000000000, 0.8660254037844387076, 1.000000000000000000, 0.8660254037844387076, 1.000000000000000000, 0.8660254037844387076, 1.000000000000000000, 0.8660254037844387076, 1.000000000000000000, 0.8660254037844387076, 1.000000000000000000, 0.8660254037844387076, 1.000000000000000000, 0.8660254037844387076, 1.000000000000000000, 0.8660254037844387076, 1.000000000000000000, 0.8660254037844387076, 1.000000000000000000, 0.8660254037844387076, 1.000000000000000000, 0.8660254037844387076, 1.000000000000000000, 0.8660254037844387076, 1.000000000000000000, 0.8660254037844387076, 1.000000000000000000, 0.8660254037844387076, 1.000000000000000000, 0.8660254037844387076, 1.000000000000000000, 0.8660254037844387076, 1.000000000000000000, 0.8660254037844387076, 1.000000000000000000, 0.8660254037844387076, 1.000000000000000000, 0.8660254037844387076, 1.000000000000000000, 0.8660254037844387076, 1.000000000000000000, 0.8660254037844387076, 1.000000000000000000, 0.8660254037844387076, 1.000000000000000000, 0.8660254037844387076, 1.000000000000000000, 0.8660254037844387076, 1.000000000000000000, 0.8660254037844387076, 1.000000000000000000, 0.8660254037844387076, 1.000000000000000000, 0.8660254037844387076, 1.000000000000000000, 0.8660254037844387076, 1.000000000000000000, 0.8660254037844387076, 1.000000000000000000, 0.8660254037844387076, 1.000000000000000000, 0.8660254037844387076, 1.000000000000000000, 0.8660254037844387076, 1.000000000000000000, 0.8660254037844387076, 1.000000000000000000, 0.8660254037844387076, 1.000000000000000000, 0.8660254037844387076, 1.000000000000000000, 0.8660254037844387076, 1.000000000000000000, 0.8660254037844387076, 1.000000000000000000, 0.8660254037844387076, 1.000000000000000000, 0.8660254037844387076, 1.000000000000000000, 0.8660254037844387076, 1.000000000000000000, 0.8660254037844387076, 1.000000000000000000, 0.8660254037844387076, 1.000000000000000000, 0.8660254037844387076, 1.000000000000000000, 0.8660254037844387076, 1.000000000000000000, 0.8660254037844387076, 1.000000000000000000, 0.8660254037844387076, 1.000000000000000000, 0.8660254037844387076, 1.000000000000000000, 0.8660254037844387076, 1.000000000000000000, 0.8660254037844387076, 1.000000000000000000, 0.8660254037844387076, 1.000000000000000000, 0.8660254037844387076, 1.000000000000000000, 0.8660254037844387076, 1.000000000000000000, 0.9111409417988175496, 0.9401539645359766606),
 ( 1.000000000000000000, 0.8660254037844387076, 1.000000000000000000, 0.8660254037844387076, 1.000000000000000000, 0.8660254037844387076, 1.000000000000000000, 0.8660254037844387076, 1.000000000000000000, 0.8660254037844387076, 1.000000000000000000, 0.8660254037844387076, 1.000000000000000000, 0.8660254037844387076, 1.000000000000000000, 0.8660254037844387076, 1.000000000000000000, 0.8660254037844387076, 1.000000000000000000, 0.8660254037844387076, 1.000000000000000000, 0.8660254037844387076, 1.000000000000000000, 0.8660254037844387076, 1.000000000000000000, 0.8660254037844387076, 1.000000000000000000, 0.8660254037844387076, 1.000000000000000000, 0.8660254037844387076, 1.000000000000000000, 0.8660254037844387076, 1.000000000000000000, 0.8660254037844387076, 1.000000000000000000, 0.8660254037844387076, 1.000000000000000000, 0.8660254037844387076, 1.000000000000000000, 0.8660254037844387076, 1.000000000000000000, 0.8660254037844387076, 1.000000000000000000, 0.8660254037844387076, 1.000000000000000000, 0.8660254037844387076, 1.000000000000000000, 0.8660254037844387076, 1.000000000000000000, 0.8660254037844387076, 1.000000000000000000, 0.8660254037844387076, 1.000000000000000000, 0.8660254037844387076, 1.000000000000000000, 0.8660254037844387076, 1.000000000000000000, 0.8660254037844387076, 1.000000000000000000, 0.8660254037844387076, 1.000000000000000000, 0.8660254037844387076, 1.000000000000000000, 0.8660254037844387076, 1.000000000000000000, 0.8660254037844387076, 1.000000000000000000, 0.8660254037844387076, 1.000000000000000000, 0.8660254037844387076, 1.000000000000000000, 0.8660254037844387076, 1.000000000000000000, 0.8660254037844387076, 1.000000000000000000, 0.8660254037844387076, 1.000000000000000000, 0.8660254037844387076, 1.000000000000000000, 0.8660254037844387076, 1.000000000000000000, 0.8660254037844387076, 1.000000000000000000, 0.8660254037844387076, 1.000000000000000000, 0.8660254037844387076, 1.000000000000000000, 0.8660254037844387076, 1.000000000000000000, 0.8660254037844387076, 1.000000000000000000, 0.8660254037844387076, 1.000000000000000000, 0.8660254037844387076, 1.000000000000000000, 0.8660254037844387076, 1.000000000000000000, 0.8660254037844387076, 1.000000000000000000, 0.8660254037844387076, 1.000000000000000000, 0.8660254037844387076, 1.000000000000000000, 0.8660254037844387076, 1.000000000000000000, 0.8660254037844387076, 1.000000000000000000, 0.8660254037844387076, 1.000000000000000000, 0.8660254037844387076, 1.000000000000000000, 0.8660254037844387076, 1.000000000000000000, 0.8660254037844387076, 1.000000000000000000, 0.8660254037844387076, 1.000000000000000000, 0.8660254037844387076, 1.000000000000000000, 0.8660254037844387076, 1.000000000000000000, 0.8660254037844387076, 1.000000000000000000, 0.8660254037844387076, 1.000000000000000000, 0.8660254037844387076, 1.000000000000000000, 0.8660254037844387076, 1.000000000000000000, 0.8660254037844387076, 1.000000000000000000, 0.8660254037844387076, 1.000000000000000000, 0.9111409417988175496, 0.9401539645359766606) ) ) 
 REPRESENTATION_ITEM ( '' )  SURFACE ( )  );
#17277=CARTESIAN_POINT ( 'NONE',  ( 85.40000000000000568, -31.29374999877096997, 99.99999999999998579 ) ) ;
#17280=CARTESIAN_POINT ( 'NONE',  ( 85.40000000000000568, -34.50000000000000000, 99.99999999999998579 ) ) ;
#17284=CARTESIAN_POINT ( 'NONE',  ( -85.15643035624999868, -32.35312499938549280, -98.40857419181659793 ) ) ;
#17285=CARTESIAN_POINT ( 'NONE',  ( 85.40000000000000568, -33.11250000000000426, 98.26794919243111792 ) ) ;
#17286=EDGE_LOOP ( 'NONE', ( #3735, #7424, #6157, #38 ) ) ;
#17287=CARTESIAN_POINT ( 'NONE',  ( 82.39999999999999147, -32.39062499938548711, 96.81714838363319586 ) ) ;
#17288=CARTESIAN_POINT ( 'NONE',  ( -83.77821517812500929, -30.62812499938548783, -97.61286128772489690 ) ) ;
#17289=CARTESIAN_POINT ( 'NONE',  ( 85.40000000000000568, -34.05000000000000426, 99.99999999999998579 ) ) ;
#17293=CARTESIAN_POINT ( 'NONE',  ( -79.64356964374998427, -32.12812499938548427, -101.5914258081833879 ) ) ;
#17294=CARTESIAN_POINT ( 'NONE',  ( -82.40000000000000568, -34.10624999877096997, -102.9999999999999858 ) ) ;
#17295=LINE ( 'NONE', #3709, #4781 ) ;
#17297=EDGE_LOOP ( 'NONE', ( #2527, #18476, #15925, #9458 ) ) ;
#17298=CARTESIAN_POINT ( 'NONE',  ( 79.64356964374999848, -33.51562499938548711, -99.99999999999998579 ) ) ;
#17302=CARTESIAN_POINT ( 'NONE',  ( 85.40000000000000568, -32.66250000000000142, 98.26794919243111792 ) ) ;
#17305=ORIENTED_EDGE ( 'NONE', *, *, #17735, .F. ) ;
#17306=CARTESIAN_POINT ( 'NONE',  ( -83.20384757729335945, -34.08615380933863293, -102.9999999999999858 ) ) ;
#17308=VERTEX_POINT ( 'NONE', #5977 ) ;
#17309=( BOUNDED_CURVE ( )  B_SPLINE_CURVE ( 2, ( #3171, #10409, #10604, #9222, #68, #4359, #10696, #6116, #1804 ),
 .UNSPECIFIED., .F., .F. ) 
 B_SPLINE_CURVE_WITH_KNOTS ( ( 3, 2, 2, 2, 3 ),
 ( 0.4375000000000000555, 0.4444444444444444198, 0.4583333333333333148, 0.4722222222222222099, 0.4791666666666666297 ),
 .UNSPECIFIED. ) 
 CURVE ( )  GEOMETRIC_REPRESENTATION_ITEM ( )  RATIONAL_B_SPLINE_CURVE ( ( 0.9330127018922192983, 0.9330127018922198534, 1.000000000000000000, 0.8660254037844387076, 1.000000000000000000, 0.8660254037844387076, 1.000000000000000000, 0.9330127018922196314, 0.9330127018922194093 ) ) 
 REPRESENTATION_ITEM ( '' )  );
#17310=DIRECTION ( 'NONE',  ( -1.000000000000000000, -0.000000000000000000, 0.000000000000000000 ) ) ;
#17311=CARTESIAN_POINT ( 'NONE',  ( 79.39999999999999147, -33.78750000000000142, -98.26794919243110371 ) ) ;
#17313=CARTESIAN_POINT ( 'NONE',  ( -83.77821517812500929, -31.22812499938548569, 97.61286128772489690 ) ) ;
#17317=CARTESIAN_POINT ( 'NONE',  ( 84.05108659120818970, -32.00820041275124339, 102.2295963284773563 ) ) ;
#17318=CARTESIAN_POINT ( 'NONE',  ( 81.59615242270662350, -33.91740381056766296, 96.99999999999997158 ) ) ;
#17319=CARTESIAN_POINT ( 'NONE',  ( 83.43443729601550274, -34.99999999999999289, 97.42249611015769517 ) ) ;
#17321=EDGE_LOOP ( 'NONE', ( #655, #8225, #620, #11723 ) ) ;
#17324=FACE_OUTER_BOUND ( 'NONE', #15712, .T. ) ;
#17332=CARTESIAN_POINT ( 'NONE',  ( 84.28136653320183314, -32.00000000000000711, 102.0145392219077394 ) ) ;
#17333=CARTESIAN_POINT ( 'NONE',  ( 82.39999999999999147, -30.11250000000000426, 103.4641016151377499 ) ) ;
#17335=AXIS2_PLACEMENT_3D ( 'NONE', #12907, #15936, #15651 ) ;
#17338=CARTESIAN_POINT ( 'NONE',  ( -81.02178482187500208, -34.60312499938549280, -97.61286128772489690 ) ) ;
#17339=CARTESIAN_POINT ( 'NONE',  ( 85.15643035624999868, -31.07812499938548356, 101.5914258081833879 ) ) ;
#17340=( BOUNDED_CURVE ( )  B_SPLINE_CURVE ( 2, ( #15462, #3539, #17217, #436, #15752, #6381, #5207, #8029, #6477 ),
 .UNSPECIFIED., .F., .F. ) 
 B_SPLINE_CURVE_WITH_KNOTS ( ( 3, 2, 2, 2, 3 ),
 ( 0.3125000000000001665, 0.3194444444444444198, 0.3333333333333333148, 0.3472222222222222099, 0.3541666666666666297 ),
 .UNSPECIFIED. ) 
 CURVE ( )  GEOMETRIC_REPRESENTATION_ITEM ( )  RATIONAL_B_SPLINE_CURVE ( ( 0.9330127018922194093, 0.9330127018922209636, 1.000000000000000000, 0.8660254037844387076, 1.000000000000000000, 0.8660254037844387076, 1.000000000000000000, 0.9330127018922196314, 0.9330127018922194093 ) ) 
 REPRESENTATION_ITEM ( '' )  );
#17341=CARTESIAN_POINT ( 'NONE',  ( 82.39999999999999147, -34.86562499938548854, -96.81714838363319586 ) ) ;
#17343=CARTESIAN_POINT ( 'NONE',  ( -79.64356964374998427, -34.37812499938548427, 98.40857419181659793 ) ) ;
#17344=CARTESIAN_POINT ( 'NONE',  ( 79.64356964375001269, -31.30312499938548854, -101.5914258081833879 ) ) ;
#17346=CARTESIAN_POINT ( 'NONE',  ( -82.40000000000000568, -30.00000000000000355, -96.99999999999998579 ) ) ;
#17349=CARTESIAN_POINT ( 'NONE',  ( -79.64356964374999848, -33.96562499938548285, 99.99999999999998579 ) ) ;
#17350=CARTESIAN_POINT ( 'NONE',  ( -83.77821517812500929, -31.11562499938548498, 97.61286128772489690 ) ) ;
#17352=CARTESIAN_POINT ( 'NONE',  ( -83.33080762004576059, -35.05289549976084373, -103.5578907812544855 ) ) ;
#17357=EDGE_CURVE ( 'NONE', #9562, #14525, #6747, .T. ) ;
#17362=AXIS2_PLACEMENT_3D ( 'NONE', #11918, #17891, #13284 ) ;
#17364=LINE ( 'NONE', #3974, #2147 ) ;
#17365=CARTESIAN_POINT ( 'NONE',  ( 81.02178482187500208, -34.90312499938548285, -97.61286128772489690 ) ) ;
#17368=CARTESIAN_POINT ( 'NONE',  ( 82.39999999999999147, -32.30624999877097281, 103.4641016151377499 ) ) ;
#17373=DIRECTION ( 'NONE',  ( 0.000000000000000000, 0.000000000000000000, -1.000000000000000000 ) ) ;
#17375=CARTESIAN_POINT ( 'NONE',  ( -85.15643035624999868, -31.97812499938548925, -101.5914258081833879 ) ) ;
#17376=EDGE_CURVE ( 'NONE', #2879, #13090, #12023, .T. ) ;
#17378=VERTEX_POINT ( 'NONE', #4506 ) ;
#17379=CARTESIAN_POINT ( 'NONE',  ( 85.15643035625001289, -32.91562499938548569, 98.40857419181659793 ) ) ;
#17380=CARTESIAN_POINT ( 'NONE',  ( -85.15643035625001289, -31.60312499938548569, -99.99999999999998579 ) ) ;
#17381=CARTESIAN_POINT ( 'NONE',  ( 85.40000000000000568, -34.46249999999999858, 98.26794919243111792 ) ) ;
#17386=CARTESIAN_POINT ( 'NONE',  ( -79.64356964374999848, -33.51562499938548711, -99.99999999999998579 ) ) ;
#17390=CARTESIAN_POINT ( 'NONE',  ( 83.90000000000000568, -32.11874999877097281, -102.5980762113533018 ) ) ;
#17394=CARTESIAN_POINT ( 'NONE',  ( 79.64356964374999848, -32.61562499938548854, -99.99999999999998579 ) ) ;
#17397=( BOUNDED_CURVE ( )  B_SPLINE_CURVE ( 2, ( #18300, #3443, #6774, #5115, #9396, #8132, #10960, #12722, #4919 ),
 .UNSPECIFIED., .F., .F. ) 
 B_SPLINE_CURVE_WITH_KNOTS ( ( 3, 2, 2, 2, 3 ),
 ( 0.5208333333333334814, 0.5277777777777777901, 0.5416666666666666297, 0.5555555555555555802, 0.5625000000000000000 ),
 .UNSPECIFIED. ) 
 CURVE ( )  GEOMETRIC_REPRESENTATION_ITEM ( )  RATIONAL_B_SPLINE_CURVE ( ( 0.9330127018922194093, 0.9330127018922209636, 1.000000000000000000, 0.8660254037844387076, 1.000000000000000000, 0.8660254037844387076, 1.000000000000000000, 0.9330127018922194093, 0.9330127018922194093 ) ) 
 REPRESENTATION_ITEM ( '' )  );
#17400=AXIS2_PLACEMENT_3D ( 'NONE', #7135, #16024, #2247 ) ;
#17407=CARTESIAN_POINT ( 'NONE',  ( 83.90000000000000568, -32.62500000000000000, -102.5980762113533018 ) ) ;
#17408=EDGE_CURVE ( 'NONE', #12671, #18799, #1765, .T. ) ;
#17409=CARTESIAN_POINT ( 'NONE',  ( 79.79666399293472523, -31.99999999999998579, -101.4892189721552427 ) ) ;
#17411=CARTESIAN_POINT ( 'NONE',  ( -82.39999999999999147, -31.49062499938548854, 103.1828516163667899 ) ) ;
#17415=CARTESIAN_POINT ( 'NONE',  ( 81.02178482187500208, -32.09062499938548285, 102.3871387122750889 ) ) ;
#17417=EDGE_CURVE ( 'NONE', #13089, #10928, #13337, .T. ) ;
#17418=CARTESIAN_POINT ( 'NONE',  ( 79.77811200999867935, -34.99999999999999289, 99.14934632385235602 ) ) ;
#17419=CARTESIAN_POINT ( 'NONE',  ( -82.39999999999999147, -34.52812499938548996, 103.1828516163667899 ) ) ;
#17420=CARTESIAN_POINT ( 'NONE',  ( 85.15643035625001289, -35.09062499938548285, -99.99999999999998579 ) ) ;
#17422=CARTESIAN_POINT ( 'NONE',  ( 81.59615242270662350, -33.01740381056767148, 96.99999999999998579 ) ) ;
#17425=( BOUNDED_CURVE ( )  B_SPLINE_CURVE ( 2, ( #1777, #6472, #15555, #3238, #9589, #16923, #12330, #4821, #10761 ),
 .UNSPECIFIED., .F., .F. ) 
 B_SPLINE_CURVE_WITH_KNOTS ( ( 3, 2, 2, 2, 3 ),
 ( 0.5208333333333334814, 0.5277777777777777901, 0.5416666666666666297, 0.5555555555555555802, 0.5625000000000000000 ),
 .UNSPECIFIED. ) 
 CURVE ( )  GEOMETRIC_REPRESENTATION_ITEM ( )  RATIONAL_B_SPLINE_CURVE ( ( 0.9330127018922194093, 0.9330127018922209636, 1.000000000000000000, 0.8660254037844387076, 1.000000000000000000, 0.8660254037844387076, 1.000000000000000000, 0.9330127018922194093, 0.9330127018922194093 ) ) 
 REPRESENTATION_ITEM ( '' )  );
#17430=EDGE_LOOP ( 'NONE', ( #6001, #12473, #18874, #2538 ) ) ;
#17433=DIRECTION ( 'NONE',  ( 0.000000000000000000, 0.000000000000000000, -1.000000000000000000 ) ) ;
#17434=CARTESIAN_POINT ( 'NONE',  ( 79.64356964374999848, -33.96562499938548285, 99.99999999999998579 ) ) ;
#17435=CARTESIAN_POINT ( 'NONE',  ( 82.65333140691205926, -34.99995246259152282, -97.01071553687880566 ) ) ;
#17439=CARTESIAN_POINT ( 'NONE',  ( -85.15643035625001289, -34.79062499938548569, -101.5914258081833879 ) ) ;
#17440=CARTESIAN_POINT ( 'NONE',  ( 82.39999999999999147, -33.17812499938548854, 96.81714838363319586 ) ) ;
#17441=CARTESIAN_POINT ( 'NONE',  ( 81.02178482187500208, -34.15312499938548285, -102.3871387122750889 ) ) ;
#17443=CARTESIAN_POINT ( 'NONE',  ( -79.64356964374999848, -32.61562499938548854, 99.99999999999998579 ) ) ;
#17444=CARTESIAN_POINT ( 'NONE',  ( 79.64356964374999848, -30.36562499938548498, -99.99999999999998579 ) ) ;
#17446=CARTESIAN_POINT ( 'NONE',  ( 79.64356964374999848, -34.52812499938548285, 99.99999999999998579 ) ) ;
#17449=CARTESIAN_POINT ( 'NONE',  ( -81.02178482187500208, -34.04062499938548569, 102.3871387122750889 ) ) ;
#17450=CARTESIAN_POINT ( 'NONE',  ( -85.15643035625001289, -30.14062499938548711, 99.99999999999998579 ) ) ;
#17452=LINE ( 'NONE', #15888, #4948 ) ;
#17454=CARTESIAN_POINT ( 'NONE',  ( 79.67114894419047744, -35.00000000000000711, -99.22311565912301035 ) ) ;
#17456=( BOUNDED_CURVE ( )  B_SPLINE_CURVE ( 2, ( #14322, #12769, #14413, #2217, #961, #11497, #18637, #7099, #1141 ),
 .UNSPECIFIED., .F., .F. ) 
 B_SPLINE_CURVE_WITH_KNOTS ( ( 3, 2, 2, 2, 3 ),
 ( 0.4791666666666666297, 0.4861111111111111049, 0.5000000000000000000, 0.5138888888888888395, 0.5208333333333334814 ),
 .UNSPECIFIED. ) 
 CURVE ( )  GEOMETRIC_REPRESENTATION_ITEM ( )  RATIONAL_B_SPLINE_CURVE ( ( 0.9330127018922194093, 0.9330127018922190762, 1.000000000000000000, 0.8660254037844387076, 1.000000000000000000, 0.8660254037844387076, 1.000000000000000000, 0.9330127018922177440, 0.9330127018922194093 ) ) 
 REPRESENTATION_ITEM ( '' )  );
#17457=CARTESIAN_POINT ( 'NONE',  ( -83.20384757729335945, -34.40759618943233988, 102.9999999999999858 ) ) ;
#17458=CARTESIAN_POINT ( 'NONE',  ( -82.65333140691201663, -34.99995246259153703, 97.01071553687880566 ) ) ;
#17459=CARTESIAN_POINT ( 'NONE',  ( -81.59615242270662350, -33.41115380933863577, -96.99999999999998579 ) ) ;
#17461=CARTESIAN_POINT ( 'NONE',  ( 82.39999999999999147, -30.36562499938549209, 103.1828516163667899 ) ) ;
#17463=CARTESIAN_POINT ( 'NONE',  ( -83.90000000000000568, -32.71874999877096712, -102.5980762113533018 ) ) ;
#17464=CARTESIAN_POINT ( 'NONE',  ( 79.64356964375001269, -34.11562499938548854, -101.5914258081833879 ) ) ;
#17467=CARTESIAN_POINT ( 'NONE',  ( 82.39999999999999147, -32.98124999877096997, 96.53589838486223584 ) ) ;
#17473=CARTESIAN_POINT ( 'NONE',  ( 82.40000000000001990, -34.16250000000000853, 103.0000000000000000 ) ) ;
#17475=CARTESIAN_POINT ( 'NONE',  ( -85.15643035625001289, -33.29062499938547859, -99.99999999999998579 ) ) ;
#17478=DIRECTION ( 'NONE',  ( 1.000000000000000000, 0.000000000000000000, -0.000000000000000000 ) ) ;
#17479=CARTESIAN_POINT ( 'NONE',  ( -79.64356964375001269, -31.41562499938548569, -98.40857419181659793 ) ) ;
#17480=CARTESIAN_POINT ( 'NONE',  ( 84.01447415327271528, -35.02670941564510088, 102.7431224211893692 ) ) ;
#17487=CARTESIAN_POINT ( 'NONE',  ( -94.79999999999999716, -5.200000000000000178, 150.0000000000000000 ) ) ;
#17489=CARTESIAN_POINT ( 'NONE',  ( 82.39999999999999147, -32.98124999877096997, -103.4641016151377499 ) ) ;
#17497=ORIENTED_EDGE ( 'NONE', *, *, #15097, .T. ) ;
#17498=ORIENTED_EDGE ( 'NONE', *, *, #7465, .F. ) ;
#17500=CARTESIAN_POINT ( 'NONE',  ( -83.90000000000000568, -32.11874999877097281, 102.5980762113533018 ) ) ;
#17501=ORIENTED_EDGE ( 'NONE', *, *, #18203, .T. ) ;
#17503=CARTESIAN_POINT ( 'NONE',  ( 82.39999999999999147, -31.68750000000000355, -103.4641016151377499 ) ) ;
#17504=CARTESIAN_POINT ( 'NONE',  ( -82.39999999999999147, -33.65624999877097423, -103.0000000000000000 ) ) ;
#17505=CARTESIAN_POINT ( 'NONE',  ( -79.64356964375001269, -32.76562499938548711, 101.5914258081833879 ) ) ;
#17515=CARTESIAN_POINT ( 'NONE',  ( -83.77821517812500929, -31.86562499938548498, -97.61286128772489690 ) ) ;
#17517=CARTESIAN_POINT ( 'NONE',  ( 69.99999999999998579, -34.99999999999999289, -150.0000000000000000 ) ) ;
#17520=CARTESIAN_POINT ( 'NONE',  ( 79.39999999999999147, -32.43750000000000000, 101.7320508075688963 ) ) ;
#17526=CARTESIAN_POINT ( 'NONE',  ( 80.90000000000000568, -30.30000000000000426, 97.40192378864668399 ) ) ;
#17527=FACE_OUTER_BOUND ( 'NONE', #449, .T. ) ;
#17531=CARTESIAN_POINT ( 'NONE',  ( -79.64356964374998427, -33.14062499938548711, -101.5914258081833879 ) ) ;
#17532=CARTESIAN_POINT ( 'NONE',  ( 85.15643035624999868, -34.15312499938548285, 98.40857419181659793 ) ) ;
#17533=CARTESIAN_POINT ( 'NONE',  ( 85.15643035624999868, -35.16562499938547859, -101.5914258081833879 ) ) ;
#17535=CARTESIAN_POINT ( 'NONE',  ( -85.15643035625001289, -32.39062499938548711, 99.99999999999998579 ) ) ;
#17538=CARTESIAN_POINT ( 'NONE',  ( 82.39999999999999147, -34.41562499938547859, 103.1828516163667899 ) ) ;
#17541=CARTESIAN_POINT ( 'NONE',  ( -79.64356964375001269, -32.12812499938548427, 98.40857419181659793 ) ) ;
#17542=CARTESIAN_POINT ( 'NONE',  ( -82.39999999999999147, -30.25312499938548783, 96.81714838363319586 ) ) ;
#17543=ORIENTED_EDGE ( 'NONE', *, *, #2702, .T. ) ;
#17545=VECTOR ( 'NONE', #3989, 1000.000000000000000 ) ;
#17549=CARTESIAN_POINT ( 'NONE',  ( 82.40000000000000568, -32.08124999877097139, -102.9999999999999858 ) ) ;
#17554=CARTESIAN_POINT ( 'NONE',  ( 85.15643035624999868, -32.54062499938548569, 101.5914258081833879 ) ) ;
#17556=EDGE_CURVE ( 'NONE', #14982, #18033, #7505, .T. ) ;
#17557=CARTESIAN_POINT ( 'NONE',  ( -85.40000000000000568, -32.64374999877097139, -99.99999999999998579 ) ) ;
#17558=CARTESIAN_POINT ( 'NONE',  ( 83.77821517812500929, -34.22812499938549280, -102.3871387122750889 ) ) ;
#17563=CARTESIAN_POINT ( 'NONE',  ( 85.40000000000000568, -33.58124999877097139, 101.7320508075688679 ) ) ;
#17565=CARTESIAN_POINT ( 'NONE',  ( 85.40000000000000568, -32.60624999877096997, 98.26794919243111792 ) ) ;
#17569=CARTESIAN_POINT ( 'NONE',  ( -85.15643035625001289, -34.64062499938548711, -99.99999999999998579 ) ) ;
#17570=CARTESIAN_POINT ( 'NONE',  ( 82.40000000000000568, -30.00000000000000355, 96.99999999999998579 ) ) ;
#17573=CARTESIAN_POINT ( 'NONE',  ( 79.77811200999867935, -34.99999999999999289, 99.14934632385235602 ) ) ;
#17574=CARTESIAN_POINT ( 'NONE',  ( -85.15643035624999868, -30.74062499938548143, -101.5914258081833879 ) ) ;
#17575=CARTESIAN_POINT ( 'NONE',  ( -79.39999999999999147, -30.65624999877096712, -98.26794919243113213 ) ) ;
#17576=CARTESIAN_POINT ( 'NONE',  ( 79.77811200999867935, -34.99999999999999289, 99.14934632385235602 ) ) ;
#17581=CARTESIAN_POINT ( 'NONE',  ( 80.90000000000000568, -31.14374999877097139, -102.5980762113533018 ) ) ;
#17584=CARTESIAN_POINT ( 'NONE',  ( 79.64356964374998427, -34.37812499938548427, -98.40857419181659793 ) ) ;
#17590=ORIENTED_EDGE ( 'NONE', *, *, #15435, .T. ) ;
#17591=CARTESIAN_POINT ( 'NONE',  ( -82.40000000000001990, -32.13750000000000284, 103.0000000000000000 ) ) ;
#17593=ORIENTED_EDGE ( 'NONE', *, *, #13422, .F. ) ;
#17595=CARTESIAN_POINT ( 'NONE',  ( 82.39999999999999147, -31.91250000000000497, -96.53589838486223584 ) ) ;
#17598=CARTESIAN_POINT ( 'NONE',  ( -82.39999999999999147, -32.39062499938548001, 103.1828516163667899 ) ) ;
#17603=CARTESIAN_POINT ( 'NONE',  ( 81.48596794228855344, -35.00000000000000000, 102.8136019330778907 ) ) ;
#17606=VERTEX_POINT ( 'NONE', #2916 ) ;
#17607=CARTESIAN_POINT ( 'NONE',  ( -79.64356964375001269, -35.01562499938548711, -98.40857419181659793 ) ) ;
#17612=CARTESIAN_POINT ( 'NONE',  ( 82.39999999999999147, -32.81250000000000000, -97.00000000000000000 ) ) ;
#17621=CARTESIAN_POINT ( 'NONE',  ( 82.39999999999999147, -30.78750000000000497, 96.53589838486223584 ) ) ;
#17622=FACE_OUTER_BOUND ( 'NONE', #8470, .T. ) ;
#17624=( BOUNDED_CURVE ( )  B_SPLINE_CURVE ( 2, ( #15793, #8074, #18631, #2399, #6613, #12563, #5251, #11197, #11390 ),
 .UNSPECIFIED., .F., .F. ) 
 B_SPLINE_CURVE_WITH_KNOTS ( ( 3, 2, 2, 2, 3 ),
 ( 0.5208333333333333703, 0.5277777777777777901, 0.5416666666666666297, 0.5555555555555555802, 0.5625000000000000000 ),
 .UNSPECIFIED. ) 
 CURVE ( )  GEOMETRIC_REPRESENTATION_ITEM ( )  RATIONAL_B_SPLINE_CURVE ( ( 0.9330127018922192983, 0.9330127018922198534, 1.000000000000000000, 0.8660254037844387076, 1.000000000000000000, 0.8660254037844387076, 1.000000000000000000, 0.9330127018922194093, 0.9330127018922194093 ) ) 
 REPRESENTATION_ITEM ( '' )  );
#17626=LINE ( 'NONE', #1762, #5222 ) ;
#17627=CARTESIAN_POINT ( 'NONE',  ( 82.39999999999999147, -33.85312499938547859, 103.1828516163667899 ) ) ;
#17628=CARTESIAN_POINT ( 'NONE',  ( 79.64356964375001269, -31.30312499938548854, -101.5914258081833879 ) ) ;
#17629=ADVANCED_FACE ( 'NONE', ( #13462 ), #13370, .T. ) ;
#17631=CARTESIAN_POINT ( 'NONE',  ( -85.15643035625001289, -34.22812499938548569, 98.40857419181659793 ) ) ;
#17632=CARTESIAN_POINT ( 'NONE',  ( 81.02178482187500208, -30.44062499938548783, -102.3871387122750889 ) ) ;
#17633=B_SPLINE_CURVE_WITH_KNOTS ( 'NONE', 3,
 ( #1997, #12449, #6308, #5036, #6595, #14009, #16749, #18416, #13812, #12543, #1802, #6694, #453, #7954, #16947, #3367 ),
 .UNSPECIFIED., .F., .F.,
 ( 4, 2, 2, 2, 2, 2, 2, 4 ),
 ( 0.000000000000000000, 0.0005391024520904312426, 0.001078204904180862485, 0.002156409808361685505, 0.002695512260452097124, 0.003234614712542508742, 0.003773717164632920361, 0.004312819616723331979 ),
 .UNSPECIFIED. ) ;
#17635=CARTESIAN_POINT ( 'NONE',  ( 81.02178482187500208, -34.15312499938548285, 97.61286128772489690 ) ) ;
#17638=CARTESIAN_POINT ( 'NONE',  ( -85.15643035624999868, -34.22812499938547859, 98.40857419181659793 ) ) ;
#17640=CARTESIAN_POINT ( 'NONE',  ( -82.40000000000000568, -34.10624999877096997, 96.99999999999998579 ) ) ;
#17641=B_SPLINE_CURVE_WITH_KNOTS ( 'NONE', 3,
 ( #17235, #18512, #10883, #8049, #3745, #5330, #13905, #16852, #9711, #3557, #11174, #3456, #14005, #15580, #14196, #9619 ),
 .UNSPECIFIED., .F., .F.,
 ( 4, 2, 2, 2, 2, 2, 2, 4 ),
 ( 0.000000000000000000, 0.0005391024520904608413, 0.001078204904180921683, 0.002156409808361816477, 0.002695512260452254550, 0.003234614712542692189, 0.003773717164633130262, 0.004312819616723567902 ),
 .UNSPECIFIED. ) ;
#17642=AXIS2_PLACEMENT_3D ( 'NONE', #7118, #13453, #11604 ) ;
#17646=EDGE_CURVE ( 'NONE', #3049, #10326, #13451, .T. ) ;
#17648=CARTESIAN_POINT ( 'NONE',  ( -79.39999999999999147, -32.45624999877097139, 101.7320508075688537 ) ) ;
#17651=CARTESIAN_POINT ( 'NONE',  ( 79.64356964375001269, -32.76562499938548711, 98.40857419181659793 ) ) ;
#17653=CARTESIAN_POINT ( 'NONE',  ( -80.90000000000000568, -32.40000000000000568, -102.5980762113533018 ) ) ;
#17654=CARTESIAN_POINT ( 'NONE',  ( 81.02178482187500208, -33.55312499938548854, -97.61286128772489690 ) ) ;
#17655=CARTESIAN_POINT ( 'NONE',  ( -79.64356964374999848, -30.92812499938548498, -99.99999999999998579 ) ) ;
#17658=CARTESIAN_POINT ( 'NONE',  ( 80.90000000000000568, -33.84374999877096712, 97.40192378864668399 ) ) ;
#17662=CARTESIAN_POINT ( 'NONE',  ( -85.23110191009446623, -35.00000000000000000, -100.8575180188184675 ) ) ;
#17663=VERTEX_POINT ( 'NONE', #8966 ) ;
#17664=CARTESIAN_POINT ( 'NONE',  ( -85.15643035625001289, -35.09062499938548285, -99.99999999999998579 ) ) ;
#17667=CYLINDRICAL_SURFACE ( 'NONE', #17642, 3.000000000000002665 ) ;
#17668=CARTESIAN_POINT ( 'NONE',  ( -80.90000000000000568, -35.04374999877096997, -102.5980762113533018 ) ) ;
#17669=CARTESIAN_POINT ( 'NONE',  ( -82.61711639270095020, -32.00000000000000000, -102.8399189874719042 ) ) ;
#17670=CARTESIAN_POINT ( 'NONE',  ( -79.39999999999999147, -31.06874999877096855, -99.99999999999998579 ) ) ;
#17674=CARTESIAN_POINT ( 'NONE',  ( -79.64356964374999848, -34.86562499938548143, -99.99999999999998579 ) ) ;
#17675=CARTESIAN_POINT ( 'NONE',  ( 94.79999999999995453, -5.200000000000000178, 150.0000000000000000 ) ) ;
#17677=CARTESIAN_POINT ( 'NONE',  ( 79.39999999999999147, -30.65624999877096712, -101.7320508075688537 ) ) ;
#17688=CARTESIAN_POINT ( 'NONE',  ( 81.59615242270665192, -34.18259618943233136, -97.00000000000000000 ) ) ;
#17689=CARTESIAN_POINT ( 'NONE',  ( 99.99999999999997158, -5.200000000000008171, 150.0000000000000000 ) ) ;
#17691=EDGE_LOOP ( 'NONE', ( #10289, #16318, #1676, #18286 ) ) ;
#17693=CARTESIAN_POINT ( 'NONE',  ( 85.40000000000000568, -34.91250000000000142, -101.7320508075688679 ) ) ;
#17695=CARTESIAN_POINT ( 'NONE',  ( 80.90000000000000568, -35.04374999877096997, 102.5980762113533018 ) ) ;
#17696=CARTESIAN_POINT ( 'NONE',  ( -85.15643035625001289, -33.85312499938549280, 99.99999999999998579 ) ) ;
#17698=AXIS2_PLACEMENT_3D ( 'NONE', #8110, #18379, #792 ) ;
#17700=CARTESIAN_POINT ( 'NONE',  ( 81.70916641599873742, -34.99999999999999289, 102.8868501612598862 ) ) ;
#17701=CARTESIAN_POINT ( 'NONE',  ( 83.20395887649176814, -35.00000000000001421, 97.36341917746361219 ) ) ;
#17702=CARTESIAN_POINT ( 'NONE',  ( -83.90000000000000568, -34.51874999877097139, -102.5980762113533018 ) ) ;
#17703=ORIENTED_EDGE ( 'NONE', *, *, #17168, .F. ) ;
#17706=CARTESIAN_POINT ( 'NONE',  ( -83.77821517812500929, -30.21562499938548285, -102.3871387122750889 ) ) ;
#17710=CARTESIAN_POINT ( 'NONE',  ( -85.40000000000000568, -34.95000000000000284, -99.99999999999998579 ) ) ;
#17712=CARTESIAN_POINT ( 'NONE',  ( 80.90000000000000568, -33.30000000000000426, 102.5980762113533018 ) ) ;
#17715=ADVANCED_FACE ( 'NONE', ( #16113 ), #1268, .F. ) ;
#17718=EDGE_LOOP ( 'NONE', ( #15292, #14748, #8219, #17501 ) ) ;
#17722=CARTESIAN_POINT ( 'NONE',  ( 83.90000000000000568, -32.11874999877097281, -102.5980762113533018 ) ) ;
#17723=CARTESIAN_POINT ( 'NONE',  ( 83.77821517812500929, -34.11562499938548854, 97.61286128772489690 ) ) ;
#17730=CARTESIAN_POINT ( 'NONE',  ( 85.15643035624999868, -34.22812499938547859, 101.5914258081833879 ) ) ;
#17732=EDGE_CURVE ( 'NONE', #10833, #11539, #11965, .T. ) ;
#17733=CARTESIAN_POINT ( 'NONE',  ( 81.02178482187500208, -30.44062499938548783, -102.3871387122750889 ) ) ;
#17735=EDGE_CURVE ( 'NONE', #11141, #15349, #15334, .T. ) ;
#17736=CARTESIAN_POINT ( 'NONE',  ( 81.59615242270662350, -34.12634618820329990, 102.9999999999999858 ) ) ;
#17737=CARTESIAN_POINT ( 'NONE',  ( 81.02178482187500208, -32.69062499938548427, -102.3871387122750889 ) ) ;
#17738=ORIENTED_EDGE ( 'NONE', *, *, #15919, .F. ) ;
#17742=DIRECTION ( 'NONE',  ( -1.000000000000000000, 4.625929269271494788E-16, 0.000000000000000000 ) ) ;
#17743=CARTESIAN_POINT ( 'NONE',  ( -83.77821517812500929, -33.81562499938548427, 97.61286128772489690 ) ) ;
#17744=EDGE_LOOP ( 'NONE', ( #16206, #9365, #14742, #14624 ) ) ;
#17745=CARTESIAN_POINT ( 'NONE',  ( -84.59935209580208948, -35.00000000000002132, 101.7928000422517272 ) ) ;
#17747=( BOUNDED_CURVE ( )  B_SPLINE_CURVE ( 2, ( #15992, #14415, #11303, #14225, #18741, #864, #6827, #16089, #8275 ),
 .UNSPECIFIED., .F., .F. ) 
 B_SPLINE_CURVE_WITH_KNOTS ( ( 3, 2, 2, 2, 3 ),
 ( 0.4791666666666666297, 0.4861111111111111049, 0.5000000000000000000, 0.5138888888888888395, 0.5208333333333333703 ),
 .UNSPECIFIED. ) 
 CURVE ( )  GEOMETRIC_REPRESENTATION_ITEM ( )  RATIONAL_B_SPLINE_CURVE ( ( 0.9330127018922194093, 0.9330127018922190762, 1.000000000000000000, 0.8660254037844387076, 1.000000000000000000, 0.8660254037844387076, 1.000000000000000000, 0.9330127018922187432, 0.9330127018922192983 ) ) 
 REPRESENTATION_ITEM ( '' )  );
#17755=CARTESIAN_POINT ( 'NONE',  ( 83.77821517812500929, -31.97812499938548925, 97.61286128772489690 ) ) ;
#17756=CYLINDRICAL_SURFACE ( 'NONE', #18012, 2.649999999999985700 ) ;
#17757=CARTESIAN_POINT ( 'NONE',  ( -83.77821517812500929, -32.12812499938548427, 97.61286128772489690 ) ) ;
#17758=CARTESIAN_POINT ( 'NONE',  ( -82.39999999999999147, -30.81562499938548427, -103.1828516163667899 ) ) ;
#17760=CARTESIAN_POINT ( 'NONE',  ( 85.40000000000000568, -33.54374999877096286, 99.99999999999998579 ) ) ;
#17761=FACE_OUTER_BOUND ( 'NONE', #17297, .T. ) ;
#17763=CARTESIAN_POINT ( 'NONE',  ( -85.15643035625001289, -30.70312499938548711, 99.99999999999998579 ) ) ;
#17765=ORIENTED_EDGE ( 'NONE', *, *, #6731, .F. ) ;
#17766=CARTESIAN_POINT ( 'NONE',  ( -79.64356964374999848, -34.86562499938548143, -99.99999999999998579 ) ) ;
#17768=VERTEX_POINT ( 'NONE', #13838 ) ;
#17771=CARTESIAN_POINT ( 'NONE',  ( -81.02178482187500208, -33.10312499938548569, -102.3871387122750889 ) ) ;
#17772=CARTESIAN_POINT ( 'NONE',  ( -79.79868554276779946, -32.00000000000000711, -101.4716133421136846 ) ) ;
#17773=CARTESIAN_POINT ( 'NONE',  ( -79.39999999999999147, -32.45624999877097139, -98.26794919243113213 ) ) ;
#17777=CARTESIAN_POINT ( 'NONE',  ( -81.02178482187500208, -34.04062499938548569, -97.61286128772489690 ) ) ;
#17779=DIRECTION ( 'NONE',  ( 0.000000000000000000, 0.000000000000000000, -1.000000000000000000 ) ) ;
#17780=CARTESIAN_POINT ( 'NONE',  ( 79.39999999999999147, -32.38124999877096855, -98.26794919243110371 ) ) ;
#17790=CARTESIAN_POINT ( 'NONE',  ( 79.39999999999999147, -34.31250000000000000, -101.7320508075688537 ) ) ;
#17792=CARTESIAN_POINT ( 'NONE',  ( -82.40000000000000568, -32.30624999877097281, 97.00000000000000000 ) ) ;
#17794=CARTESIAN_POINT ( 'NONE',  ( -79.83361526238435601, -35.00000000000000711, 101.0217260113603572 ) ) ;
#17795=CARTESIAN_POINT ( 'NONE',  ( -83.77821517812500929, -33.02812499938548285, 97.61286128772489690 ) ) ;
#17799=CARTESIAN_POINT ( 'NONE',  ( -82.41196654184768988, -35.00000000000000711, -102.9991646027828693 ) ) ;
#17801=ORIENTED_EDGE ( 'NONE', *, *, #17357, .F. ) ;
#17802=ADVANCED_FACE ( 'NONE', ( #2021 ), #6431, .T. ) ;
#17804=CARTESIAN_POINT ( 'NONE',  ( -83.77821517812500929, -31.11562499938548498, -102.3871387122750889 ) ) ;
#17805=CARTESIAN_POINT ( 'NONE',  ( -83.20384757729337366, -33.50759618943233420, 103.0000000000000000 ) ) ;
#17807=LINE ( 'NONE', #12031, #7102 ) ;
#17809=CARTESIAN_POINT ( 'NONE',  ( 82.39999999999999147, -34.33124999877097139, 97.00000000000000000 ) ) ;
#17811=EDGE_LOOP ( 'NONE', ( #4254, #15840, #5024, #1085 ) ) ;
#17812=ORIENTED_EDGE ( 'NONE', *, *, #4882, .F. ) ;
#17815=CARTESIAN_POINT ( 'NONE',  ( -79.39999999999999147, -32.38124999877096855, 98.26794919243110371 ) ) ;
#17816=CARTESIAN_POINT ( 'NONE',  ( 83.90000000000000568, -33.07500000000000284, 97.40192378864668399 ) ) ;
#17817=CARTESIAN_POINT ( 'NONE',  ( -82.86160995759659897, -32.00000000000002132, -97.18959324165045643 ) ) ;
#17819=CARTESIAN_POINT ( 'NONE',  ( 85.40000000000000568, -32.15624999877096712, 98.26794919243111792 ) ) ;
#17820=CARTESIAN_POINT ( 'NONE',  ( 79.64356964375001269, -33.47812499938547859, 101.5914258081833879 ) ) ;
#17822=CARTESIAN_POINT ( 'NONE',  ( 79.64356964375001269, -30.40312499938548285, -101.5914258081833879 ) ) ;
#17824=CARTESIAN_POINT ( 'NONE',  ( -82.39999999999999147, -34.75312499938548427, 96.81714838363319586 ) ) ;
#17825=CARTESIAN_POINT ( 'NONE',  ( 82.39999999999999147, -34.07812499938548711, -103.1828516163667899 ) ) ;
#17830=CARTESIAN_POINT ( 'NONE',  ( -83.90000000000000568, -31.42500000000000071, 97.40192378864668399 ) ) ;
#17832=CARTESIAN_POINT ( 'NONE',  ( -69.99999999999998579, -35.00000000000000000, 150.0000000000000000 ) ) ;
#17835=CARTESIAN_POINT ( 'NONE',  ( -82.39999999999999147, -34.33124999877097139, -97.00000000000000000 ) ) ;
#17841=CARTESIAN_POINT ( 'NONE',  ( 83.77821517812500929, -31.67812499938548498, 102.3871387122750889 ) ) ;
#17842=EDGE_CURVE ( 'NONE', #13089, #893, #11005, .T. ) ;
#17845=B_SPLINE_CURVE_WITH_KNOTS ( 'NONE', 3,
 ( #17095, #2047, #14156, #8006, #8207, #15536, #4997, #790, #411, #2152, #12692, #3707, #8109, #9673, #3419, #9371, #11229, #18666 ),
 .UNSPECIFIED., .F., .F.,
 ( 4, 2, 2, 2, 2, 2, 2, 2, 4 ),
 ( 0.000000000000000000, 0.0007089252359871620014, 0.001417850471974324003, 0.002126775707961485896, 0.002835700943948648006, 0.003544626179935810115, 0.004253551415922971791, 0.004962476651910133901, 0.005671401887897296011 ),
 .UNSPECIFIED. ) ;
#17846=CARTESIAN_POINT ( 'NONE',  ( 84.51155386534844638, -35.25364837475780888, -98.22820752270799005 ) ) ;
#17847=CARTESIAN_POINT ( 'NONE',  ( -85.15643035624999868, -32.01562499938548711, -98.40857419181659793 ) ) ;
#17849=CARTESIAN_POINT ( 'NONE',  ( 79.64356964374999848, -30.92812499938548498, 99.99999999999998579 ) ) ;
#17850=CARTESIAN_POINT ( 'NONE',  ( 83.90000000000000568, -34.36874999877097281, 97.40192378864668399 ) ) ;
#17855=CARTESIAN_POINT ( 'NONE',  ( -79.64356964375001269, -32.24062499938548854, 98.40857419181659793 ) ) ;
#17856=CYLINDRICAL_SURFACE ( 'NONE', #9618, 3.000000000000002665 ) ;
#17858=CARTESIAN_POINT ( 'NONE',  ( -79.64356964375001269, -33.55312499938548854, -98.40857419181659793 ) ) ;
#17859=CARTESIAN_POINT ( 'NONE',  ( 80.90000000000000568, -32.49374999877097281, 97.40192378864668399 ) ) ;
#17860=ADVANCED_FACE ( 'NONE', ( #3585 ), #6242, .T. ) ;
#17862=CARTESIAN_POINT ( 'NONE',  ( -83.77821517812500929, -33.92812499938548854, -102.3871387122750889 ) ) ;
#17864=CARTESIAN_POINT ( 'NONE',  ( -85.40000000000000568, -31.74374999877096926, -99.99999999999998579 ) ) ;
#17868=DIRECTION ( 'NONE',  ( -0.000000000000000000, -1.000000000000000000, -0.000000000000000000 ) ) ;
#17869=CARTESIAN_POINT ( 'NONE',  ( 85.15643035625001289, -33.32812499938548711, 101.5914258081833879 ) ) ;
#17870=CARTESIAN_POINT ( 'NONE',  ( 79.39999999999999147, -32.51250000000000284, -101.7320508075688537 ) ) ;
#17874=CARTESIAN_POINT ( 'NONE',  ( 83.90000000000000568, -34.81874999877096855, -102.5980762113533018 ) ) ;
#17884=VERTEX_POINT ( 'NONE', #16593 ) ;
#17885=CARTESIAN_POINT ( 'NONE',  ( -80.90000000000000568, -32.10000000000000142, 102.5980762113533018 ) ) ;
#17886=AXIS2_PLACEMENT_3D ( 'NONE', #16918, #15449, #3233 ) ;
#17888=DIRECTION ( 'NONE',  ( -0.000000000000000000, -1.000000000000000000, -0.000000000000000000 ) ) ;
#17891=DIRECTION ( 'NONE',  ( 4.625929269271494788E-16, 1.000000000000000000, -0.000000000000000000 ) ) ;
#17892=CARTESIAN_POINT ( 'NONE',  ( -81.02178482187500208, -35.05312499938548854, 102.3871387122750889 ) ) ;
#17898=DIRECTION ( 'NONE',  ( -0.000000000000000000, -1.000000000000000000, -0.000000000000000000 ) ) ;
#17900=ORIENTED_EDGE ( 'NONE', *, *, #15807, .F. ) ;
#17902=CARTESIAN_POINT ( 'NONE',  ( -79.64356964375001269, -32.12812499938548427, -101.5914258081833879 ) ) ;
#17905=( BOUNDED_CURVE ( )  B_SPLINE_CURVE ( 2, ( #7902, #4989, #6162, #9268, #6258, #10832, #16802, #15235, #3412 ),
 .UNSPECIFIED., .F., .F. ) 
 B_SPLINE_CURVE_WITH_KNOTS ( ( 3, 2, 2, 2, 3 ),
 ( 0.7291666666666668517, 0.7361111111111111605, 0.7500000000000000000, 0.7638888888888888395, 0.7708333333333332593 ),
 .UNSPECIFIED. ) 
 CURVE ( )  GEOMETRIC_REPRESENTATION_ITEM ( )  RATIONAL_B_SPLINE_CURVE ( ( 0.9330127018922194093, 0.9330127018922209636, 1.000000000000000000, 0.8660254037844387076, 1.000000000000000000, 0.8660254037844387076, 1.000000000000000000, 0.9330127018922198534, 0.9330127018922192983 ) ) 
 REPRESENTATION_ITEM ( '' )  );
#17906=CARTESIAN_POINT ( 'NONE',  ( 80.17984880387895430, -35.00000000000000000, -101.6434491389460817 ) ) ;
#17911=ORIENTED_EDGE ( 'NONE', *, *, #15817, .F. ) ;
#17914=CARTESIAN_POINT ( 'NONE',  ( -85.40000000000000568, -32.68124999877097281, 98.26794919243111792 ) ) ;
#17915=CARTESIAN_POINT ( 'NONE',  ( 83.90000000000000568, -31.27500000000000568, 97.40192378864668399 ) ) ;
#17916=CARTESIAN_POINT ( 'NONE',  ( 82.40000000000001990, -32.53124999877097423, 97.00000000000000000 ) ) ;
#17919=CARTESIAN_POINT ( 'NONE',  ( 82.39999999999999147, -34.07812499938548711, 96.81714838363319586 ) ) ;
#17920=CARTESIAN_POINT ( 'NONE',  ( 79.64356964375001269, -32.20312499938548001, -101.5914258081833879 ) ) ;
#17923=CARTESIAN_POINT ( 'NONE',  ( 81.59615242270662350, -34.31115380933863435, 96.99999999999998579 ) ) ;
#17924=CARTESIAN_POINT ( 'NONE',  ( 85.15643035624999868, -32.87812499938549138, -98.40857419181659793 ) ) ;
#17925=DIRECTION ( 'NONE',  ( -1.000000000000000000, 0.000000000000000000, 0.000000000000000000 ) ) ;
#17928=CARTESIAN_POINT ( 'NONE',  ( -85.40000000000000568, -30.86250000000000071, 101.7320508075688679 ) ) ;
#17932=CARTESIAN_POINT ( 'NONE',  ( -79.39999999999999147, -34.27499999999999858, 99.99999999999998579 ) ) ;
#17933=CARTESIAN_POINT ( 'NONE',  ( 85.15643035624999868, -30.62812499938548427, 101.5914258081833879 ) ) ;
#17936=CARTESIAN_POINT ( 'NONE',  ( -82.40000000000000568, -32.08124999877097139, 102.9999999999999858 ) ) ;
#17939=CARTESIAN_POINT ( 'NONE',  ( 81.02178482187500208, -33.10312499938548569, 102.3871387122750889 ) ) ;
#17940=CARTESIAN_POINT ( 'NONE',  ( 82.39999999999999147, -30.36562499938549209, -96.81714838363319586 ) ) ;
#17942=CARTESIAN_POINT ( 'NONE',  ( 85.15643035625001289, -35.22676544108147567, -98.99674642581742035 ) ) ;
#17943=CARTESIAN_POINT ( 'NONE',  ( -81.02178482187500208, -31.45312499938549067, -97.61286128772489690 ) ) ;
#17945=CARTESIAN_POINT ( 'NONE',  ( 79.64356964375001269, -30.44062499938548783, 101.5914258081833879 ) ) ;
#17946=DIRECTION ( 'NONE',  ( -0.000000000000000000, -0.000000000000000000, -1.000000000000000000 ) ) ;
#17947=CARTESIAN_POINT ( 'NONE',  ( 83.20384757729337366, -32.55134618820330417, 97.00000000000000000 ) ) ;
#17949=VECTOR ( 'NONE', #9643, 1000.000000000000000 ) ;
#17951=CARTESIAN_POINT ( 'NONE',  ( -83.77821517812500929, -32.42812499938548854, 102.3871387122750889 ) ) ;
#17954=CARTESIAN_POINT ( 'NONE',  ( -82.39999999999999147, -31.68750000000000355, -96.53589838486223584 ) ) ;
#17957=CARTESIAN_POINT ( 'NONE',  ( -85.40000000000000568, -34.93124999877096570, -101.7320508075688821 ) ) ;
#17958=CARTESIAN_POINT ( 'NONE',  ( -85.15643035624999868, -32.91562499938549280, -98.40857419181659793 ) ) ;
#17963=CARTESIAN_POINT ( 'NONE',  ( -81.02178482187500208, -34.49062499938548854, -97.61286128772489690 ) ) ;
#17964=CARTESIAN_POINT ( 'NONE',  ( 83.77821517812500929, -33.81562499938548427, 102.3871387122750889 ) ) ;
#17966=AXIS2_PLACEMENT_3D ( 'NONE', #8746, #10406, #12065 ) ;
#17967=DIRECTION ( 'NONE',  ( -1.000000000000000000, 1.586032892321652285E-15, -0.000000000000000000 ) ) ;
#17968=CARTESIAN_POINT ( 'NONE',  ( 83.90000000000000568, -34.36874999877097281, -102.5980762113533018 ) ) ;
#17970=( BOUNDED_CURVE ( )  B_SPLINE_CURVE ( 2, ( #17195, #606, #12312, #15437, #6652, #12598, #18567, #3610, #6555 ),
 .UNSPECIFIED., .F., .F. ) 
 B_SPLINE_CURVE_WITH_KNOTS ( ( 3, 2, 2, 2, 3 ),
 ( 0.6875000000000000000, 0.6944444444444444198, 0.7083333333333333703, 0.7222222222222222099, 0.7291666666666666297 ),
 .UNSPECIFIED. ) 
 CURVE ( )  GEOMETRIC_REPRESENTATION_ITEM ( )  RATIONAL_B_SPLINE_CURVE ( ( 0.9330127018922194093, 0.9330127018922194093, 1.000000000000000000, 0.8660254037844387076, 1.000000000000000000, 0.8660254037844387076, 1.000000000000000000, 0.9330127018922198534, 0.9330127018922192983 ) ) 
 REPRESENTATION_ITEM ( '' )  );
#17971=EDGE_CURVE ( 'NONE', #8657, #12671, #17456, .T. ) ;
#17977=EDGE_CURVE ( 'NONE', #11363, #9248, #5550, .T. ) ;
#17979=ORIENTED_EDGE ( 'NONE', *, *, #1374, .F. ) ;
#17980=ORIENTED_EDGE ( 'NONE', *, *, #10096, .F. ) ;
#17987=CARTESIAN_POINT ( 'NONE',  ( -82.39999999999999147, -33.20624999877097849, -103.0000000000000000 ) ) ;
#17988=CARTESIAN_POINT ( 'NONE',  ( -81.02178482187500208, -34.60312499938549280, 102.3871387122750889 ) ) ;
#17994=CYLINDRICAL_SURFACE ( 'NONE', #12115, 3.000000000000002665 ) ;
#17995=CARTESIAN_POINT ( 'NONE',  ( -82.40000000000000568, -30.00000000000000355, 99.99999999999998579 ) ) ;
#17996=VECTOR ( 'NONE', #8956, 1000.000000000000000 ) ;
#17997=CARTESIAN_POINT ( 'NONE',  ( -85.40000000000000568, -34.44374999877096855, -99.99999999999998579 ) ) ;
#17998=EDGE_LOOP ( 'NONE', ( #13969, #13850, #13918, #18572 ) ) ;
#18000=CARTESIAN_POINT ( 'NONE',  ( -79.64356964375001269, -33.92812499938548854, -101.5914258081833879 ) ) ;
#18004=CARTESIAN_POINT ( 'NONE',  ( -82.40000000000000568, -33.43124999877096570, 102.9999999999999858 ) ) ;
#18007=ORIENTED_EDGE ( 'NONE', *, *, #3556, .T. ) ;
#18009=VERTEX_POINT ( 'NONE', #18540 ) ;
#18010=CARTESIAN_POINT ( 'NONE',  ( -85.40000000000000568, -34.91250000000000142, -98.26794919243111792 ) ) ;
#18012=AXIS2_PLACEMENT_3D ( 'NONE', #8751, #14703, #10224 ) ;
#18013=CARTESIAN_POINT ( 'NONE',  ( -85.40000000000000568, -33.05624999877096570, 101.7320508075688679 ) ) ;
#18014=CARTESIAN_POINT ( 'NONE',  ( 85.40000000000000568, -32.21249999999999858, 98.26794919243111792 ) ) ;
#18022=CARTESIAN_POINT ( 'NONE',  ( 85.15643035624999868, -30.17812499938548498, -98.40857419181659793 ) ) ;
#18026=CARTESIAN_POINT ( 'NONE',  ( -82.40000000000000568, -33.93750000000000711, 102.9999999999999858 ) ) ;
#18027=CARTESIAN_POINT ( 'NONE',  ( 79.64356964375001269, -34.45312499938548711, -101.5914258081833879 ) ) ;
#18028=AXIS2_PLACEMENT_3D ( 'NONE', #7054, #14281, #821 ) ;
#18030=CARTESIAN_POINT ( 'NONE',  ( 81.59615242270662350, -33.73259618943233562, -96.99999999999998579 ) ) ;
#18032=CARTESIAN_POINT ( 'NONE',  ( -79.39999999999999147, -31.61250000000000071, 101.7320508075688537 ) ) ;
#18033=VERTEX_POINT ( 'NONE', #2501 ) ;
#18034=CARTESIAN_POINT ( 'NONE',  ( -85.32499745258149915, -34.99999999999999289, 99.84129707247753061 ) ) ;
#18036=CARTESIAN_POINT ( 'NONE',  ( -82.40000000000000568, -34.38749999999999574, 102.9999999999999858 ) ) ;
#18037=CARTESIAN_POINT ( 'NONE',  ( 81.02178482187500208, -30.89062499938548711, 97.61286128772489690 ) ) ;
#18039=VECTOR ( 'NONE', #7724, 1000.000000000000000 ) ;
#18044=CARTESIAN_POINT ( 'NONE',  ( 85.15643035625001289, -30.59062499938548285, 99.99999999999998579 ) ) ;
#18045=CARTESIAN_POINT ( 'NONE',  ( 85.15643035624999868, -30.29062499938548925, -98.40857419181659793 ) ) ;
#18046=AXIS2_PLACEMENT_3D ( 'NONE', #14116, #18627, #12946 ) ;
#18048=CARTESIAN_POINT ( 'NONE',  ( -84.53225329756183726, -32.00000000000000000, -101.7559005160110956 ) ) ;
#18049=CARTESIAN_POINT ( 'NONE',  ( -83.77821517812500929, -31.07812499938548711, -97.61286128772489690 ) ) ;
#18051=CARTESIAN_POINT ( 'NONE',  ( 81.02178482187500208, -31.45312499938549067, 97.61286128772489690 ) ) ;
#18053=VECTOR ( 'NONE', #5410, 1000.000000000000000 ) ;
#18055=CARTESIAN_POINT ( 'NONE',  ( -81.02178482187500208, -30.85312499938548569, 97.61286128772489690 ) ) ;
#18056=( BOUNDED_CURVE ( )  B_SPLINE_CURVE ( 2, ( #6503, #18226, #12638, #5131, #18514, #11076, #5229 ),
 .UNSPECIFIED., .F., .T. ) 
 B_SPLINE_CURVE_WITH_KNOTS ( ( 3, 2, 2, 3 ),
 ( 0.3702305174531529408, 0.3750000000000000000, 0.3888888888888888951, 0.3958333333333334259 ),
 .UNSPECIFIED. ) 
 CURVE ( )  GEOMETRIC_REPRESENTATION_ITEM ( )  RATIONAL_B_SPLINE_CURVE ( ( 0.9395835397632826824, 0.9539927561172878434, 1.000000000000000000, 0.8660254037844387076, 1.000000000000000000, 0.9330127018922185211, 0.9330127018922192983 ) ) 
 REPRESENTATION_ITEM ( '' )  );
#18058=CARTESIAN_POINT ( 'NONE',  ( -85.40000000000000568, -32.21249999999999858, -98.26794919243111792 ) ) ;
#18060=CARTESIAN_POINT ( 'NONE',  ( -83.77821517812500929, -32.57812499938548711, -102.3871387122750889 ) ) ;
#18065=CYLINDRICAL_SURFACE ( 'NONE', #18822, 3.000000000000002665 ) ;
#18066=CARTESIAN_POINT ( 'NONE',  ( 79.64356964374998427, -33.55312499938548854, 98.40857419181659793 ) ) ;
#18069=CARTESIAN_POINT ( 'NONE',  ( 83.90000000000000568, -33.61874999877097281, -97.40192378864668399 ) ) ;
#18071=ADVANCED_FACE ( 'NONE', ( #15706 ), #5359, .T. ) ;
#18072=ADVANCED_FACE ( 'NONE', ( #3775 ), #15459, .F. ) ;
#18073=EDGE_LOOP ( 'NONE', ( #9487, #13952, #14075, #507 ) ) ;
#18080=ORIENTED_EDGE ( 'NONE', *, *, #13335, .F. ) ;
#18082=CARTESIAN_POINT ( 'NONE',  ( -99.99999999999998579, -32.00000000000000000, 150.0000000000000000 ) ) ;
#18087=EDGE_CURVE ( 'NONE', #10401, #4006, #11853, .T. ) ;
#18088=CARTESIAN_POINT ( 'NONE',  ( -82.39999999999999147, -34.19062499938548427, 103.1828516163667899 ) ) ;
#18093=CARTESIAN_POINT ( 'NONE',  ( -81.59615242270662350, -33.91740381056766296, 103.0000000000000000 ) ) ;
#18095=DIRECTION ( 'NONE',  ( -0.000000000000000000, -1.000000000000000000, -0.000000000000000000 ) ) ;
#18100=CARTESIAN_POINT ( 'NONE',  ( -82.39999999999999147, -33.62812499938549138, -96.81714838363319586 ) ) ;
#18103=CARTESIAN_POINT ( 'NONE',  ( 79.90595866893272614, -34.99999999999998579, -101.1871036926522578 ) ) ;
#18107=EDGE_LOOP ( 'NONE', ( #3597, #17210, #10069, #7826 ) ) ;
#18108=CARTESIAN_POINT ( 'NONE',  ( -99.99999999999998579, -32.00000000000000000, 150.0000000000000000 ) ) ;
#18110=CARTESIAN_POINT ( 'NONE',  ( -79.39999999999999147, -32.83124999877097139, 98.26794919243110371 ) ) ;
#18111=CARTESIAN_POINT ( 'NONE',  ( 83.90000000000000568, -32.62500000000000000, 97.40192378864668399 ) ) ;
#18112=CARTESIAN_POINT ( 'NONE',  ( 85.40000000000000568, -33.50624999877096855, 98.26794919243111792 ) ) ;
#18114=CARTESIAN_POINT ( 'NONE',  ( 81.02178482187500208, -33.70312499938548711, -102.3871387122750889 ) ) ;
#18116=CARTESIAN_POINT ( 'NONE',  ( 83.77821517812500929, -33.36562499938548854, -97.61286128772489690 ) ) ;
#18117=ORIENTED_EDGE ( 'NONE', *, *, #17971, .T. ) ;
#18119=CARTESIAN_POINT ( 'NONE',  ( -79.64356964374998427, -34.90312499938548285, 101.5914258081833879 ) ) ;
#18120=CARTESIAN_POINT ( 'NONE',  ( 79.64356964375001269, -34.00312499938549138, -101.5914258081833879 ) ) ;
#18125=CARTESIAN_POINT ( 'NONE',  ( -79.39999999999999147, -30.63750000000000284, 98.26794919243110371 ) ) ;
#18126=ORIENTED_EDGE ( 'NONE', *, *, #2537, .F. ) ;
#18133=CARTESIAN_POINT ( 'NONE',  ( 82.39999999999999147, -34.41562499938547859, 103.1828516163667899 ) ) ;
#18134=EDGE_CURVE ( 'NONE', #19014, #11146, #8482, .T. ) ;
#18135=CARTESIAN_POINT ( 'NONE',  ( 81.02178482187500208, -32.65312499938548996, -97.61286128772489690 ) ) ;
#18137=CARTESIAN_POINT ( 'NONE',  ( -85.15643035625001289, -32.50312499938548427, 99.99999999999998579 ) ) ;
#18138=CARTESIAN_POINT ( 'NONE',  ( -85.15643035624999868, -34.79062499938548569, -101.5914258081833879 ) ) ;
#18141=CARTESIAN_POINT ( 'NONE',  ( 81.02178482187500208, -30.55312499938548854, 97.61286128772489690 ) ) ;
#18142=CARTESIAN_POINT ( 'NONE',  ( 85.40000000000000568, -34.40624999877096712, 98.26794919243111792 ) ) ;
#18144=CARTESIAN_POINT ( 'NONE',  ( -79.64356964375001269, -30.51562499938548711, 101.5914258081833879 ) ) ;
#18147=CARTESIAN_POINT ( 'NONE',  ( -79.39999999999999147, -30.22500000000000142, -99.99999999999998579 ) ) ;
#18148=LINE ( 'NONE', #16771, #11612 ) ;
#18150=CARTESIAN_POINT ( 'NONE',  ( -85.15643035625001289, -34.30312499938548854, -99.99999999999998579 ) ) ;
#18154=ORIENTED_EDGE ( 'NONE', *, *, #13289, .T. ) ;
#18156=CARTESIAN_POINT ( 'NONE',  ( -82.39999999999999147, -33.65624999877097423, 97.00000000000000000 ) ) ;
#18157=CARTESIAN_POINT ( 'NONE',  ( 85.15643035625001289, -32.80312499938548854, 98.40857419181659793 ) ) ;
#18158=CARTESIAN_POINT ( 'NONE',  ( 83.90000000000000568, -34.51874999877097139, -97.40192378864668399 ) ) ;
#18159=CARTESIAN_POINT ( 'NONE',  ( -82.40000000000001990, -34.55624999877097281, 97.00000000000000000 ) ) ;
#18160=CARTESIAN_POINT ( 'NONE',  ( 80.90000000000000568, -33.84374999877096712, -102.5980762113533018 ) ) ;
#18161=CARTESIAN_POINT ( 'NONE',  ( 81.59615242270662350, -34.63259618943234130, 103.0000000000000000 ) ) ;
#18163=ORIENTED_EDGE ( 'NONE', *, *, #11869, .F. ) ;
#18168=CARTESIAN_POINT ( 'NONE',  ( -82.40000000000000568, -33.03750000000000142, -96.99999999999998579 ) ) ;
#18169=VERTEX_POINT ( 'NONE', #7937 ) ;
#18173=CARTESIAN_POINT ( 'NONE',  ( -81.59615242270662350, -34.63259618943234130, 96.99999999999997158 ) ) ;
#18176=CARTESIAN_POINT ( 'NONE',  ( -99.99999999999998579, -5.200000000000000178, 150.0000000000000000 ) ) ;
#18185=LINE ( 'NONE', #1673, #2130 ) ;
#18186=CARTESIAN_POINT ( 'NONE',  ( -79.39999999999999147, -34.63124999877096855, -101.7320508075688963 ) ) ;
#18190=CARTESIAN_POINT ( 'NONE',  ( -81.02178482187500208, -32.54062499938548569, -102.3871387122750889 ) ) ;
#18193=VECTOR ( 'NONE', #9443, 1000.000000000000000 ) ;
#18195=DIRECTION ( 'NONE',  ( 0.000000000000000000, -1.000000000000000000, 0.000000000000000000 ) ) ;
#18198=DIRECTION ( 'NONE',  ( 0.000000000000000000, 0.000000000000000000, -1.000000000000000000 ) ) ;
#18199=ORIENTED_EDGE ( 'NONE', *, *, #15488, .F. ) ;
#18201=CARTESIAN_POINT ( 'NONE',  ( -82.39076102795759482, -32.00000000000002132, 102.8695224571928719 ) ) ;
#18202=CARTESIAN_POINT ( 'NONE',  ( 85.15643035624999868, -35.11426541925033007, -98.99674735228809652 ) ) ;
#18203=EDGE_CURVE ( 'NONE', #8568, #1717, #7550, .T. ) ;
#18204=CARTESIAN_POINT ( 'NONE',  ( -79.39999999999999147, -31.51874999877096784, 99.99999999999998579 ) ) ;
#18205=CARTESIAN_POINT ( 'NONE',  ( 85.40000000000000568, -32.73750000000000426, 101.7320508075688679 ) ) ;
#18209=CARTESIAN_POINT ( 'NONE',  ( 85.15643035625001289, -33.81562499938548427, -101.5914258081833879 ) ) ;
#18210=CARTESIAN_POINT ( 'NONE',  ( 96.99999999999994316, -29.80000000000000426, 150.0000000000000000 ) ) ;
#18211=CARTESIAN_POINT ( 'NONE',  ( 85.15643035624999868, -33.77812499938548285, -98.40857419181659793 ) ) ;
#18214=CARTESIAN_POINT ( 'NONE',  ( 83.77821517812500929, -32.46562499938548285, -97.61286128772489690 ) ) ;
#18215=PLANE ( 'NONE',  #10835 ) ;
#18216=EDGE_CURVE ( 'NONE', #18536, #2292, #16484, .T. ) ;
#18220=EDGE_CURVE ( 'NONE', #867, #4201, #6013, .T. ) ;
#18221=CARTESIAN_POINT ( 'NONE',  ( -85.40000000000000568, -30.48749999999999716, 98.26794919243111792 ) ) ;
#18226=CARTESIAN_POINT ( 'NONE',  ( 79.40000000000000568, -32.01330983656912821, -99.46005447970492241 ) ) ;
#18229=CARTESIAN_POINT ( 'NONE',  ( 79.93183330737453218, -31.99999999999997158, 98.31447495408103521 ) ) ;
#18230=CARTESIAN_POINT ( 'NONE',  ( 81.02178482187500208, -34.45312499938548711, 102.3871387122750889 ) ) ;
#18231=CARTESIAN_POINT ( 'NONE',  ( 82.39999999999999147, -32.84062499938548996, -103.1828516163667899 ) ) ;
#18233=CARTESIAN_POINT ( 'NONE',  ( -85.15643035625001289, -33.81562499938548427, 101.5914258081833879 ) ) ;
#18234=CARTESIAN_POINT ( 'NONE',  ( -79.64356964374999848, -33.62812499938548427, -99.99999999999998579 ) ) ;
#18236=CARTESIAN_POINT ( 'NONE',  ( 79.64356964375001269, -30.51562499938548711, 98.40857419181659793 ) ) ;
#18239=CARTESIAN_POINT ( 'NONE',  ( -85.15643035624999868, -33.81562499938549138, 101.5914258081833879 ) ) ;
#18241=ORIENTED_EDGE ( 'NONE', *, *, #4863, .F. ) ;
#18243=CARTESIAN_POINT ( 'NONE',  ( -79.39999999999999147, -31.98750000000000071, -101.7320508075688821 ) ) ;
#18244=CARTESIAN_POINT ( 'NONE',  ( 84.12112955302457351, -35.00000000000000000, 102.4658001909610476 ) ) ;
#18246=CARTESIAN_POINT ( 'NONE',  ( -83.77821517812500929, -34.82812499938548711, -102.3871387122750889 ) ) ;
#18251=ADVANCED_FACE ( 'NONE', ( #3344 ), #14980, .F. ) ;
#18252=DIRECTION ( 'NONE',  ( 0.000000000000000000, -1.000000000000000000, 0.000000000000000000 ) ) ;
#18253=CARTESIAN_POINT ( 'NONE',  ( 83.90000000000000568, -32.32500000000000284, 102.5980762113533018 ) ) ;
#18254=CARTESIAN_POINT ( 'NONE',  ( 79.64356964374999848, -33.51562499938548711, 99.99999999999998579 ) ) ;
#18255=CARTESIAN_POINT ( 'NONE',  ( 81.59615242270662350, -34.36740381056766580, 96.99999999999998579 ) ) ;
#18258=CARTESIAN_POINT ( 'NONE',  ( 85.40000000000000568, -33.50624999877096855, -101.7320508075688679 ) ) ;
#18260=ORIENTED_EDGE ( 'NONE', *, *, #11635, .F. ) ;
#18265=CARTESIAN_POINT ( 'NONE',  ( -80.90000000000000568, -33.00000000000000000, -97.40192378864668399 ) ) ;
#18272=PLANE ( 'NONE',  #7645 ) ;
#18273=CARTESIAN_POINT ( 'NONE',  ( -85.40000000000000568, -33.95624999877097139, -98.26794919243111792 ) ) ;
#18278=LINE ( 'NONE', #5089, #6965 ) ;
#18284=VERTEX_POINT ( 'NONE', #7841 ) ;
#18285=CARTESIAN_POINT ( 'NONE',  ( -81.02178482187500208, -32.24062499938548854, -97.61286128772489690 ) ) ;
#18286=ORIENTED_EDGE ( 'NONE', *, *, #18668, .F. ) ;
#18295=CARTESIAN_POINT ( 'NONE',  ( 81.59615242270662350, -34.57634618820329564, 103.0000000000000000 ) ) ;
#18296=CARTESIAN_POINT ( 'NONE',  ( 85.15643035625001289, -34.64062499938548711, -99.99999999999998579 ) ) ;
#18298=CARTESIAN_POINT ( 'NONE',  ( -82.39999999999999147, -34.55624999877096570, 96.53589838486223584 ) ) ;
#18299=CARTESIAN_POINT ( 'NONE',  ( 82.40000000000001990, -32.13750000000000284, -103.0000000000000000 ) ) ;
#18300=CARTESIAN_POINT ( 'NONE',  ( 82.39999999999999147, -33.20624999877097849, 102.9999999999999858 ) ) ;
#18302=CARTESIAN_POINT ( 'NONE',  ( 83.77821517812500929, -33.92812499938548854, -97.61286128772489690 ) ) ;
#18303=CARTESIAN_POINT ( 'NONE',  ( 82.40000000000001990, -33.26250000000000284, -97.00000000000000000 ) ) ;
#18304=CARTESIAN_POINT ( 'NONE',  ( -79.64356964374999848, -33.06562499938548427, 99.99999999999998579 ) ) ;
#18305=CARTESIAN_POINT ( 'NONE',  ( 83.77821517812500929, -34.71562499938548285, -97.61286128772489690 ) ) ;
#18309=ADVANCED_FACE ( 'NONE', ( #7748 ), #13705, .F. ) ;
#18310=EDGE_CURVE ( 'NONE', #10782, #12847, #10486, .T. ) ;
#18315=CARTESIAN_POINT ( 'NONE',  ( -79.39999999999999147, -31.98750000000000071, 98.26794919243110371 ) ) ;
#18317=CARTESIAN_POINT ( 'NONE',  ( -85.31192385480822793, -35.00000000000001421, 99.60674545265970892 ) ) ;
#18318=CARTESIAN_POINT ( 'NONE',  ( -80.90000000000000568, -33.75000000000000000, -102.5980762113533018 ) ) ;
#18321=EDGE_CURVE ( 'NONE', #2879, #7789, #15105, .T. ) ;
#18326=CARTESIAN_POINT ( 'NONE',  ( 80.24533121543018410, -31.99999999999996447, 97.95829548583768087 ) ) ;
#18327=CARTESIAN_POINT ( 'NONE',  ( 83.77821517812500929, -30.21562499938548285, 102.3871387122750889 ) ) ;
#18329=CARTESIAN_POINT ( 'NONE',  ( 81.02178482187500208, -32.35312499938548569, -102.3871387122750889 ) ) ;
#18331=CARTESIAN_POINT ( 'NONE',  ( -85.15643035625001289, -34.71562499938548285, 101.5914258081833879 ) ) ;
#18332=CARTESIAN_POINT ( 'NONE',  ( -82.39999999999999147, -34.41562499938547859, -103.1828516163667899 ) ) ;
#18334=CARTESIAN_POINT ( 'NONE',  ( 83.77821517812500929, -31.67812499938548498, 102.3871387122750889 ) ) ;
#18336=CARTESIAN_POINT ( 'NONE',  ( -85.15643035625001289, -33.85312499938549280, 99.99999999999998579 ) ) ;
#18339=CARTESIAN_POINT ( 'NONE',  ( -79.39999999999999147, -31.12500000000000355, -99.99999999999998579 ) ) ;
#18347=EDGE_LOOP ( 'NONE', ( #593, #4884, #16529, #16438 ) ) ;
#18350=CARTESIAN_POINT ( 'NONE',  ( -85.40000000000000568, -33.11250000000000426, 101.7320508075688821 ) ) ;
#18351=DIRECTION ( 'NONE',  ( -0.000000000000000000, -0.000000000000000000, -1.000000000000000000 ) ) ;
#18353=CARTESIAN_POINT ( 'NONE',  ( 81.02178482187500208, -32.35312499938548569, -102.3871387122750889 ) ) ;
#18362=CARTESIAN_POINT ( 'NONE',  ( -85.40000000000000568, -34.91250000000000142, 101.7320508075688821 ) ) ;
#18363=AXIS2_PLACEMENT_3D ( 'NONE', #13068, #6733, #17373 ) ;
#18365=EDGE_CURVE ( 'NONE', #13374, #5491, #17127, .T. ) ;
#18370=ORIENTED_EDGE ( 'NONE', *, *, #8175, .T. ) ;
#18372=CARTESIAN_POINT ( 'NONE',  ( -85.40000000000000568, -32.60624999877097707, -98.26794919243111792 ) ) ;
#18375=CARTESIAN_POINT ( 'NONE',  ( -85.15643035625001289, -35.22676544108147567, 98.99674642581742035 ) ) ;
#18379=DIRECTION ( 'NONE',  ( 0.000000000000000000, -1.000000000000000000, 0.000000000000000000 ) ) ;
#18392=ORIENTED_EDGE ( 'NONE', *, *, #14393, .T. ) ;
#18395=CARTESIAN_POINT ( 'NONE',  ( 79.39999999999999147, -31.57499999999999929, -99.99999999999998579 ) ) ;
#18396=CARTESIAN_POINT ( 'NONE',  ( -79.64356964374999848, -34.97812499938548569, -99.99999999999998579 ) ) ;
#18397=CARTESIAN_POINT ( 'NONE',  ( -80.90000000000000568, -34.14374999877097139, 97.40192378864668399 ) ) ;
#18398=LINE ( 'NONE', #5312, #16625 ) ;
#18399=CARTESIAN_POINT ( 'NONE',  ( 81.02178482187500208, -32.65312499938548996, -97.61286128772489690 ) ) ;
#18402=CARTESIAN_POINT ( 'NONE',  ( -79.64356964374999848, -32.16562499938548569, 99.99999999999998579 ) ) ;
#18403=CARTESIAN_POINT ( 'NONE',  ( 82.39999999999999147, -33.62812499938549138, -103.1828516163667899 ) ) ;
#18406=CARTESIAN_POINT ( 'NONE',  ( -82.39999999999999147, -33.48750000000000426, 103.4641016151377499 ) ) ;
#18407=CARTESIAN_POINT ( 'NONE',  ( 79.68596062386910717, -31.99999999999998579, -101.2782762865714972 ) ) ;
#18411=CARTESIAN_POINT ( 'NONE',  ( -85.40000000000000568, -32.70000000000000284, 99.99999999999998579 ) ) ;
#18415=CARTESIAN_POINT ( 'NONE',  ( 83.77821517812500929, -31.41562499938548569, 97.61286128772489690 ) ) ;
#18416=CARTESIAN_POINT ( 'NONE',  ( 85.14613134194621580, -32.00000000000003553, -99.70214005991869044 ) ) ;
#18418=CARTESIAN_POINT ( 'NONE',  ( 82.15584532983334043, -31.99999999999999289, 97.13032736203115292 ) ) ;
#18419=CARTESIAN_POINT ( 'NONE',  ( 85.15643035625001289, -34.30312499938548854, 99.99999999999998579 ) ) ;
#18420=CARTESIAN_POINT ( 'NONE',  ( 85.15643035625001289, -31.60312499938548569, -99.99999999999998579 ) ) ;
#18422=CARTESIAN_POINT ( 'NONE',  ( -79.77811200999887831, -35.00000000000000000, 100.8506536761481414 ) ) ;
#18423=CARTESIAN_POINT ( 'NONE',  ( -79.64356964375001269, -32.76562499938548711, -98.40857419181659793 ) ) ;
#18426=CARTESIAN_POINT ( 'NONE',  ( 82.39999999999999147, -32.39062499938548001, 96.81714838363319586 ) ) ;
#18428=CARTESIAN_POINT ( 'NONE',  ( -85.15643035624999868, -30.55312499938548854, 101.5914258081833879 ) ) ;
#18430=CARTESIAN_POINT ( 'NONE',  ( -83.77821517812500929, -33.02812499938548285, 97.61286128772489690 ) ) ;
#18431=EDGE_CURVE ( 'NONE', #13374, #13408, #18594, .T. ) ;
#18433=VERTEX_POINT ( 'NONE', #8418 ) ;
#18434=CARTESIAN_POINT ( 'NONE',  ( -85.40000000000000568, -33.11250000000000426, -98.26794919243111792 ) ) ;
#18436=CARTESIAN_POINT ( 'NONE',  ( 82.65333140691205926, -34.99995246259152282, -97.01071553687880566 ) ) ;
#18437=CARTESIAN_POINT ( 'NONE',  ( -96.99999999999998579, 0.000000000000000000, -150.0000000000000000 ) ) ;
#18441=ORIENTED_EDGE ( 'NONE', *, *, #5204, .T. ) ;
#18443=CARTESIAN_POINT ( 'NONE',  ( -85.40000000000000568, -33.58124999877097139, -101.7320508075688821 ) ) ;
#18446=CARTESIAN_POINT ( 'NONE',  ( -85.40000000000000568, -34.48124999877096997, 98.26794919243111792 ) ) ;
#18447=CARTESIAN_POINT ( 'NONE',  ( 83.77821517812500929, -31.07812499938548711, -102.3871387122750889 ) ) ;
#18448=CARTESIAN_POINT ( 'NONE',  ( 82.40000000000000568, -30.00000000000000355, -99.99999999999998579 ) ) ;
#18450=CARTESIAN_POINT ( 'NONE',  ( 79.39999999999999147, -31.48124999877097352, 101.7320508075688821 ) ) ;
#18456=CARTESIAN_POINT ( 'NONE',  ( 82.39999999999999147, -33.20624999877097849, 103.0000000000000000 ) ) ;
#18457=ORIENTED_EDGE ( 'NONE', *, *, #11033, .T. ) ;
#18459=CARTESIAN_POINT ( 'NONE',  ( -83.77821517812500929, -32.01562499938548001, -102.3871387122750889 ) ) ;
#18465=CARTESIAN_POINT ( 'NONE',  ( -82.39999999999999147, -33.88124999877096855, -96.53589838486223584 ) ) ;
#18466=CARTESIAN_POINT ( 'NONE',  ( -82.41196654184768988, -35.00000000000001421, 97.00083539721711645 ) ) ;
#18470=EDGE_CURVE ( 'NONE', #17768, #779, #5117, .T. ) ;
#18475=CARTESIAN_POINT ( 'NONE',  ( -81.59615242270662350, -32.96115380933864003, -97.00000000000000000 ) ) ;
#18476=ORIENTED_EDGE ( 'NONE', *, *, #2657, .T. ) ;
#18477=CARTESIAN_POINT ( 'NONE',  ( -79.39999999999999147, -33.41250000000000142, -98.26794919243113213 ) ) ;
#18480=ORIENTED_EDGE ( 'NONE', *, *, #12618, .F. ) ;
#18481=CARTESIAN_POINT ( 'NONE',  ( -85.40000000000000568, -33.95624999877097139, -98.26794919243111792 ) ) ;
#18483=( BOUNDED_CURVE ( )  B_SPLINE_CURVE ( 2, ( #3736, #12824, #5415, #3830, #9701, #8328, #17032, #17422, #6583 ),
 .UNSPECIFIED., .F., .F. ) 
 B_SPLINE_CURVE_WITH_KNOTS ( ( 3, 2, 2, 2, 3 ),
 ( 0.5208333333333333703, 0.5277777777777777901, 0.5416666666666666297, 0.5555555555555555802, 0.5625000000000000000 ),
 .UNSPECIFIED. ) 
 CURVE ( )  GEOMETRIC_REPRESENTATION_ITEM ( )  RATIONAL_B_SPLINE_CURVE ( ( 0.9330127018922192983, 0.9330127018922198534, 1.000000000000000000, 0.8660254037844387076, 1.000000000000000000, 0.8660254037844387076, 1.000000000000000000, 0.9330127018922194093, 0.9330127018922194093 ) ) 
 REPRESENTATION_ITEM ( '' )  );
#18487=LINE ( 'NONE', #18108, #14759 ) ;
#18488=CARTESIAN_POINT ( 'NONE',  ( 83.90000000000000568, -30.82500000000000284, -102.5980762113533018 ) ) ;
#18489=ADVANCED_FACE ( 'NONE', ( #7241 ), #13010, .F. ) ;
#18491=CARTESIAN_POINT ( 'NONE',  ( -83.90000000000000568, -33.61874999877097281, 97.40192378864668399 ) ) ;
#18493=CARTESIAN_POINT ( 'NONE',  ( -81.59615242270662350, -33.22634618820330843, 97.00000000000000000 ) ) ;
#18495=CARTESIAN_POINT ( 'NONE',  ( 83.77821517812500929, -32.12812499938548427, -97.61286128772489690 ) ) ;
#18497=CARTESIAN_POINT ( 'NONE',  ( -79.64356964375001269, -33.92812499938548854, 98.40857419181659793 ) ) ;
#18499=AXIS2_PLACEMENT_3D ( 'NONE', #15078, #12050, #7649 ) ;
#18500=CARTESIAN_POINT ( 'NONE',  ( 83.77821517812500929, -34.11562499938548854, -102.3871387122750889 ) ) ;
#18504=CARTESIAN_POINT ( 'NONE',  ( 83.20384757729335945, -33.63615380933863008, -96.99999999999998579 ) ) ;
#18505=CARTESIAN_POINT ( 'NONE',  ( 83.90000000000000568, -33.52499999999999858, 97.40192378864668399 ) ) ;
#18508=CARTESIAN_POINT ( 'NONE',  ( -83.90000000000000568, -32.62500000000000000, 102.5980762113533018 ) ) ;
#18511=CIRCLE ( 'NONE', #2281, 5.199999999999996625 ) ;
#18512=CARTESIAN_POINT ( 'NONE',  ( 79.83361526238431338, -35.00000000000000000, 98.97827398863964277 ) ) ;
#18513=CARTESIAN_POINT ( 'NONE',  ( 79.64356964374999848, -33.06562499938548427, 99.99999999999998579 ) ) ;
#18514=CARTESIAN_POINT ( 'NONE',  ( 80.90000000000000568, -32.10000000000000142, -102.5980762113533018 ) ) ;
#18516=CARTESIAN_POINT ( 'NONE',  ( -79.64356964374998427, -32.76562499938548711, -98.40857419181659793 ) ) ;
#18517=CARTESIAN_POINT ( 'NONE',  ( 81.02178482187500208, -31.19062499938548427, 102.3871387122750889 ) ) ;
#18518=CARTESIAN_POINT ( 'NONE',  ( 85.15643035624999868, -32.09062499938548996, -98.40857419181659793 ) ) ;
#18520=CARTESIAN_POINT ( 'NONE',  ( -79.64356964374998427, -34.94062499938548427, 98.40857419181659793 ) ) ;
#18521=CARTESIAN_POINT ( 'NONE',  ( -79.64356964375001269, -34.49062499938548854, -101.5914258081833879 ) ) ;
#18523=CARTESIAN_POINT ( 'NONE',  ( 79.64356964375001269, -32.31562499938548427, 98.40857419181659793 ) ) ;
#18526=CARTESIAN_POINT ( 'NONE',  ( -79.64356964374999848, -33.62812499938548427, 99.99999999999998579 ) ) ;
#18530=CARTESIAN_POINT ( 'NONE',  ( -82.39999999999999147, -34.38750000000000284, -96.53589838486223584 ) ) ;
#18531=DIRECTION ( 'NONE',  ( 0.000000000000000000, -1.000000000000000000, 0.000000000000000000 ) ) ;
#18533=CARTESIAN_POINT ( 'NONE',  ( -84.51155386534844638, -35.25364837475780888, -101.7717924772919957 ) ) ;
#18536=VERTEX_POINT ( 'NONE', #1294 ) ;
#18539=CARTESIAN_POINT ( 'NONE',  ( 85.15643035625001289, -34.67812499938548143, 101.5914258081833879 ) ) ;
#18540=CARTESIAN_POINT ( 'NONE',  ( -94.79999999999999716, 0.000000000000000000, -150.0000000000000000 ) ) ;
#18542=CARTESIAN_POINT ( 'NONE',  ( 79.64356964375001269, -31.41562499938548569, -101.5914258081833879 ) ) ;
#18544=EDGE_CURVE ( 'NONE', #17308, #5485, #13196, .T. ) ;
#18553=ORIENTED_EDGE ( 'NONE', *, *, #13543, .T. ) ;
#18555=CARTESIAN_POINT ( 'NONE',  ( -82.39999999999999147, -30.47812499938548569, -96.81714838363319586 ) ) ;
#18556=CARTESIAN_POINT ( 'NONE',  ( -85.40000000000000568, -32.21250000000000568, -98.26794919243111792 ) ) ;
#18558=CARTESIAN_POINT ( 'NONE',  ( 81.02178482187500208, -32.35312499938548569, 97.61286128772489690 ) ) ;
#18559=CARTESIAN_POINT ( 'NONE',  ( -85.40000000000000568, -34.85624999877096997, -98.26794919243111792 ) ) ;
#18560=CARTESIAN_POINT ( 'NONE',  ( 82.39999999999999147, -34.83749999999999858, 96.53589838486223584 ) ) ;
#18565=PRODUCT_DEFINITION_SHAPE ( 'NONE', 'NONE',  #14653 ) ;
#18567=CARTESIAN_POINT ( 'NONE',  ( 80.90000000000000568, -34.29374999877096997, -102.5980762113533018 ) ) ;
#18568=EDGE_CURVE ( 'NONE', #19033, #7323, #19064, .T. ) ;
#18572=ORIENTED_EDGE ( 'NONE', *, *, #11276, .F. ) ;
#18574=CARTESIAN_POINT ( 'NONE',  ( 82.39999999999999147, -32.50312499938548427, -96.81714838363319586 ) ) ;
#18586=CARTESIAN_POINT ( 'NONE',  ( -82.40000000000001990, -32.13750000000000284, -97.00000000000000000 ) ) ;
#18587=CARTESIAN_POINT ( 'NONE',  ( 80.90000000000000568, -30.60000000000000142, -97.40192378864668399 ) ) ;
#18588=CYLINDRICAL_SURFACE ( 'NONE', #4555, 3.000000000000002665 ) ;
#18589=CARTESIAN_POINT ( 'NONE',  ( -79.39999999999999147, -34.63124999877096855, 98.26794919243110371 ) ) ;
#18593=CARTESIAN_POINT ( 'NONE',  ( 85.40000000000000568, -33.95624999877097139, 98.26794919243111792 ) ) ;
#18594=LINE ( 'NONE', #8323, #9303 ) ;
#18595=CARTESIAN_POINT ( 'NONE',  ( -83.77821517812500929, -32.91562499938547859, 97.61286128772489690 ) ) ;
#18597=CARTESIAN_POINT ( 'NONE',  ( -84.70388354820684640, -35.00002705695768412, 98.07851859032987818 ) ) ;
#18601=CARTESIAN_POINT ( 'NONE',  ( -83.90000000000000568, -34.87500000000000000, 102.5980762113533018 ) ) ;
#18612=CARTESIAN_POINT ( 'NONE',  ( 81.02178482187500208, -31.79062499938548925, 97.61286128772489690 ) ) ;
#18615=CARTESIAN_POINT ( 'NONE',  ( 83.74167325096738068, -32.00000000000000000, 97.53412486788937485 ) ) ;
#18616=CARTESIAN_POINT ( 'NONE',  ( 82.39999999999999147, -31.82812499938548356, 96.81714838363319586 ) ) ;
#18617=CARTESIAN_POINT ( 'NONE',  ( 85.15643035625001289, -32.95312499938548711, -99.99999999999998579 ) ) ;
#18619=CARTESIAN_POINT ( 'NONE',  ( -85.15643035625001289, -33.89062499938548711, 98.40857419181659793 ) ) ;
#18620=CARTESIAN_POINT ( 'NONE',  ( -82.39999999999999147, -31.60312499938548569, -103.1828516163667899 ) ) ;
#18622=CARTESIAN_POINT ( 'NONE',  ( 83.77821517812500929, -31.97812499938548925, 97.61286128772489690 ) ) ;
#18625=CARTESIAN_POINT ( 'NONE',  ( -81.02178482187500208, -31.64062499938548356, 97.61286128772489690 ) ) ;
#18626=CARTESIAN_POINT ( 'NONE',  ( -85.15643035624999868, -33.89062499938548711, 98.40857419181659793 ) ) ;
#18627=DIRECTION ( 'NONE',  ( 0.000000000000000000, -1.000000000000000000, 0.000000000000000000 ) ) ;
#18629=CARTESIAN_POINT ( 'NONE',  ( -80.90000000000000568, -33.00000000000000000, -97.40192378864668399 ) ) ;
#18630=CARTESIAN_POINT ( 'NONE',  ( -79.64356964375001269, -31.86562499938548143, -98.40857419181659793 ) ) ;
#18631=CARTESIAN_POINT ( 'NONE',  ( 80.90000000000000568, -32.85000000000000142, -97.40192378864668399 ) ) ;
#18632=CARTESIAN_POINT ( 'NONE',  ( 84.42750213138106119, -35.00000000000000000, -97.77995849557630947 ) ) ;
#18635=CARTESIAN_POINT ( 'NONE',  ( -83.90000000000000568, -34.81874999877096855, 102.5980762113533018 ) ) ;
#18637=CARTESIAN_POINT ( 'NONE',  ( -83.90000000000000568, -33.16874999877096286, -102.5980762113533018 ) ) ;
#18638=DIRECTION ( 'NONE',  ( 1.000000000000000000, 3.548298019043479384E-15, 0.000000000000000000 ) ) ;
#18641=CARTESIAN_POINT ( 'NONE',  ( 81.02178482187500208, -31.45312499938549067, -102.3871387122750889 ) ) ;
#18645=CARTESIAN_POINT ( 'NONE',  ( 80.90000000000000568, -30.54374999877096997, 102.5980762113533018 ) ) ;
#18649=VECTOR ( 'NONE', #9548, 1000.000000000000000 ) ;
#18653=ORIENTED_EDGE ( 'NONE', *, *, #9586, .T. ) ;
#18655=CARTESIAN_POINT ( 'NONE',  ( -79.64356964374999848, -32.61562499938548854, -99.99999999999998579 ) ) ;
#18658=CARTESIAN_POINT ( 'NONE',  ( 79.64356964374998427, -34.11562499938548854, 98.40857419181659793 ) ) ;
#18660=CARTESIAN_POINT ( 'NONE',  ( -83.90000000000000568, -33.91874999877096997, -97.40192378864668399 ) ) ;
#18661=CARTESIAN_POINT ( 'NONE',  ( 80.90000000000000568, -33.89999999999999858, 97.40192378864668399 ) ) ;
#18666=CARTESIAN_POINT ( 'NONE',  ( 84.70388354820684640, -35.00002705695777649, -98.07851859032987818 ) ) ;
#18667=ADVANCED_FACE ( 'NONE', ( #7819 ), #17994, .F. ) ;
#18668=EDGE_CURVE ( 'NONE', #14513, #13499, #12022, .T. ) ;
#18672=ORIENTED_EDGE ( 'NONE', *, *, #11558, .F. ) ;
#18673=CARTESIAN_POINT ( 'NONE',  ( 79.64356964374998427, -32.12812499938548427, -98.40857419181659793 ) ) ;
#18683=EDGE_CURVE ( 'NONE', #5783, #12300, #3121, .T. ) ;
#18684=ORIENTED_EDGE ( 'NONE', *, *, #4701, .T. ) ;
#18685=( BOUNDED_CURVE ( )  B_SPLINE_CURVE ( 2, ( #14277, #17317, #12819, #18882, #17415, #11451, #723, #11157, #12289, #3291, #1735, #11996, #1557, #13746, #5951, #7792, #1646, #384, #10532, #10815, #12188, #13461, #16397, #18157, #12093, #10433, #3197, #6142, #15216, #16500, #4779, #14933, #6337, #6049, #4480, #13552, #4677, #17869, #16592, #7693, #9251, #15026, #18254, #18066, #3007, #8965, #97, #2, #7504, #1832, #17964, #9156, #10627, #15119, #4574, #11898, #3103, #1453, #9061, #13650, #7599, #192, #13369, #292, #4871, #6241, #10722, #16686, #7406, #16782, #3396, #14555, #3584, #18539, #5358, #6718, #8084, #860, #479, #2308, #6823, #17267, #14127 ),
 .UNSPECIFIED., .F., .F. ) 
 B_SPLINE_CURVE_WITH_KNOTS ( ( 3, 2, 2, 2, 2, 2, 2, 2, 2, 2, 2, 2, 2, 2, 2, 2, 2, 2, 2, 2, 2, 2, 2, 2, 2, 2, 2, 2, 2, 2, 2, 2, 2, 2, 2, 2, 2, 2, 2, 2, 2, 3 ),
 ( 0.3716916592825996735, 0.3750191855951752751, 0.3900199530189822905, 0.4050207204427893615, 0.4200214878665963769, 0.4350222552904033924, 0.4500230227142104078, 0.4650237901380174232, 0.4800245575618243832, 0.4950253249856314541, 0.5100260924094384141, 0.5250268598332454850, 0.5400276272570524450, 0.5550283946808594049, 0.5700291621046664758, 0.5850299295284735468, 0.6000306969522806178, 0.6150314643760875777, 0.6300322317998945376, 0.6450329992237016086, 0.6600337666475086795, 0.6750345340713156395, 0.6900353014951225994, 0.7050360689189296703, 0.7200368363427367413, 0.7350376037665437012, 0.7500383711903506612, 0.7650391386141577321, 0.7800399060379648031, 0.7950406734617718740, 0.8100414408855787229, 0.8250422083093857939, 0.8400429757331928649, 0.8550437431569998248, 0.8700445105808068957, 0.8850452780046138557, 0.9000460454284209266, 0.9150468128522277755, 0.9300475802760350685, 0.9450483476998419174, 0.9600491151236487664, 0.9717223562348824561 ),
 .UNSPECIFIED. ) 
 CURVE ( )  GEOMETRIC_REPRESENTATION_ITEM ( )  RATIONAL_B_SPLINE_CURVE ( ( 0.9537471549766856072, 0.9702812541832720461, 1.000000000000000000, 0.8660254037844387076, 1.000000000000000000, 0.8660254037844387076, 1.000000000000000000, 0.8660254037844387076, 1.000000000000000000, 0.8660254037844387076, 1.000000000000000000, 0.8660254037844387076, 1.000000000000000000, 0.8660254037844387076, 1.000000000000000000, 0.8660254037844387076, 1.000000000000000000, 0.8660254037844387076, 1.000000000000000000, 0.8660254037844387076, 1.000000000000000000, 0.8660254037844387076, 1.000000000000000000, 0.8660254037844387076, 1.000000000000000000, 0.8660254037844387076, 1.000000000000000000, 0.8660254037844387076, 1.000000000000000000, 0.8660254037844387076, 1.000000000000000000, 0.8660254037844387076, 1.000000000000000000, 0.8660254037844387076, 1.000000000000000000, 0.8660254037844387076, 1.000000000000000000, 0.8660254037844387076, 1.000000000000000000, 0.8660254037844387076, 1.000000000000000000, 0.8660254037844387076, 1.000000000000000000, 0.8660254037844387076, 1.000000000000000000, 0.8660254037844387076, 1.000000000000000000, 0.8660254037844387076, 1.000000000000000000, 0.8660254037844387076, 1.000000000000000000, 0.8660254037844387076, 1.000000000000000000, 0.8660254037844387076, 1.000000000000000000, 0.8660254037844387076, 1.000000000000000000, 0.8660254037844387076, 1.000000000000000000, 0.8660254037844387076, 1.000000000000000000, 0.8660254037844387076, 1.000000000000000000, 0.8660254037844387076, 1.000000000000000000, 0.8660254037844387076, 1.000000000000000000, 0.8660254037844387076, 1.000000000000000000, 0.8660254037844387076, 1.000000000000000000, 0.8660254037844387076, 1.000000000000000000, 0.8660254037844387076, 1.000000000000000000, 0.8660254037844387076, 1.000000000000000000, 0.8660254037844387076, 1.000000000000000000, 0.8660254037844387076, 1.000000000000000000, 0.8957441496011472326, 0.9537471549767071455 ) ) 
 REPRESENTATION_ITEM ( '' )  );
#18688=CARTESIAN_POINT ( 'NONE',  ( 85.40000000000000568, -32.25000000000000000, -99.99999999999998579 ) ) ;
#18689=DIRECTION ( 'NONE',  ( 0.000000000000000000, 0.000000000000000000, -1.000000000000000000 ) ) ;
#18691=CARTESIAN_POINT ( 'NONE',  ( -79.39999999999999147, -33.28124999877096712, 98.26794919243110371 ) ) ;
#18693=CARTESIAN_POINT ( 'NONE',  ( 85.40000000000000568, -32.25000000000000000, -99.99999999999998579 ) ) ;
#18694=CARTESIAN_POINT ( 'NONE',  ( 99.99999999999994316, -29.80000000000000782, -150.0000000000000000 ) ) ;
#18696=CARTESIAN_POINT ( 'NONE',  ( 83.20384757729335945, -34.08615380933863293, 102.9999999999999858 ) ) ;
#18698=DIRECTION ( 'NONE',  ( 0.000000000000000000, -1.000000000000000000, 0.000000000000000000 ) ) ;
#18699=CARTESIAN_POINT ( 'NONE',  ( -85.15643035624999868, -33.77812499938548285, 98.40857419181659793 ) ) ;
#18701=ORIENTED_EDGE ( 'NONE', *, *, #10457, .F. ) ;
#18702=DIRECTION ( 'NONE',  ( 0.000000000000000000, 1.000000000000000000, 0.000000000000000000 ) ) ;
#18706=ORIENTED_EDGE ( 'NONE', *, *, #1350, .F. ) ;
#18707=CARTESIAN_POINT ( 'NONE',  ( -82.65333140691201663, -34.99995246259153703, 97.01071553687880566 ) ) ;
#18710=CARTESIAN_POINT ( 'NONE',  ( 81.02178482187500208, -33.14062499938548711, 97.61286128772489690 ) ) ;
#18714=CARTESIAN_POINT ( 'NONE',  ( -85.15643035625001289, -33.85312499938549280, -99.99999999999998579 ) ) ;
#18715=CARTESIAN_POINT ( 'NONE',  ( 79.64356964375001269, -33.10312499938549280, 98.40857419181659793 ) ) ;
#18716=( BOUNDED_CURVE ( )  B_SPLINE_CURVE ( 2, ( #11882, #7585, #17850, #18142, #15104, #7294, #9140, #10515, #1629 ),
 .UNSPECIFIED., .F., .T. ) 
 B_SPLINE_CURVE_WITH_KNOTS ( ( 3, 2, 2, 2, 3 ),
 ( 0.7291666666666666297, 0.7361111111111111605, 0.7500000000000000000, 0.7638888888888888395, 0.7708333333333331483 ),
 .UNSPECIFIED. ) 
 CURVE ( )  GEOMETRIC_REPRESENTATION_ITEM ( )  RATIONAL_B_SPLINE_CURVE ( ( 0.9330127018922192983, 0.9330127018922187432, 1.000000000000000000, 0.8660254037844387076, 1.000000000000000000, 0.8660254037844387076, 1.000000000000000000, 0.9330127018922209636, 0.9330127018922194093 ) ) 
 REPRESENTATION_ITEM ( '' )  );
#18717=CARTESIAN_POINT ( 'NONE',  ( 82.39999999999999147, -33.74062499938548854, -103.1828516163667899 ) ) ;
#18720=CARTESIAN_POINT ( 'NONE',  ( -83.77821517812500929, -33.21562499938548285, 102.3871387122750889 ) ) ;
#18722=CARTESIAN_POINT ( 'NONE',  ( 79.64356964375001269, -32.24062499938548854, 101.5914258081833879 ) ) ;
#18725=FACE_OUTER_BOUND ( 'NONE', #16582, .T. ) ;
#18726=CARTESIAN_POINT ( 'NONE',  ( -83.77821517812500929, -31.56562499938548427, 97.61286128772489690 ) ) ;
#18729=CARTESIAN_POINT ( 'NONE',  ( -82.39999999999999147, -33.48750000000000426, -96.53589838486223584 ) ) ;
#18731=LINE ( 'NONE', #11093, #80 ) ;
#18736=CARTESIAN_POINT ( 'NONE',  ( -82.40000000000000568, -34.78124999877096712, 102.9999999999999858 ) ) ;
#18738=CARTESIAN_POINT ( 'NONE',  ( -83.20384757729335945, -33.63615380933863008, -102.9999999999999716 ) ) ;
#18739=CARTESIAN_POINT ( 'NONE',  ( 83.77821517812500929, -31.22812499938548569, 102.3871387122750889 ) ) ;
#18741=CARTESIAN_POINT ( 'NONE',  ( -85.40000000000000568, -32.70000000000000284, -99.99999999999998579 ) ) ;
#18742=CARTESIAN_POINT ( 'NONE',  ( 79.64356964375001269, -30.51562499938548711, -101.5914258081833879 ) ) ;
#18745=CARTESIAN_POINT ( 'NONE',  ( 79.39999999999999147, -31.06874999877096855, 99.99999999999998579 ) ) ;
#18750=CARTESIAN_POINT ( 'NONE',  ( -84.59935209580211790, -35.00000000000002842, -98.20719995774828703 ) ) ;
#18751=ORIENTED_EDGE ( 'NONE', *, *, #16270, .T. ) ;
#18752=CARTESIAN_POINT ( 'NONE',  ( -81.02178482187500208, -31.34062499938548996, -97.61286128772489690 ) ) ;
#18755=CARTESIAN_POINT ( 'NONE',  ( 82.39999999999999147, -34.64062499938548711, 96.81714838363319586 ) ) ;
#18756=CARTESIAN_POINT ( 'NONE',  ( -82.39999999999999147, -31.26562499938549067, -103.1828516163667899 ) ) ;
#18757=CARTESIAN_POINT ( 'NONE',  ( 79.39999999999999147, -33.78750000000000142, 101.7320508075688821 ) ) ;
#18758=CARTESIAN_POINT ( 'NONE',  ( -79.64057174634726266, -35.00000000000000000, 100.3964642588222063 ) ) ;
#18761=CARTESIAN_POINT ( 'NONE',  ( -81.02178482187500208, -32.54062499938548569, -102.3871387122750889 ) ) ;
#18765=CARTESIAN_POINT ( 'NONE',  ( 81.02178482187500208, -32.99062499938548854, -97.61286128772489690 ) ) ;
#18774=CARTESIAN_POINT ( 'NONE',  ( -83.90000000000000568, -34.06874999877096855, -102.5980762113533018 ) ) ;
#18778=CARTESIAN_POINT ( 'NONE',  ( 85.40000000000000568, -33.14999999999999858, -99.99999999999998579 ) ) ;
#18779=CARTESIAN_POINT ( 'NONE',  ( 84.29633955546289314, -32.00000000000002132, -102.0295751981968806 ) ) ;
#18780=CARTESIAN_POINT ( 'NONE',  ( -83.77821517812500929, -32.57812499938548711, 97.61286128772489690 ) ) ;
#18784=CARTESIAN_POINT ( 'NONE',  ( 82.39999999999999147, -34.64062499938548711, -103.1828516163667899 ) ) ;
#18786=CARTESIAN_POINT ( 'NONE',  ( -85.15643035624999868, -34.60312499938548569, 101.5914258081833879 ) ) ;
#18793=( BOUNDED_CURVE ( )  B_SPLINE_CURVE ( 2, ( #16086, #6915, #15800, #3970, #4263, #19114, #2500, #2405, #8369 ),
 .UNSPECIFIED., .F., .F. ) 
 B_SPLINE_CURVE_WITH_KNOTS ( ( 3, 2, 2, 2, 3 ),
 ( 0.3541666666666666297, 0.3611111111111111049, 0.3750000000000000000, 0.3888888888888888951, 0.3958333333333334259 ),
 .UNSPECIFIED. ) 
 CURVE ( )  GEOMETRIC_REPRESENTATION_ITEM ( )  RATIONAL_B_SPLINE_CURVE ( ( 0.9330127018922194093, 0.9330127018922190762, 1.000000000000000000, 0.8660254037844387076, 1.000000000000000000, 0.8660254037844387076, 1.000000000000000000, 0.9330127018922185211, 0.9330127018922192983 ) ) 
 REPRESENTATION_ITEM ( '' )  );
#18798=EDGE_CURVE ( 'NONE', #7737, #4219, #18185, .T. ) ;
#18799=VERTEX_POINT ( 'NONE', #11926 ) ;
#18802=CARTESIAN_POINT ( 'NONE',  ( -83.04276107155152431, -35.00000000000000000, -102.9375709370400784 ) ) ;
#18803=CARTESIAN_POINT ( 'NONE',  ( 83.77821517812500929, -32.46562499938548285, 102.3871387122750889 ) ) ;
#18807=ADVANCED_FACE ( 'NONE', ( #7625, #3423, #9373 ), #13680, .T. ) ;
#18809=CARTESIAN_POINT ( 'NONE',  ( -83.77821517812500929, -33.02812499938548285, -102.3871387122750889 ) ) ;
#18810=CARTESIAN_POINT ( 'NONE',  ( 83.77821517812500929, -31.56562499938548427, 102.3871387122750889 ) ) ;
#18812=CARTESIAN_POINT ( 'NONE',  ( 82.39999999999999147, -34.64062499938548711, -103.1828516163667899 ) ) ;
#18814=CARTESIAN_POINT ( 'NONE',  ( -79.64356964374999848, -33.96562499938548285, 99.99999999999998579 ) ) ;
#18815=CARTESIAN_POINT ( 'NONE',  ( 83.77821517812500929, -31.11562499938548498, -97.61286128772489690 ) ) ;
#18819=CARTESIAN_POINT ( 'NONE',  ( 82.39999999999999147, -34.19062499938548427, 96.81714838363319586 ) ) ;
#18822=AXIS2_PLACEMENT_3D ( 'NONE', #4676, #17868, #7692 ) ;
#18823=CARTESIAN_POINT ( 'NONE',  ( -85.15643035624999868, -32.87812499938549138, 98.40857419181659793 ) ) ;
#18824=CARTESIAN_POINT ( 'NONE',  ( -79.64356964374999848, -30.36562499938548498, 99.99999999999998579 ) ) ;
#18825=CYLINDRICAL_SURFACE ( 'NONE', #18046, 3.000000000000002665 ) ;
#18826=CARTESIAN_POINT ( 'NONE',  ( -85.12124608221316180, -31.99999999999999289, 99.52644304241999862 ) ) ;
#18828=CARTESIAN_POINT ( 'NONE',  ( 83.95700771753406855, -35.00000000000000000, -97.42750194505821071 ) ) ;
#18834=DIRECTION ( 'NONE',  ( 0.000000000000000000, 0.000000000000000000, 1.000000000000000000 ) ) ;
#18836=CARTESIAN_POINT ( 'NONE',  ( 82.39999999999999147, -31.04062499938548569, 96.81714838363319586 ) ) ;
#18838=CARTESIAN_POINT ( 'NONE',  ( 82.40000000000000568, -30.00000000000000355, -103.0000000000000000 ) ) ;
#18839=CARTESIAN_POINT ( 'NONE',  ( 81.02178482187500208, -32.80312499938548854, -102.3871387122750889 ) ) ;
#18841=CARTESIAN_POINT ( 'NONE',  ( 82.39999999999999147, -32.08124999877097139, 96.53589838486223584 ) ) ;
#18843=EDGE_CURVE ( 'NONE', #11212, #14259, #17747, .T. ) ;
#18847=EDGE_LOOP ( 'NONE', ( #10553, #1749, #9213, #9011 ) ) ;
#18848=CARTESIAN_POINT ( 'NONE',  ( -81.02178482187500208, -31.79062499938548925, -97.61286128772489690 ) ) ;
#18849=FACE_OUTER_BOUND ( 'NONE', #11718, .T. ) ;
#18851=CARTESIAN_POINT ( 'NONE',  ( 79.64356964374999848, -32.72812499938548569, 99.99999999999998579 ) ) ;
#18852=EDGE_CURVE ( 'NONE', #15758, #11084, #5263, .T. ) ;
#18853=CARTESIAN_POINT ( 'NONE',  ( -81.02178482187500208, -31.45312499938549067, -97.61286128772489690 ) ) ;
#18855=CARTESIAN_POINT ( 'NONE',  ( 83.90000000000000568, -34.87500000000000000, 97.40192378864668399 ) ) ;
#18859=CARTESIAN_POINT ( 'NONE',  ( -85.15643035625001289, -33.32812499938548711, -101.5914258081833879 ) ) ;
#18861=CARTESIAN_POINT ( 'NONE',  ( 85.40000000000000568, -30.84374999877096712, -99.99999999999998579 ) ) ;
#18863=EDGE_LOOP ( 'NONE', ( #5293, #3530, #12492, #5006 ) ) ;
#18864=CARTESIAN_POINT ( 'NONE',  ( 79.64356964374998427, -34.00312499938548427, -101.5914258081833879 ) ) ;
#18869=CARTESIAN_POINT ( 'NONE',  ( 79.39999999999997726, -32.01330983656912110, 100.5399455202950492 ) ) ;
#18870=EDGE_LOOP ( 'NONE', ( #2763, #12487, #15831, #5581 ) ) ;
#18872=AXIS2_PLACEMENT_3D ( 'NONE', #12345, #4835, #6785 ) ;
#18874=ORIENTED_EDGE ( 'NONE', *, *, #3170, .T. ) ;
#18876=CARTESIAN_POINT ( 'NONE',  ( 83.90000000000000568, -31.87500000000000000, -97.40192378864668399 ) ) ;
#18877=LINE ( 'NONE', #20, #12665 ) ;
#18878=CARTESIAN_POINT ( 'NONE',  ( -81.02178482187500208, -32.20312499938548711, 97.61286128772489690 ) ) ;
#18882=CARTESIAN_POINT ( 'NONE',  ( 82.39999999999999147, -32.05312499938548854, 103.1828516163667899 ) ) ;
#18883=DIRECTION ( 'NONE',  ( 0.000000000000000000, -1.000000000000000000, 0.000000000000000000 ) ) ;
#18884=CARTESIAN_POINT ( 'NONE',  ( -83.77821517812500929, -35.01562499938548711, 102.3871387122750889 ) ) ;
#18885=( BOUNDED_SURFACE ( )  B_SPLINE_SURFACE ( 1, 2, ( 
 ( #8432, #9907, #8338, #15958, #1024, #6976, #8527, #7166, #2564, #14477, #13024, #9104, #9198, #15067, #235, #16253, #7355, #340, #13312, #4626, #11847, #5992, #1598, #2862, #3052, #10579, #19286, #7453, #4425, #1688, #18204, #5901, #12236, #6191, #14975, #8911, #13411, #16636, #10667, #9015, #6287, #16545, #10384, #4823, #8819, #16346, #14775, #1403, #2956, #1779, #14872, #4724, #12039, #17815, #1501, #7640, #15161, #12141, #13594, #41, #6092, #17914, #4520, #11943, #13503, #18110, #10478, #142, #3144, #3240, #16443, #18013, #7545, #7741, #13699, #14081, #9692, #18691, #16835, #6476, #13884, #9297, #13791, #5205, #15460, #7837, #18491, #1976, #17121, #15262, #8129, #12520, #12429, #6771, #719, #9492, #2260, #2070, #15654, #11052, #18397, #8229, #435, #7933, #5017, #6675, #1877, #6380, #10958, #12616, #17021, #18298, #10763, #18589, #3631, #522, #3441, #12332, #11152, #4917, #3727, #9594, #16926, #3538, #14177, #8027, #2172, #10863, #812, #12719, #16728, #9392, #13986, #624, #15358 ),
 ( #3337, #6572, #5111, #15558, #1289, #15750, #6868, #16133, #3920, #14456, #4116, #10078, #8602, #2743, #11543, #17214, #8504, #909, #8704, #7147, #1192, #14552, #7237, #12910, #1088, #13192, #17313, #9887, #13098, #14654, #5687, #5308, #8318, #17411, #2356, #14366, #16036, #15849, #2542, #2458, #19068, #5598, #15940, #1003, #11250, #4024, #8414, #4211, #3819, #6958, #14272, #2637, #18878, #11636, #5500, #9788, #12815, #17598, #11447, #9985, #10170, #5405, #18780, #11348, #7046, #13004, #18975, #17505, #14848, #15045, #5776, #1576, #10362, #3029, #17795, #10558, #16519, #14951, #7524, #8989, #13480, #4405, #13387, #16326, #211, #120, #10455, #11828, #6167, #2935, #5971, #3122, #1757, #3219, #7332, #11728, #17696, #13285, #4696, #19260, #7620, #6069, #1385, #2840, #9079, #18088, #1668, #13572, #5878, #12015, #1473, #7430, #21, #16419, #12117, #4311, #17988, #4599, #10645, #9177, #16613, #8888, #15141, #7715, #19163, #10274, #16235, #11921, #17892, #4500, #8797, #14752, #8106, #18375, #10741 ) ),
 .UNSPECIFIED., .F., .F., .F. ) 
 B_SPLINE_SURFACE_WITH_KNOTS ( ( 2, 2 ),
 ( 3, 2, 2, 2, 2, 2, 2, 2, 2, 2, 2, 2, 2, 2, 2, 2, 2, 2, 2, 2, 2, 2, 2, 2, 2, 2, 2, 2, 2, 2, 2, 2, 2, 2, 2, 2, 2, 2, 2, 2, 2, 2, 2, 2, 2, 2, 2, 2, 2, 2, 2, 2, 2, 2, 2, 2, 2, 2, 2, 2, 2, 2, 2, 2, 2, 2, 2, 3 ),
 ( 0.000000000000000000, 1.000000000000000000 ),
 ( 0.000000000000000000, 0.01388888888888888812, 0.02777777777777777624, 0.04166666666666666435, 0.05555555555555555247, 0.06944444444444444753, 0.08333333333333332871, 0.09722222222222222376, 0.1111111111111111049, 0.1250000000000000000, 0.1388888888888888951, 0.1527777777777777901, 0.1666666666666666574, 0.1805555555555555525, 0.1944444444444444475, 0.2083333333333333426, 0.2222222222222222099, 0.2361111111111111049, 0.2500000000000000000, 0.2638888888888888951, 0.2777777777777777901, 0.2916666666666666852, 0.3055555555555555802, 0.3194444444444444198, 0.3333333333333333148, 0.3472222222222222099, 0.3611111111111111049, 0.3750000000000000000, 0.3888888888888888951, 0.4027777777777777901, 0.4166666666666666852, 0.4305555555555555802, 0.4444444444444444198, 0.4583333333333333148, 0.4722222222222222099, 0.4861111111111111049, 0.5000000000000000000, 0.5138888888888888395, 0.5277777777777777901, 0.5416666666666666297, 0.5555555555555555802, 0.5694444444444444198, 0.5833333333333333703, 0.5972222222222222099, 0.6111111111111111605, 0.6250000000000000000, 0.6388888888888888395, 0.6527777777777777901, 0.6666666666666666297, 0.6805555555555555802, 0.6944444444444444198, 0.7083333333333333703, 0.7222222222222222099, 0.7361111111111111605, 0.7500000000000000000, 0.7638888888888888395, 0.7777777777777777901, 0.7916666666666666297, 0.8055555555555555802, 0.8194444444444444198, 0.8333333333333333703, 0.8472222222222222099, 0.8611111111111111605, 0.8750000000000000000, 0.8888888888888888395, 0.9027777777777777901, 0.9166666666666666297, 0.9258785144422092550 ),
 .UNSPECIFIED. ) 
 GEOMETRIC_REPRESENTATION_ITEM ( )  RATIONAL_B_SPLINE_SURFACE ( (
 ( 1.000000000000000000, 0.8660254037844387076, 1.000000000000000000, 0.8660254037844387076, 1.000000000000000000, 0.8660254037844387076, 1.000000000000000000, 0.8660254037844387076, 1.000000000000000000, 0.8660254037844387076, 1.000000000000000000, 0.8660254037844387076, 1.000000000000000000, 0.8660254037844387076, 1.000000000000000000, 0.8660254037844387076, 1.000000000000000000, 0.8660254037844387076, 1.000000000000000000, 0.8660254037844387076, 1.000000000000000000, 0.8660254037844387076, 1.000000000000000000, 0.8660254037844387076, 1.000000000000000000, 0.8660254037844387076, 1.000000000000000000, 0.8660254037844387076, 1.000000000000000000, 0.8660254037844387076, 1.000000000000000000, 0.8660254037844387076, 1.000000000000000000, 0.8660254037844387076, 1.000000000000000000, 0.8660254037844387076, 1.000000000000000000, 0.8660254037844387076, 1.000000000000000000, 0.8660254037844387076, 1.000000000000000000, 0.8660254037844387076, 1.000000000000000000, 0.8660254037844387076, 1.000000000000000000, 0.8660254037844387076, 1.000000000000000000, 0.8660254037844387076, 1.000000000000000000, 0.8660254037844387076, 1.000000000000000000, 0.8660254037844387076, 1.000000000000000000, 0.8660254037844387076, 1.000000000000000000, 0.8660254037844387076, 1.000000000000000000, 0.8660254037844387076, 1.000000000000000000, 0.8660254037844387076, 1.000000000000000000, 0.8660254037844387076, 1.000000000000000000, 0.8660254037844387076, 1.000000000000000000, 0.8660254037844387076, 1.000000000000000000, 0.8660254037844387076, 1.000000000000000000, 0.8660254037844387076, 1.000000000000000000, 0.8660254037844387076, 1.000000000000000000, 0.8660254037844387076, 1.000000000000000000, 0.8660254037844387076, 1.000000000000000000, 0.8660254037844387076, 1.000000000000000000, 0.8660254037844387076, 1.000000000000000000, 0.8660254037844387076, 1.000000000000000000, 0.8660254037844387076, 1.000000000000000000, 0.8660254037844387076, 1.000000000000000000, 0.8660254037844387076, 1.000000000000000000, 0.8660254037844387076, 1.000000000000000000, 0.8660254037844387076, 1.000000000000000000, 0.8660254037844387076, 1.000000000000000000, 0.8660254037844387076, 1.000000000000000000, 0.8660254037844387076, 1.000000000000000000, 0.8660254037844387076, 1.000000000000000000, 0.8660254037844387076, 1.000000000000000000, 0.8660254037844387076, 1.000000000000000000, 0.8660254037844387076, 1.000000000000000000, 0.8660254037844387076, 1.000000000000000000, 0.8660254037844387076, 1.000000000000000000, 0.8660254037844387076, 1.000000000000000000, 0.8660254037844387076, 1.000000000000000000, 0.8660254037844387076, 1.000000000000000000, 0.8660254037844387076, 1.000000000000000000, 0.8660254037844387076, 1.000000000000000000, 0.8660254037844387076, 1.000000000000000000, 0.8660254037844387076, 1.000000000000000000, 0.8660254037844387076, 1.000000000000000000, 0.8660254037844387076, 1.000000000000000000, 0.8660254037844387076, 1.000000000000000000, 0.8660254037844387076, 1.000000000000000000, 0.9111409417988175496, 0.9401539645359766606),
 ( 1.000000000000000000, 0.8660254037844387076, 1.000000000000000000, 0.8660254037844387076, 1.000000000000000000, 0.8660254037844387076, 1.000000000000000000, 0.8660254037844387076, 1.000000000000000000, 0.8660254037844387076, 1.000000000000000000, 0.8660254037844387076, 1.000000000000000000, 0.8660254037844387076, 1.000000000000000000, 0.8660254037844387076, 1.000000000000000000, 0.8660254037844387076, 1.000000000000000000, 0.8660254037844387076, 1.000000000000000000, 0.8660254037844387076, 1.000000000000000000, 0.8660254037844387076, 1.000000000000000000, 0.8660254037844387076, 1.000000000000000000, 0.8660254037844387076, 1.000000000000000000, 0.8660254037844387076, 1.000000000000000000, 0.8660254037844387076, 1.000000000000000000, 0.8660254037844387076, 1.000000000000000000, 0.8660254037844387076, 1.000000000000000000, 0.8660254037844387076, 1.000000000000000000, 0.8660254037844387076, 1.000000000000000000, 0.8660254037844387076, 1.000000000000000000, 0.8660254037844387076, 1.000000000000000000, 0.8660254037844387076, 1.000000000000000000, 0.8660254037844387076, 1.000000000000000000, 0.8660254037844387076, 1.000000000000000000, 0.8660254037844387076, 1.000000000000000000, 0.8660254037844387076, 1.000000000000000000, 0.8660254037844387076, 1.000000000000000000, 0.8660254037844387076, 1.000000000000000000, 0.8660254037844387076, 1.000000000000000000, 0.8660254037844387076, 1.000000000000000000, 0.8660254037844387076, 1.000000000000000000, 0.8660254037844387076, 1.000000000000000000, 0.8660254037844387076, 1.000000000000000000, 0.8660254037844387076, 1.000000000000000000, 0.8660254037844387076, 1.000000000000000000, 0.8660254037844387076, 1.000000000000000000, 0.8660254037844387076, 1.000000000000000000, 0.8660254037844387076, 1.000000000000000000, 0.8660254037844387076, 1.000000000000000000, 0.8660254037844387076, 1.000000000000000000, 0.8660254037844387076, 1.000000000000000000, 0.8660254037844387076, 1.000000000000000000, 0.8660254037844387076, 1.000000000000000000, 0.8660254037844387076, 1.000000000000000000, 0.8660254037844387076, 1.000000000000000000, 0.8660254037844387076, 1.000000000000000000, 0.8660254037844387076, 1.000000000000000000, 0.8660254037844387076, 1.000000000000000000, 0.8660254037844387076, 1.000000000000000000, 0.8660254037844387076, 1.000000000000000000, 0.8660254037844387076, 1.000000000000000000, 0.8660254037844387076, 1.000000000000000000, 0.8660254037844387076, 1.000000000000000000, 0.8660254037844387076, 1.000000000000000000, 0.8660254037844387076, 1.000000000000000000, 0.8660254037844387076, 1.000000000000000000, 0.8660254037844387076, 1.000000000000000000, 0.8660254037844387076, 1.000000000000000000, 0.8660254037844387076, 1.000000000000000000, 0.8660254037844387076, 1.000000000000000000, 0.8660254037844387076, 1.000000000000000000, 0.8660254037844387076, 1.000000000000000000, 0.8660254037844387076, 1.000000000000000000, 0.8660254037844387076, 1.000000000000000000, 0.8660254037844387076, 1.000000000000000000, 0.9111409417988175496, 0.9401539645359766606) ) ) 
 REPRESENTATION_ITEM ( '' )  SURFACE ( )  );
#18886=PLANE ( 'NONE',  #14897 ) ;
#18889=FACE_OUTER_BOUND ( 'NONE', #17691, .T. ) ;
#18896=ORIENTED_EDGE ( 'NONE', *, *, #10788, .T. ) ;
#18899=CARTESIAN_POINT ( 'NONE',  ( 85.15643035624999868, -34.15312499938548285, 98.40857419181659793 ) ) ;
#18903=CARTESIAN_POINT ( 'NONE',  ( -85.15643035625001289, -33.89062499938548711, -101.5914258081833879 ) ) ;
#18904=CARTESIAN_POINT ( 'NONE',  ( 81.02178482187500208, -32.99062499938548854, 102.3871387122750889 ) ) ;
#18905=EDGE_CURVE ( 'NONE', #16451, #16118, #18931, .T. ) ;
#18907=CARTESIAN_POINT ( 'NONE',  ( 79.64356964375001269, -33.66562499938549280, -101.5914258081833879 ) ) ;
#18909=CARTESIAN_POINT ( 'NONE',  ( -83.77821517812500929, -34.11562499938548854, 102.3871387122750889 ) ) ;
#18910=CARTESIAN_POINT ( 'NONE',  ( 82.39999999999999147, -31.82812499938548356, -103.1828516163667899 ) ) ;
#18912=CARTESIAN_POINT ( 'NONE',  ( 85.15643035624999868, -34.34062499938548285, 101.5914258081833879 ) ) ;
#18916=CARTESIAN_POINT ( 'NONE',  ( -83.77821517812500929, -32.76562499938548711, 102.3871387122750889 ) ) ;
#18917=CARTESIAN_POINT ( 'NONE',  ( -83.77821517812500929, -31.41562499938548569, 102.3871387122750889 ) ) ;
#18918=CARTESIAN_POINT ( 'NONE',  ( 83.90000000000000568, -34.87500000000000000, 97.40192378864668399 ) ) ;
#18920=ADVANCED_FACE ( 'NONE', ( #14509 ), #11209, .T. ) ;
#18923=CARTESIAN_POINT ( 'NONE',  ( 82.40000000000000568, -33.71249999999998437, -96.99999999999998579 ) ) ;
#18925=CARTESIAN_POINT ( 'NONE',  ( -85.40000000000000568, -34.85624999877096997, 101.7320508075688821 ) ) ;
#18926=CARTESIAN_POINT ( 'NONE',  ( -80.90000000000000568, -33.24374999877097281, -102.5980762113533018 ) ) ;
#18928=DIRECTION ( 'NONE',  ( -0.000000000000000000, 0.000000000000000000, -1.000000000000000000 ) ) ;
#18931=LINE ( 'NONE', #18838, #4648 ) ;
#18932=CARTESIAN_POINT ( 'NONE',  ( 85.15643035624999868, -33.89062499938548711, -98.40857419181659793 ) ) ;
#18934=ORIENTED_EDGE ( 'NONE', *, *, #6579, .T. ) ;
#18935=CARTESIAN_POINT ( 'NONE',  ( 80.90000000000000568, -32.49374999877097281, 97.40192378864668399 ) ) ;
#18939=FACE_OUTER_BOUND ( 'NONE', #1867, .T. ) ;
#18942=CARTESIAN_POINT ( 'NONE',  ( -82.39999999999999147, -33.40312499938548285, -103.1828516163667899 ) ) ;
#18946=CARTESIAN_POINT ( 'NONE',  ( 85.15643035625001289, -33.89062499938548711, 101.5914258081833879 ) ) ;
#18947=CARTESIAN_POINT ( 'NONE',  ( -83.77821517812500929, -31.22812499938548569, -102.3871387122750889 ) ) ;
#18948=CARTESIAN_POINT ( 'NONE',  ( 80.90000000000000568, -34.64999999999999858, 102.5980762113533018 ) ) ;
#18949=CARTESIAN_POINT ( 'NONE',  ( 81.59615242270662350, -34.76115380933863719, -103.0000000000000000 ) ) ;
#18953=CARTESIAN_POINT ( 'NONE',  ( -85.15643035625001289, -32.87812499938548427, -101.5914258081833879 ) ) ;
#18955=CARTESIAN_POINT ( 'NONE',  ( 79.39999999999999147, -32.41874999877096997, -99.99999999999998579 ) ) ;
#18961=EDGE_CURVE ( 'NONE', #3695, #11655, #5648, .T. ) ;
#18971=CARTESIAN_POINT ( 'NONE',  ( 85.40000000000000568, -31.76249999999999929, -101.7320508075688679 ) ) ;
#18972=CARTESIAN_POINT ( 'NONE',  ( 81.01744233620649993, -31.99999999999999289, -102.5835086888312162 ) ) ;
#18973=AXIS2_PLACEMENT_3D ( 'NONE', #17995, #9184, #9087 ) ;
#18975=CARTESIAN_POINT ( 'NONE',  ( -79.64356964374999848, -32.72812499938548569, 99.99999999999998579 ) ) ;
#18980=CARTESIAN_POINT ( 'NONE',  ( 81.05805657947855991, -35.00000000000000711, 102.6149389257479640 ) ) ;
#18981=CARTESIAN_POINT ( 'NONE',  ( 84.25709831968876529, -34.99999999999999289, 97.88253972981353002 ) ) ;
#18982=CARTESIAN_POINT ( 'NONE',  ( 85.15643035624999868, -35.05312499938548143, -101.5914258081833879 ) ) ;
#18983=ORIENTED_EDGE ( 'NONE', *, *, #4026, .T. ) ;
#18985=CARTESIAN_POINT ( 'NONE',  ( -81.02178482187500208, -31.19062499938548427, -102.3871387122750889 ) ) ;
#18994=EDGE_LOOP ( 'NONE', ( #1851, #18480, #6123, #11511 ) ) ;
#18996=CARTESIAN_POINT ( 'NONE',  ( 83.25523545990762386, -35.19352049914630953, 103.2690260512239604 ) ) ;
#18997=CARTESIAN_POINT ( 'NONE',  ( -82.40000000000000568, -33.71249999999998437, 96.99999999999998579 ) ) ;
#19000=CYLINDRICAL_SURFACE ( 'NONE', #12963, 3.000000000000002665 ) ;
#19002=CARTESIAN_POINT ( 'NONE',  ( -81.02178482187500208, -33.70312499938548711, -97.61286128772489690 ) ) ;
#19004=CARTESIAN_POINT ( 'NONE',  ( 81.02178482187500208, -33.10312499938548569, -97.61286128772489690 ) ) ;
#19006=CARTESIAN_POINT ( 'NONE',  ( -85.15643035625001289, -34.15312499938548285, 101.5914258081833879 ) ) ;
#19007=CARTESIAN_POINT ( 'NONE',  ( 79.64356964375001269, -30.40312499938548285, -101.5914258081833879 ) ) ;
#19008=EDGE_LOOP ( 'NONE', ( #8873, #686, #3716, #18370 ) ) ;
#19009=CARTESIAN_POINT ( 'NONE',  ( 81.02178482187500208, -34.45312499938548711, 102.3871387122750889 ) ) ;
#19012=CARTESIAN_POINT ( 'NONE',  ( -79.64356964374999848, -34.41562499938548569, 99.99999999999998579 ) ) ;
#19013=CARTESIAN_POINT ( 'NONE',  ( -83.77821517812500929, -30.51562499938548711, 102.3871387122750889 ) ) ;
#19014=VERTEX_POINT ( 'NONE', #5460 ) ;
#19018=CARTESIAN_POINT ( 'NONE',  ( -83.90000000000000568, -34.42500000000000426, 102.5980762113533018 ) ) ;
#19020=CARTESIAN_POINT ( 'NONE',  ( -79.39999999999999147, -33.35624999877096997, -98.26794919243113213 ) ) ;
#19021=CARTESIAN_POINT ( 'NONE',  ( 84.93334430221547393, -32.00000000000000000, 98.89901723338974193 ) ) ;
#19022=CARTESIAN_POINT ( 'NONE',  ( 79.64356964375001269, -32.24062499938548854, 101.5914258081833879 ) ) ;
#19025=CARTESIAN_POINT ( 'NONE',  ( 85.15643035625001289, -33.85312499938549280, -99.99999999999998579 ) ) ;
#19026=CARTESIAN_POINT ( 'NONE',  ( 79.39999999999999147, -32.86874999877097281, 99.99999999999998579 ) ) ;
#19027=ORIENTED_EDGE ( 'NONE', *, *, #2123, .T. ) ;
#19028=CARTESIAN_POINT ( 'NONE',  ( 82.39999999999999147, -32.75624999877096855, 103.4641016151377499 ) ) ;
#19031=CARTESIAN_POINT ( 'NONE',  ( 82.40000000000000568, -34.38749999999999574, 96.99999999999998579 ) ) ;
#19033=VERTEX_POINT ( 'NONE', #9744 ) ;
#19034=CARTESIAN_POINT ( 'NONE',  ( -82.39999999999999147, -34.30312499938548143, -103.1828516163667899 ) ) ;
#19035=CARTESIAN_POINT ( 'NONE',  ( 85.40000000000000568, -33.14999999999999858, 99.99999999999998579 ) ) ;
#19038=CARTESIAN_POINT ( 'NONE',  ( 82.39999999999999147, -34.86562499938548854, 103.1828516163667899 ) ) ;
#19039=CARTESIAN_POINT ( 'NONE',  ( -79.39999999999999147, -35.08124999877097139, -101.7320508075688821 ) ) ;
#19040=CARTESIAN_POINT ( 'NONE',  ( -83.90000000000000568, -32.11874999877097281, -97.40192378864668399 ) ) ;
#19041=LINE ( 'NONE', #1068, #15692 ) ;
#19044=CARTESIAN_POINT ( 'NONE',  ( -79.64356964374998427, -33.02812499938548285, -101.5914258081833879 ) ) ;
#19047=EDGE_CURVE ( 'NONE', #15577, #14, #17364, .T. ) ;
#19048=CARTESIAN_POINT ( 'NONE',  ( 80.90000000000000568, -32.49374999877097281, -102.5980762113533018 ) ) ;
#19050=EDGE_CURVE ( 'NONE', #13807, #13667, #13060, .T. ) ;
#19052=CARTESIAN_POINT ( 'NONE',  ( 81.02178482187500208, -34.34062499938548285, -97.61286128772489690 ) ) ;
#19056=EDGE_CURVE ( 'NONE', #6865, #11363, #7141, .T. ) ;
#19061=CARTESIAN_POINT ( 'NONE',  ( 81.59615242270662350, -34.36740381056766580, -102.9999999999999858 ) ) ;
#19064=B_SPLINE_CURVE_WITH_KNOTS ( 'NONE', 3,
 ( #8606, #10277, #14659, #17700, #17603, #18980, #4409, #2641, #8509, #4216, #8707, #2547, #4316, #7436, #16239, #1195, #8802, #17418 ),
 .UNSPECIFIED., .F., .F.,
 ( 4, 2, 2, 2, 2, 2, 2, 2, 4 ),
 ( 0.000000000000000000, 0.0007106627595359126057, 0.001421325519071825211, 0.002131988278607738034, 0.002842651038143650423, 0.003553313797679562812, 0.004263976557215476068, 0.004974639316751388457, 0.005685302076287300846 ),
 .UNSPECIFIED. ) ;
#19066=CARTESIAN_POINT ( 'NONE',  ( 80.90000000000000568, -31.65000000000000568, -102.5980762113533018 ) ) ;
#19067=CARTESIAN_POINT ( 'NONE',  ( 94.79999999999995453, -35.00000000000000000, 150.0000000000000000 ) ) ;
#19068=CARTESIAN_POINT ( 'NONE',  ( -81.02178482187500208, -31.75312499938548427, 97.61286128772489690 ) ) ;
#19070=EDGE_CURVE ( 'NONE', #17663, #11212, #19106, .T. ) ;
#19074=CARTESIAN_POINT ( 'NONE',  ( -85.40000000000000568, -34.53750000000000142, -101.7320508075688821 ) ) ;
#19075=ORIENTED_EDGE ( 'NONE', *, *, #892, .T. ) ;
#19076=CARTESIAN_POINT ( 'NONE',  ( -81.02178482187500208, -31.64062499938548356, -102.3871387122750889 ) ) ;
#19078=FACE_OUTER_BOUND ( 'NONE', #661, .T. ) ;
#19081=CARTESIAN_POINT ( 'NONE',  ( 82.39999999999999147, -32.58749999999999858, 96.99999999999998579 ) ) ;
#19085=EDGE_LOOP ( 'NONE', ( #19281, #12178, #3811, #427 ) ) ;
#19088=CARTESIAN_POINT ( 'NONE',  ( 79.64356964375001269, -34.90312499938548285, 98.40857419181659793 ) ) ;
#19092=CARTESIAN_POINT ( 'NONE',  ( -79.39999999999999147, -33.86250000000000426, 101.7320508075688537 ) ) ;
#19093=CARTESIAN_POINT ( 'NONE',  ( 85.40000000000000568, -33.05624999877097281, -101.7320508075688821 ) ) ;
#19094=CARTESIAN_POINT ( 'NONE',  ( 79.64356964375001269, -31.67812499938548143, -98.40857419181659793 ) ) ;
#19096=CARTESIAN_POINT ( 'NONE',  ( -83.77821517812500929, -32.76562499938548711, 102.3871387122750889 ) ) ;
#19097=CARTESIAN_POINT ( 'NONE',  ( 83.77821517812500929, -30.66562499938548569, -97.61286128772489690 ) ) ;
#19102=CARTESIAN_POINT ( 'NONE',  ( -81.02178482187500208, -32.69062499938548427, 102.3871387122750889 ) ) ;
#19106=( BOUNDED_CURVE ( )  B_SPLINE_CURVE ( 2, ( #6025, #11973, #17653, #14704, #10607, #2892, #15006, #1341, #8848 ),
 .UNSPECIFIED., .F., .F. ) 
 B_SPLINE_CURVE_WITH_KNOTS ( ( 3, 2, 2, 2, 3 ),
 ( 0.4375000000000000555, 0.4444444444444444198, 0.4583333333333333148, 0.4722222222222222099, 0.4791666666666666297 ),
 .UNSPECIFIED. ) 
 CURVE ( )  GEOMETRIC_REPRESENTATION_ITEM ( )  RATIONAL_B_SPLINE_CURVE ( ( 0.9330127018922192983, 0.9330127018922198534, 1.000000000000000000, 0.8660254037844387076, 1.000000000000000000, 0.8660254037844387076, 1.000000000000000000, 0.9330127018922196314, 0.9330127018922194093 ) ) 
 REPRESENTATION_ITEM ( '' )  );
#19109=CARTESIAN_POINT ( 'NONE',  ( 81.70916641599872321, -34.99999999999998579, -97.11314983874012796 ) ) ;
#19111=CARTESIAN_POINT ( 'NONE',  ( -83.90000000000000568, -34.57500000000000284, 97.40192378864668399 ) ) ;
#19114=CARTESIAN_POINT ( 'NONE',  ( -79.39999999999999147, -32.45624999877097139, -98.26794919243113213 ) ) ;
#19115=CARTESIAN_POINT ( 'NONE',  ( 79.64356964375001269, -31.41562499938548569, 98.40857419181659793 ) ) ;
#19116=LINE ( 'NONE', #14611, #3966 ) ;
#19117=DIRECTION ( 'NONE',  ( 0.000000000000000000, -0.000000000000000000, 1.000000000000000000 ) ) ;
#19118=CARTESIAN_POINT ( 'NONE',  ( 85.15643035624999868, -32.91562499938549280, -101.5914258081833879 ) ) ;
#19119=CARTESIAN_POINT ( 'NONE',  ( -83.77821517812500929, -31.67812499938548498, -102.3871387122750889 ) ) ;
#19120=AXIS2_PLACEMENT_3D ( 'NONE', #1209, #10003, #17433 ) ;
#19122=CARTESIAN_POINT ( 'NONE',  ( 83.90000000000000568, -33.46874999877096712, 97.40192378864668399 ) ) ;
#19124=DIRECTION ( 'NONE',  ( 0.000000000000000000, 0.000000000000000000, 1.000000000000000000 ) ) ;
#19126=CARTESIAN_POINT ( 'NONE',  ( 79.39999999999999147, -33.80624999877097281, -101.7320508075688537 ) ) ;
#19128=CARTESIAN_POINT ( 'NONE',  ( -81.02178482187500208, -34.94062499938548427, -97.61286128772489690 ) ) ;
#19132=CARTESIAN_POINT ( 'NONE',  ( -84.69813954184694182, -35.39427337414329600, -101.9283554252781272 ) ) ;
#19134=CARTESIAN_POINT ( 'NONE',  ( -83.92761994968563499, -32.00000000000000000, -102.3311504458614394 ) ) ;
#19135=CARTESIAN_POINT ( 'NONE',  ( -79.39999999999999147, -31.48124999877097352, -101.7320508075688821 ) ) ;
#19139=CARTESIAN_POINT ( 'NONE',  ( -79.64356964374999848, -32.16562499938548569, -99.99999999999998579 ) ) ;
#19140=ADVANCED_FACE ( 'NONE', ( #14907 ), #5930, .T. ) ;
#19142=FACE_OUTER_BOUND ( 'NONE', #3880, .T. ) ;
#19143=CARTESIAN_POINT ( 'NONE',  ( 79.39999999999999147, -32.45624999877097139, -101.7320508075688537 ) ) ;
#19148=CARTESIAN_POINT ( 'NONE',  ( 85.15643035625001289, -34.64062499938548711, -99.99999999999998579 ) ) ;
#19156=CARTESIAN_POINT ( 'NONE',  ( -82.39999999999999147, -32.98124999877096286, 102.9999999999999858 ) ) ;
#19163=CARTESIAN_POINT ( 'NONE',  ( -81.02178482187500208, -34.90312499938548285, 97.61286128772489690 ) ) ;
#19166=CARTESIAN_POINT ( 'NONE',  ( -81.59615242270662350, -34.63259618943234130, -103.0000000000000000 ) ) ;
#19170=CARTESIAN_POINT ( 'NONE',  ( 83.65502553130815500, -34.99999999999999289, 97.51146709331014506 ) ) ;
#19172=ORIENTED_EDGE ( 'NONE', *, *, #12234, .T. ) ;
#19173=CARTESIAN_POINT ( 'NONE',  ( -81.02178482187500208, -30.89062499938548711, -97.61286128772489690 ) ) ;
#19178=CARTESIAN_POINT ( 'NONE',  ( 82.40000000000001990, -33.26250000000000284, 103.0000000000000000 ) ) ;
#19181=VERTEX_POINT ( 'NONE', #10226 ) ;
#19182=FACE_BOUND ( 'NONE', #13379, .T. ) ;
#19185=CARTESIAN_POINT ( 'NONE',  ( 79.39999999999999147, -30.26249999999999929, 98.26794919243113213 ) ) ;
#19186=CARTESIAN_POINT ( 'NONE',  ( 83.20384757729335945, -34.14240381056767148, -96.99999999999998579 ) ) ;
#19192=CARTESIAN_POINT ( 'NONE',  ( 81.02178482187500208, -34.49062499938548854, 97.61286128772489690 ) ) ;
#19193=CARTESIAN_POINT ( 'NONE',  ( 85.15643035624999868, -31.00312499938548072, -101.5914258081833879 ) ) ;
#19195=CARTESIAN_POINT ( 'NONE',  ( -81.02178482187500208, -34.94062499938548427, 102.3871387122750889 ) ) ;
#19196=FACE_OUTER_BOUND ( 'NONE', #7949, .T. ) ;
#19197=ORIENTED_EDGE ( 'NONE', *, *, #8958, .F. ) ;
#19199=CARTESIAN_POINT ( 'NONE',  ( 85.15643035624999868, -35.16562499938547859, 98.40857419181659793 ) ) ;
#19203=CARTESIAN_POINT ( 'NONE',  ( -83.77821517812500929, -33.66562499938548569, 102.3871387122750889 ) ) ;
#19204=ORIENTED_EDGE ( 'NONE', *, *, #10846, .T. ) ;
#19208=CARTESIAN_POINT ( 'NONE',  ( 80.32125193361331128, -35.00000000000000000, -97.97655282300733859 ) ) ;
#19213=CARTESIAN_POINT ( 'NONE',  ( 85.15643035625001289, -32.50312499938548427, 99.99999999999998579 ) ) ;
#19214=CARTESIAN_POINT ( 'NONE',  ( -83.20384757729337366, -32.79240381056766296, 97.00000000000000000 ) ) ;
#19216=CARTESIAN_POINT ( 'NONE',  ( 83.77821517812500929, -34.37812499938548427, -97.61286128772489690 ) ) ;
#19217=CARTESIAN_POINT ( 'NONE',  ( -81.02178482187500208, -30.85312499938548569, -102.3871387122750889 ) ) ;
#19219=CARTESIAN_POINT ( 'NONE',  ( 79.39999999999999147, -33.31874999877096855, 99.99999999999998579 ) ) ;
#19221=CARTESIAN_POINT ( 'NONE',  ( 85.40000000000000568, -32.68124999877097281, 101.7320508075688821 ) ) ;
#19224=CARTESIAN_POINT ( 'NONE',  ( -96.99999999999998579, -29.80000000000000426, -150.0000000000000000 ) ) ;
#19225=CARTESIAN_POINT ( 'NONE',  ( 80.60346964444597972, -31.99999999999999289, 102.3251727584800648 ) ) ;
#19227=CARTESIAN_POINT ( 'NONE',  ( -83.77821517812500929, -33.66562499938548569, -97.61286128772489690 ) ) ;
#19230=EDGE_LOOP ( 'NONE', ( #19300, #11042, #7781, #4610 ) ) ;
#19232=CARTESIAN_POINT ( 'NONE',  ( -79.64356964375001269, -34.56562499938549138, -98.40857419181659793 ) ) ;
#19233=CARTESIAN_POINT ( 'NONE',  ( -81.44903907891985284, -32.00000000000000711, -102.7404298451142353 ) ) ;
#19234=CARTESIAN_POINT ( 'NONE',  ( -80.90000000000000568, -31.44374999877096855, -102.5980762113533018 ) ) ;
#19238=CARTESIAN_POINT ( 'NONE',  ( -82.39999999999999147, -34.52812499938548285, -96.81714838363319586 ) ) ;
#19239=DIRECTION ( 'NONE',  ( -0.000000000000000000, -1.000000000000000000, -0.000000000000000000 ) ) ;
#19241=CARTESIAN_POINT ( 'NONE',  ( 79.39999999999999147, -31.03124999877097068, -98.26794919243110371 ) ) ;
#19252=CARTESIAN_POINT ( 'NONE',  ( -83.30522522564109522, -32.00000000000000000, 97.33297554273082142 ) ) ;
#19257=CARTESIAN_POINT ( 'NONE',  ( 85.40000000000000568, -34.08749999999999858, -98.26794919243111792 ) ) ;
#19260=CARTESIAN_POINT ( 'NONE',  ( -82.39999999999999147, -33.96562499938548285, 96.81714838363319586 ) ) ;
#19266=CARTESIAN_POINT ( 'NONE',  ( -81.59615242270662350, -34.76115380933863719, -96.99999999999995737 ) ) ;
#19268=ORIENTED_EDGE ( 'NONE', *, *, #18961, .T. ) ;
#19269=AXIS2_PLACEMENT_3D ( 'NONE', #17008, #12510, #3525 ) ;
#19270=DIRECTION ( 'NONE',  ( 0.000000000000000000, 0.000000000000000000, 1.000000000000000000 ) ) ;
#19271=CARTESIAN_POINT ( 'NONE',  ( -79.64356964374999848, -30.36562499938548498, -99.99999999999998579 ) ) ;
#19273=EDGE_CURVE ( 'NONE', #609, #422, #18483, .T. ) ;
#19275=( BOUNDED_CURVE ( )  B_SPLINE_CURVE ( 2, ( #5289, #15542, #8114, #5094, #12602, #18673, #3903, #3614, #12893, #13709, #3804, #11236, #12247, #796, #18214, #18574, #14162, #9773, #17394, #6853, #11039, #2341, #17199, #9869, #8303, #12798, #9207, #3712, #18765, #8399, #17003, #11333, #14067, #15639, #7754, #14351, #2443, #9575, #702, #11133, #5387, #6754, #17298, #6657, #2245, #14256, #5187, #9678, #11432, #17101, #8213, #12699, #15832, #987, #6943, #18864, #5486, #15172, #5762, #7221, #13176, #7131, #10157, #14736, #19052, #17584, #7413, #2827, #16119, #1273, #5957, #11906, #19148, #7317, #8488, #12989, #4195, #14834, #1459, #13375, #1371, #13271, #2728 ),
 .UNSPECIFIED., .F., .F. ) 
 B_SPLINE_CURVE_WITH_KNOTS ( ( 3, 2, 2, 2, 2, 2, 2, 2, 2, 2, 2, 2, 2, 2, 2, 2, 2, 2, 2, 2, 2, 2, 2, 2, 2, 2, 2, 2, 2, 2, 2, 2, 2, 2, 2, 2, 2, 2, 2, 2, 2, 3 ),
 ( 0.3716916592825992294, 0.3750191855951752751, 0.3900199530189822905, 0.4050207204427893060, 0.4200214878665963214, 0.4350222552904033368, 0.4500230227142103523, 0.4650237901380173677, 0.4800245575618243277, 0.4950253249856313431, 0.5100260924094383030, 0.5250268598332453740, 0.5400276272570523339, 0.5550283946808594049, 0.5700291621046664758, 0.5850299295284733248, 0.6000306969522805067, 0.6150314643760874667, 0.6300322317998945376, 0.6450329992237013865, 0.6600337666475084575, 0.6750345340713155284, 0.6900353014951223773, 0.7050360689189295593, 0.7200368363427365193, 0.7350376037665435902, 0.7500383711903504391, 0.7650391386141575101, 0.7800399060379645810, 0.7950406734617716520, 0.8100414408855785009, 0.8250422083093855719, 0.8400429757331926428, 0.8550437431569994917, 0.8700445105808066737, 0.8850452780046136336, 0.9000460454284207046, 0.9150468128522275535, 0.9300475802760348465, 0.9450483476998416954, 0.9600491151236487664, 0.9717223562348820121 ),
 .UNSPECIFIED. ) 
 CURVE ( )  GEOMETRIC_REPRESENTATION_ITEM ( )  RATIONAL_B_SPLINE_CURVE ( ( 0.9537471549766813883, 0.9702812541832683824, 1.000000000000000000, 0.8660254037844387076, 1.000000000000000000, 0.8660254037844387076, 1.000000000000000000, 0.8660254037844387076, 1.000000000000000000, 0.8660254037844387076, 1.000000000000000000, 0.8660254037844387076, 1.000000000000000000, 0.8660254037844387076, 1.000000000000000000, 0.8660254037844387076, 1.000000000000000000, 0.8660254037844387076, 1.000000000000000000, 0.8660254037844387076, 1.000000000000000000, 0.8660254037844387076, 1.000000000000000000, 0.8660254037844387076, 1.000000000000000000, 0.8660254037844387076, 1.000000000000000000, 0.8660254037844387076, 1.000000000000000000, 0.8660254037844387076, 1.000000000000000000, 0.8660254037844387076, 1.000000000000000000, 0.8660254037844387076, 1.000000000000000000, 0.8660254037844387076, 1.000000000000000000, 0.8660254037844387076, 1.000000000000000000, 0.8660254037844387076, 1.000000000000000000, 0.8660254037844387076, 1.000000000000000000, 0.8660254037844387076, 1.000000000000000000, 0.8660254037844387076, 1.000000000000000000, 0.8660254037844387076, 1.000000000000000000, 0.8660254037844387076, 1.000000000000000000, 0.8660254037844387076, 1.000000000000000000, 0.8660254037844387076, 1.000000000000000000, 0.8660254037844387076, 1.000000000000000000, 0.8660254037844387076, 1.000000000000000000, 0.8660254037844387076, 1.000000000000000000, 0.8660254037844387076, 1.000000000000000000, 0.8660254037844387076, 1.000000000000000000, 0.8660254037844387076, 1.000000000000000000, 0.8660254037844387076, 1.000000000000000000, 0.8660254037844387076, 1.000000000000000000, 0.8660254037844387076, 1.000000000000000000, 0.8660254037844387076, 1.000000000000000000, 0.8660254037844387076, 1.000000000000000000, 0.8660254037844387076, 1.000000000000000000, 0.8660254037844387076, 1.000000000000000000, 0.8957441496011493420, 0.9537471549767048140 ) ) 
 REPRESENTATION_ITEM ( '' )  );
#19277=CARTESIAN_POINT ( 'NONE',  ( 79.39999999999999147, -33.41250000000000142, 98.26794919243113213 ) ) ;
#19281=ORIENTED_EDGE ( 'NONE', *, *, #64, .F. ) ;
#19283=DIRECTION ( 'NONE',  ( -1.000000000000000000, 0.000000000000000000, 0.000000000000000000 ) ) ;
#19286=CARTESIAN_POINT ( 'NONE',  ( -83.90000000000000568, -31.36874999877096926, 97.40192378864668399 ) ) ;
#19287=CARTESIAN_POINT ( 'NONE',  ( 82.39999999999999147, -34.97812499938547859, 96.81714838363319586 ) ) ;
#19289=FACE_OUTER_BOUND ( 'NONE', #9747, .T. ) ;
#19293=CARTESIAN_POINT ( 'NONE',  ( 81.02178482187500208, -34.94062499938548427, 97.61286128772489690 ) ) ;
#19295=CARTESIAN_POINT ( 'NONE',  ( 81.02178482187500208, -31.19062499938548427, -97.61286128772489690 ) ) ;
#19297=CARTESIAN_POINT ( 'NONE',  ( -82.05869624310423660, -34.96883842999723413, 102.9857998004475803 ) ) ;
#19298=CARTESIAN_POINT ( 'NONE',  ( 85.15643035624999868, -32.35312499938549280, -101.5914258081833879 ) ) ;
#19300=ORIENTED_EDGE ( 'NONE', *, *, #17160, .F. ) ;
#19301=FACE_OUTER_BOUND ( 'NONE', #18863, .T. ) ;
#19304=CARTESIAN_POINT ( 'NONE',  ( -83.90000000000000568, -31.27500000000000568, 102.5980762113533018 ) ) ;
#19306=LINE ( 'NONE', #17832, #591 ) ;
#19307=VECTOR ( 'NONE', #12337, 1000.000000000000000 ) ;
#19310=CARTESIAN_POINT ( 'NONE',  ( 82.39999999999999147, -32.58750000000000568, -102.9999999999999858 ) ) ;
#19317=CARTESIAN_POINT ( 'NONE',  ( 83.77821517812500929, -31.52812499938548996, 97.61286128772489690 ) ) ;
#19318=CARTESIAN_POINT ( 'NONE',  ( -82.39999999999999147, -32.81250000000000000, 97.00000000000000000 ) ) ;
#19320=CARTESIAN_POINT ( 'NONE',  ( -79.64356964374998427, -32.76562499938548711, 101.5914258081833879 ) ) ;
#19344=COLOUR_RGB('Light Blue',0.38,0.62,0.78);
#19345=FILL_AREA_STYLE_COLOUR('',#19344);
#19346=FILL_AREA_STYLE('',(#19345));
#19347=SURFACE_STYLE_FILL_AREA(#19346);
#19348=SURFACE_SIDE_STYLE('',(#19347));
#19349=SURFACE_STYLE_USAGE(.BOTH.,#19348);
#19350=PRESENTATION_STYLE_ASSIGNMENT((#19349));
ENDSEC;
END-ISO-10303-21;
